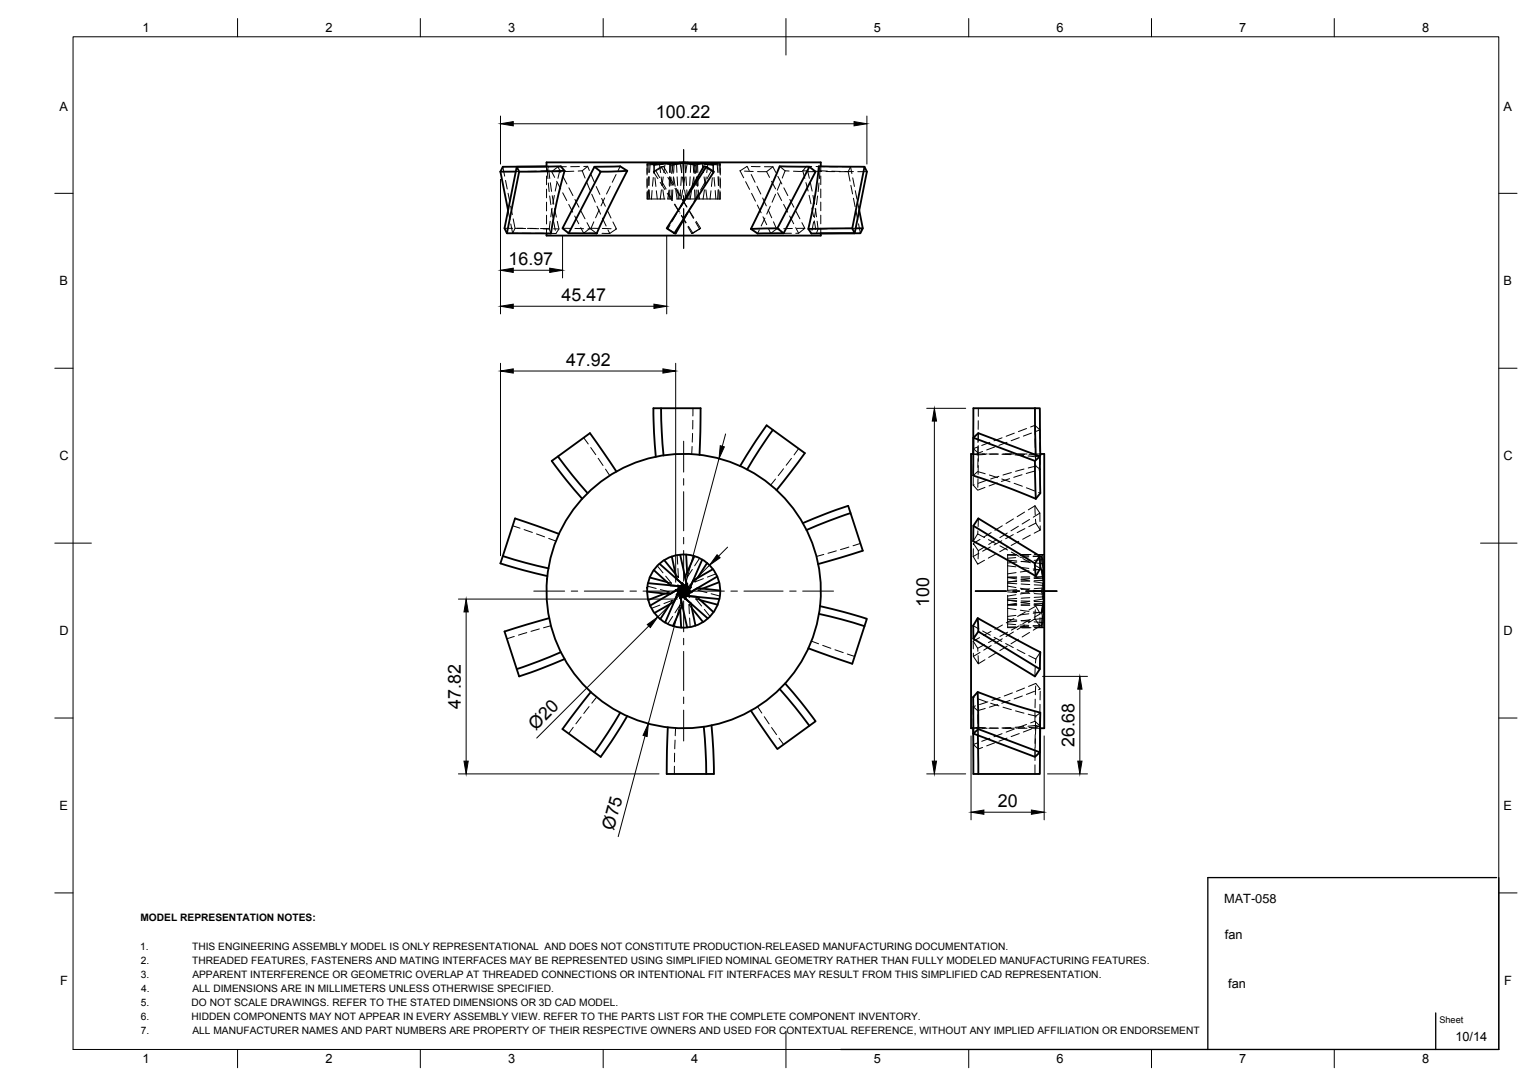
ISO-10303-21;
HEADER;
FILE_DESCRIPTION (('STEP AP214'),
    '1' );
FILE_NAME ('fan.step',
    '2026-10-21T17:54:40',
    ( '' ),
    ( '' ),
    'SwSTEP 2.0',
    'SolidWorks 2026',
    '' );
FILE_SCHEMA (( 'AUTOMOTIVE_DESIGN' ));
ENDSEC;

DATA;
#1=CARTESIAN_POINT ( 'NONE',  ( -0.3862712429686977478, 1.188820645368937390, -10.00000000000000000 ) ) ;
#18=CARTESIAN_POINT ( 'NONE',  ( -1.011271242968683426, -0.7347315653655928092, 3.333333333333333481 ) ) ;
#19=CARTESIAN_POINT ( 'NONE',  ( 42.78107912161490844, -16.56908454419397003, -9.367992836599951190 ) ) ;
#23=B_SPLINE_CURVE_WITH_KNOTS ( 'NONE', 3,
 ( #8249, #22875, #15684, #35464 ),
 .UNSPECIFIED., .F., .F.,
 ( 4, 4 ),
 ( 0.9895749839358303213, 1.000000000000000000 ),
 .UNSPECIFIED. ) ;
#32=CARTESIAN_POINT ( 'NONE',  ( -24.39427009666018265, -44.07992421011638129, 8.807470649214879543 ) ) ;
#37=CARTESIAN_POINT ( 'NONE',  ( 38.06347959788622859, -17.13191708601470964, -8.080361901872240793 ) ) ;
#38=FACE_OUTER_BOUND ( 'NONE', #34200, .T. ) ;
#42=EDGE_LOOP ( 'NONE', ( #31144, #13391, #8793, #47116, #38295 ) ) ;
#43=FACE_OUTER_BOUND ( 'NONE', #38714, .T. ) ;
#44=CARTESIAN_POINT ( 'NONE',  ( 45.64490844644691236, 21.32281559348795952, 8.807470649214879543 ) ) ;
#48=ORIENTED_EDGE ( 'NONE', *, *, #42434, .T. ) ;
#56=CARTESIAN_POINT ( 'NONE',  ( 47.23269937569327226, -16.43609759007049931, -2.408242355805840784 ) ) ;
#65=CARTESIAN_POINT ( 'NONE',  ( -0.3370904143228978245, 0.2449105217885259589, 10.00000000000000000 ) ) ;
#67=CARTESIAN_POINT ( 'NONE',  ( -12.78770032058971395, -31.68259716188267916, 7.455576670931136185 ) ) ;
#71=CARTESIAN_POINT ( 'NONE',  ( 10.30302290646030450, 13.08520913973580235, -9.683996418299976483 ) ) ;
#74=CARTESIAN_POINT ( 'NONE',  ( 50.11058929355269953, -7.578863168071589662, 7.455576670931136185 ) ) ;
#76=VERTEX_POINT ( 'NONE', #17762 ) ;
#84=CARTESIAN_POINT ( 'NONE',  ( -0.8965959638259611841, -1.582931917743307215, 9.903764339332084887 ) ) ;
#89=ORIENTED_EDGE ( 'NONE', *, *, #20681, .F. ) ;
#93=CARTESIAN_POINT ( 'NONE',  ( -32.43949840348904701, -7.871562655726274116, -9.367992836599954742 ) ) ;
#102=CARTESIAN_POINT ( 'NONE',  ( 1.011271242968688311, -0.7347315653655855927, 10.00000000000000000 ) ) ;
#108=ADVANCED_FACE ( 'NONE', ( #42862 ), #18238, .T. ) ;
#109=B_SPLINE_CURVE_WITH_KNOTS ( 'NONE', 3,
 ( #13337, #1308, #25156, #24903 ),
 .UNSPECIFIED., .F., .F.,
 ( 4, 4 ),
 ( 1.110764993427085326E-17, 0.002466147708923237519 ),
 .UNSPECIFIED. ) ;
#115=CARTESIAN_POINT ( 'NONE',  ( 24.39427009665985224, 44.07992421011656603, 8.807470649214879543 ) ) ;
#130=EDGE_CURVE ( 'NONE', #39856, #25517, #44158, .T. ) ;
#132=CIRCLE ( 'NONE', #9133, 37.50000000000000000 ) ;
#138=ADVANCED_FACE ( 'NONE', ( #43 ), #14562, .T. ) ;
#142=CARTESIAN_POINT ( 'NONE',  ( 1.088201875076330705, 0.7239277119154168272, 9.945465949847356768 ) ) ;
#146=ORIENTED_EDGE ( 'NONE', *, *, #12335, .F. ) ;
#148=CARTESIAN_POINT ( 'NONE',  ( 35.51846793572394034, -35.99772139009119343, 7.906207997025717304 ) ) ;
#149=CARTESIAN_POINT ( 'NONE',  ( -4.763548243873389154, 16.57409059453848599, 8.727788335465566760 ) ) ;
#154=CARTESIAN_POINT ( 'NONE',  ( 2.188678504086826848, -0.3267089737525829540, 9.881002359080282460 ) ) ;
#157=CARTESIAN_POINT ( 'NONE',  ( 1.249999999999999778, 0.000000000000000000, 3.333333333333333481 ) ) ;
#158=CARTESIAN_POINT ( 'NONE',  ( 1.228394325311184421, -1.341866297401743235, 9.903764339332088440 ) ) ;
#165=LINE ( 'NONE', #47317, #28159 ) ;
#170=CARTESIAN_POINT ( 'NONE',  ( -0.3862712429686977478, 1.188820645368937390, -3.333333333333333481 ) ) ;
#178=CARTESIAN_POINT ( 'NONE',  ( 26.18032376592674737, -21.95228666728361233, 7.455576670931136185 ) ) ;
#188=CARTESIAN_POINT ( 'NONE',  ( -49.46074318306826001, 9.578883844007169301, 8.807470649214879543 ) ) ;
#197=ORIENTED_EDGE ( 'NONE', *, *, #48845, .F. ) ;
#213=CARTESIAN_POINT ( 'NONE',  ( -0.4830800013901715428, -1.200413232422907761, 9.947020512645419643 ) ) ;
#219=CARTESIAN_POINT ( 'NONE',  ( 1.011271242968677653, 0.7347315653656002477, 10.00000000000000000 ) ) ;
#225=CARTESIAN_POINT ( 'NONE',  ( -1.365263087672800246, 0.5437404457009007430, 9.958264684458713489 ) ) ;
#227=CARTESIAN_POINT ( 'NONE',  ( -0.9983599181300891745, -1.124146016603549070, 9.953784399990620813 ) ) ;
#231=CARTESIAN_POINT ( 'NONE',  ( -44.99506233596264337, -23.32283626942287214, 7.455576670931136185 ) ) ;
#233=CARTESIAN_POINT ( 'NONE',  ( 0.4166666666666669072, 0.000000000000000000, 10.00000000000000000 ) ) ;
#238=CARTESIAN_POINT ( 'NONE',  ( -1.222012661920452326, 0.2471648704738776681, 9.981352469109934233 ) ) ;
#239=CARTESIAN_POINT ( 'NONE',  ( -1.249999999999999778, 0.000000000000000000, 9.972675548442463622 ) ) ;
#253=ORIENTED_EDGE ( 'NONE', *, *, #26936, .F. ) ;
#255=EDGE_CURVE ( 'NONE', #50289, #1639, #37383, .T. ) ;
#256=CARTESIAN_POINT ( 'NONE',  ( -14.52758583651993618, -8.922352469211071835, 8.953103998512858652 ) ) ;
#270=ORIENTED_EDGE ( 'NONE', *, *, #36402, .F. ) ;
#285=CARTESIAN_POINT ( 'NONE',  ( 37.27397286063867199, -4.111076158911552092, 7.697694107796188234 ) ) ;
#289=B_SPLINE_SURFACE_WITH_KNOTS ( 'NONE', 3, 3, ( 
 ( #36201, #41482, #14018, #25837 ),
 ( #10681, #49135, #24646, #8988 ),
 ( #37654, #47941, #16676, #34051 ),
 ( #45298, #29938, #45553, #6075 ) ),
 .UNSPECIFIED., .F., .F., .F.,
 ( 4, 4 ),
 ( 4, 4 ),
 ( 0.000000000000000000, 1.000000000000000000 ),
 ( 0.000000000000000000, 1.000000000000000000 ),
 .UNSPECIFIED. ) ;
#290=VERTEX_POINT ( 'NONE', #6397 ) ;
#298=CARTESIAN_POINT ( 'NONE',  ( 0.3862712429686727678, 1.188820645368945605, -3.333333333333333481 ) ) ;
#299=CARTESIAN_POINT ( 'NONE',  ( -0.1287570809895658697, 0.3962735484563123523, 10.00000000000000000 ) ) ;
#305=SHAPE_DEFINITION_REPRESENTATION ( #14247, #39915 ) ;
#308=CARTESIAN_POINT ( 'NONE',  ( -3.975459390375366997, -0.2195152216756601216, -2.642742795433417058E-16 ) ) ;
#312=CARTESIAN_POINT ( 'NONE',  ( -0.8433491450857070193, 0.9182416014173486740, 9.981352469109932457 ) ) ;
#323=VERTEX_POINT ( 'NONE', #49457 ) ;
#334=ORIENTED_EDGE ( 'NONE', *, *, #5259, .T. ) ;
#335=CARTESIAN_POINT ( 'NONE',  ( 7.937171537365877327, 0.3824377404836619698, 9.432811472610140413 ) ) ;
#339=VERTEX_POINT ( 'NONE', #33870 ) ;
#344=CARTESIAN_POINT ( 'NONE',  ( 36.97942854200454832, -6.226705766838405154, 8.914903342594563185 ) ) ;
#352=ORIENTED_EDGE ( 'NONE', *, *, #46014, .T. ) ;
#362=CARTESIAN_POINT ( 'NONE',  ( -29.18392875402943432, -17.44843138996582965, 7.906207997025717304 ) ) ;
#388=CARTESIAN_POINT ( 'NONE',  ( 8.277096487746778308, -33.14818118907697198, 7.455576670931136185 ) ) ;
#391=ORIENTED_EDGE ( 'NONE', *, *, #26509, .F. ) ;
#395=CARTESIAN_POINT ( 'NONE',  ( 23.82716369509147825, 44.49195112876006419, 8.356839323120299312 ) ) ;
#397=EDGE_LOOP ( 'NONE', ( #43742, #46810, #26881 ) ) ;
#400=CARTESIAN_POINT ( 'NONE',  ( -3.229232847726260403, 16.57333684275945629, 9.178419661560148768 ) ) ;
#408=EDGE_LOOP ( 'NONE', ( #49712, #23075, #15648, #3432 ) ) ;
#414=CARTESIAN_POINT ( 'NONE',  ( 6.174150299305392053, -50.00000000000000711, 8.807470649214879543 ) ) ;
#438=FACE_OUTER_BOUND ( 'NONE', #43936, .T. ) ;
#446=ORIENTED_EDGE ( 'NONE', *, *, #24923, .F. ) ;
#449=VERTEX_POINT ( 'NONE', #669 ) ;
#456=CARTESIAN_POINT ( 'NONE',  ( 33.08717642956892746, 5.870837526465160217, -8.016098858316199838 ) ) ;
#463=ORIENTED_EDGE ( 'NONE', *, *, #39701, .T. ) ;
#468=CARTESIAN_POINT ( 'NONE',  ( -9.998889670239194061, -0.1490146381531308739, 9.282506307616474217 ) ) ;
#478=CARTESIAN_POINT ( 'NONE',  ( -34.38425513258694366, 36.82177522737846687, 8.807470649214879543 ) ) ;
#483=CARTESIAN_POINT ( 'NONE',  ( -26.18032376592659105, 21.95228666728381128, 7.455576670931136185 ) ) ;
#487=CARTESIAN_POINT ( 'NONE',  ( -6.174150299305392053, 50.00000000000000711, 8.807470649214879543 ) ) ;
#490=CARTESIAN_POINT ( 'NONE',  ( 2.462075149652696027, -16.57295996686994499, 9.403735324607438884 ) ) ;
#494=CARTESIAN_POINT ( 'NONE',  ( 1.578643388466006714, -1.550786058692517511, 9.881002359080275355 ) ) ;
#496=CARTESIAN_POINT ( 'NONE',  ( 0.2773062244624638351, -1.251557370488896481, 9.948547179989619238 ) ) ;
#508=CARTESIAN_POINT ( 'NONE',  ( -49.46074318306826001, 9.578883844007169301, 8.807470649214879543 ) ) ;
#516=B_SPLINE_CURVE_WITH_KNOTS ( 'NONE', 3,
 ( #27272, #33769, #31384, #8032 ),
 .UNSPECIFIED., .F., .F.,
 ( 4, 4 ),
 ( 3.824349771687705441E-16, 0.009762429746916051129 ),
 .UNSPECIFIED. ) ;
#521=ORIENTED_EDGE ( 'NONE', *, *, #27225, .F. ) ;
#525=EDGE_CURVE ( 'NONE', #17682, #46476, #42731, .T. ) ;
#533=CARTESIAN_POINT ( 'NONE',  ( -1.280882217648866117, 0.5301415400469891015, 9.960033073700733652 ) ) ;
#542=CARTESIAN_POINT ( 'NONE',  ( -1.250000000000000222, 0.000000000000000000, -3.333333333333333481 ) ) ;
#549=CARTESIAN_POINT ( 'NONE',  ( -16.02661358026017524, -4.530191650547608972, -9.683996418299976483 ) ) ;
#565=CARTESIAN_POINT ( 'NONE',  ( -1.011271242968683426, -0.7347315653655928092, 3.333333333333333481 ) ) ;
#566=VERTEX_POINT ( 'NONE', #21168 ) ;
#603=ORIENTED_EDGE ( 'NONE', *, *, #32628, .T. ) ;
#616=ORIENTED_EDGE ( 'NONE', *, *, #17986, .F. ) ;
#617=CARTESIAN_POINT ( 'NONE',  ( 4.353119224256710496, 9.002796955358187247, 0.000000000000000000 ) ) ;
#634=CARTESIAN_POINT ( 'NONE',  ( -7.937171537365877327, -0.3824377404836087346, 9.432811472610140413 ) ) ;
#636=CARTESIAN_POINT ( 'NONE',  ( -0.6440276692615888310, -16.64212148744554298, -9.683996418299976483 ) ) ;
#642=FACE_OUTER_BOUND ( 'NONE', #16793, .T. ) ;
#648=CARTESIAN_POINT ( 'NONE',  ( 25.04522487443081502, -22.77512090857307925, 8.356839323120299312 ) ) ;
#655=CARTESIAN_POINT ( 'NONE',  ( -34.08355720199904226, 2.371364769369340042, 7.455576670931136185 ) ) ;
#656=ORIENTED_EDGE ( 'NONE', *, *, #48271, .F. ) ;
#657=CARTESIAN_POINT ( 'NONE',  ( -1.057156451998854996, 0.7920882637787067804, 9.943883492372851407 ) ) ;
#661=FACE_OUTER_BOUND ( 'NONE', #3377, .T. ) ;
#666=CARTESIAN_POINT ( 'NONE',  ( 34.08355720199905647, -2.371364769369109116, 7.455576670931136185 ) ) ;
#669=CARTESIAN_POINT ( 'NONE',  ( -20.21530556545279111, 31.58467066308232063, -9.422646554964174470 ) ) ;
#672=CARTESIAN_POINT ( 'NONE',  ( 20.40054609052976531, -26.26366202847973597, -3.760136334089591248 ) ) ;
#678=CARTESIAN_POINT ( 'NONE',  ( 0.9494396179258391966, -9.954826186926261755, 9.646707543097345905 ) ) ;
#686=CARTESIAN_POINT ( 'NONE',  ( 0.3896797354184660667, -1.262193838292004155, 9.943883492372872723 ) ) ;
#688=B_SPLINE_CURVE_WITH_KNOTS ( 'NONE', 3,
 ( #8937, #24844, #17140, #45060 ),
 .UNSPECIFIED., .F., .F.,
 ( 4, 4 ),
 ( 0.01010185847678695022, 0.01012833122191988955 ),
 .UNSPECIFIED. ) ;
#694=B_SPLINE_SURFACE_WITH_KNOTS ( 'NONE', 3, 3, ( 
 ( #30681, #46277, #15527, #50370 ),
 ( #15286, #30946, #46531, #27073 ),
 ( #42705, #38897, #23215, #7579 ),
 ( #3722, #19374, #35056, #28845 ) ),
 .UNSPECIFIED., .F., .F., .F.,
 ( 4, 4 ),
 ( 4, 4 ),
 ( 0.000000000000000000, 1.000000000000000000 ),
 ( 0.000000000000000000, 1.000000000000000000 ),
 .UNSPECIFIED. ) ;
#696=ORIENTED_EDGE ( 'NONE', *, *, #28856, .F. ) ;
#712=CARTESIAN_POINT ( 'NONE',  ( 34.95136153415558056, -36.40974830873469870, 8.356839323120299312 ) ) ;
#715=VERTEX_POINT ( 'NONE', #28612 ) ;
#733=CARTESIAN_POINT ( 'NONE',  ( -9.919534718723015843, 1.461167986671116470, 9.524510970296136136 ) ) ;
#736=CARTESIAN_POINT ( 'NONE',  ( 30.77287599203632951, 12.70002479445995824, 3.199614146704519602 ) ) ;
#744=CARTESIAN_POINT ( 'NONE',  ( 2.595273106918288164, 2.906811120256387326, 9.741991644047248045 ) ) ;
#745=EDGE_CURVE ( 'NONE', #4376, #24866, #38008, .T. ) ;
#747=CARTESIAN_POINT ( 'NONE',  ( 5.505322767148756569, -37.09368438467003415, 8.914903342594564961 ) ) ;
#756=CARTESIAN_POINT ( 'NONE',  ( -10.30302290646040397, -13.08520913973572597, -9.683996418299976483 ) ) ;
#763=ORIENTED_EDGE ( 'NONE', *, *, #20651, .T. ) ;
#764=ORIENTED_EDGE ( 'NONE', *, *, #23321, .T. ) ;
#776=CARTESIAN_POINT ( 'NONE',  ( -16.94310420131188266, 28.83076186680435171, -8.917361510505369182 ) ) ;
#783=CARTESIAN_POINT ( 'NONE',  ( -1.088201916217454546, -0.7239275277298468092, 9.945465957785078359 ) ) ;
#788=CARTESIAN_POINT ( 'NONE',  ( -34.38425513258695077, 36.82177522737848108, 8.807470649214879543 ) ) ;
#806=CARTESIAN_POINT ( 'NONE',  ( 0.1265591857323814795, 1.213367045380162823, 9.963925895596176474 ) ) ;
#818=CARTESIAN_POINT ( 'NONE',  ( 0.5107275442771160856, 1.175643901748075537, 9.976582533991678048 ) ) ;
#820=FACE_BOUND ( 'NONE', #42955, .T. ) ;
#823=ORIENTED_EDGE ( 'NONE', *, *, #37911, .F. ) ;
#842=PRODUCT_DEFINITION ( 'UNKNOWN', '', #50382, #12393 ) ;
#857=ORIENTED_EDGE ( 'NONE', *, *, #37508, .F. ) ;
#860=FACE_OUTER_BOUND ( 'NONE', #47872, .T. ) ;
#866=CARTESIAN_POINT ( 'NONE',  ( -46.10908423965022251, -19.89422939639105437, 1.847720168420772691 ) ) ;
#884=CARTESIAN_POINT ( 'NONE',  ( -9.645054515263723260, 2.693981805359463078, 6.429802539306485265 ) ) ;
#896=CARTESIAN_POINT ( 'NONE',  ( 4.672045878990125800, -50.00000000000000711, 1.847720168420772691 ) ) ;
#897=CARTESIAN_POINT ( 'NONE',  ( 3.239037401336969602, 33.28348308860766025, -8.917361510505369182 ) ) ;
#898=FACE_OUTER_BOUND ( 'NONE', #9786, .T. ) ;
#900=B_SPLINE_CURVE_WITH_KNOTS ( 'NONE', 3,
 ( #9085, #634, #24744, #13179 ),
 .UNSPECIFIED., .F., .F.,
 ( 4, 4 ),
 ( 0.8097120833243681703, 0.9322955464062560038 ),
 .UNSPECIFIED. ) ;
#904=CARTESIAN_POINT ( 'NONE',  ( 14.91630425054810161, -7.943683830272122215, -9.008049429158100807 ) ) ;
#914=ORIENTED_EDGE ( 'NONE', *, *, #10312, .F. ) ;
#927=CARTESIAN_POINT ( 'NONE',  ( 1.437255894074055185, -3.713052624461447682, -1.301042606982605321E-15 ) ) ;
#932=CARTESIAN_POINT ( 'NONE',  ( -1.862232582514199875, -0.9302239440314029606, 9.888808121373916293 ) ) ;
#937=LINE ( 'NONE', #39687, #19297 ) ;
#938=CARTESIAN_POINT ( 'NONE',  ( 17.23491422248386584, -0.5912720620000816441, 8.727788335465566760 ) ) ;
#949=CARTESIAN_POINT ( 'NONE',  ( 20.08067494016817633, 41.72051557472632055, 7.455576670931136185 ) ) ;
#952=CARTESIAN_POINT ( 'NONE',  ( -35.87018513526855656, -11.05844981164215746, -6.568693074176323421 ) ) ;
#955=DIRECTION ( 'NONE',  ( -0.2599384441937725998, 0.8000082703740912793, -0.5407575913134976542 ) ) ;
#961=CARTESIAN_POINT ( 'NONE',  ( -3.345242017215803276, 2.159124855890678596, -2.642742795433417058E-16 ) ) ;
#977=CARTESIAN_POINT ( 'NONE',  ( 4.030068433199813782, -6.879221474127158231, -6.505213034913026604E-16 ) ) ;
#989=CARTESIAN_POINT ( 'NONE',  ( 0.000000000000000000, 0.000000000000000000, 10.00000000000000000 ) ) ;
#993=CARTESIAN_POINT ( 'NONE',  ( 31.93002621080262671, 9.285431160462559674, -2.408242355805840784 ) ) ;
#999=EDGE_CURVE ( 'NONE', #12768, #45415, #1198, .T. ) ;
#1012=CARTESIAN_POINT ( 'NONE',  ( -0.9983599181300891745, -1.124146016603549070, 9.953784399990620813 ) ) ;
#1019=ORIENTED_EDGE ( 'NONE', *, *, #24264, .T. ) ;
#1036=CIRCLE ( 'NONE', #44408, 37.50000000000000000 ) ;
#1037=CARTESIAN_POINT ( 'NONE',  ( -34.91952936320829792, 13.67027684621028349, -9.422646554964178023 ) ) ;
#1039=VECTOR ( 'NONE', #9761, 1000.000000000000114 ) ;
#1041=CARTESIAN_POINT ( 'NONE',  ( -1.011271242968683426, -0.7347315653655928092, 10.00000000000000000 ) ) ;
#1048=CARTESIAN_POINT ( 'NONE',  ( -35.51846793572368455, 35.99772139009146343, 7.906207997025717304 ) ) ;
#1054=EDGE_CURVE ( 'NONE', #43553, #14725, #7925, .T. ) ;
#1058=VERTEX_POINT ( 'NONE', #40863 ) ;
#1069=VERTEX_POINT ( 'NONE', #12649 ) ;
#1070=CARTESIAN_POINT ( 'NONE',  ( 0.3370904143228924954, 0.2449105217885333141, 10.00000000000000000 ) ) ;
#1074=CARTESIAN_POINT ( 'NONE',  ( 18.67411147745603373, 27.51799019669827473, -3.760136334089591248 ) ) ;
#1087=ADVANCED_FACE ( 'NONE', ( #36286 ), #10893, .T. ) ;
#1089=CARTESIAN_POINT ( 'NONE',  ( 8.176860274785711979, -5.756644512789521606, 9.282506307616484875 ) ) ;
#1091=B_SPLINE_CURVE_WITH_KNOTS ( 'NONE', 3,
 ( #48534, #44212, #9084, #24739 ),
 .UNSPECIFIED., .F., .F.,
 ( 4, 4 ),
 ( 0.9688112071879400045, 0.9724175925769219520 ),
 .UNSPECIFIED. ) ;
#1097=DIRECTION ( 'NONE',  ( 0.000000000000000000, 0.000000000000000000, -1.000000000000000000 ) ) ;
#1100=CARTESIAN_POINT ( 'NONE',  ( -0.02998614097933045841, -1.600097392939481056, 9.919954280166498606 ) ) ;
#1104=CARTESIAN_POINT ( 'NONE',  ( -7.203307948779601233, 6.979912421814565171, 9.516222621873129839 ) ) ;
#1117=EDGE_CURVE ( 'NONE', #323, #20716, #47031, .T. ) ;
#1119=CARTESIAN_POINT ( 'NONE',  ( 0.3862712429686894766, -1.188820645368940276, -10.00000000000000000 ) ) ;
#1130=CARTESIAN_POINT ( 'NONE',  ( -27.73884755486766096, 25.23502201956265978, 7.697694107796191787 ) ) ;
#1131=ORIENTED_EDGE ( 'NONE', *, *, #31229, .T. ) ;
#1133=B_SPLINE_SURFACE_WITH_KNOTS ( 'NONE', 3, 3, ( 
 ( #2109, #17756, #29306, #17252 ),
 ( #33174, #21344, #17500, #24707 ),
 ( #40843, #16997, #1357, #9550 ),
 ( #40354, #36519, #21865, #49253 ) ),
 .UNSPECIFIED., .F., .F., .F.,
 ( 4, 4 ),
 ( 4, 4 ),
 ( 0.000000000000000000, 1.000000000000000000 ),
 ( 0.000000000000000000, 1.000000000000000000 ),
 .UNSPECIFIED. ) ;
#1134=CARTESIAN_POINT ( 'NONE',  ( -48.33712804702535237, -13.03701565032741705, -9.367992836599951190 ) ) ;
#1137=CARTESIAN_POINT ( 'NONE',  ( 49.46074318306830975, -9.578883844006833570, 8.807470649214879543 ) ) ;
#1144=ORIENTED_EDGE ( 'NONE', *, *, #37806, .T. ) ;
#1164=CARTESIAN_POINT ( 'NONE',  ( 44.99506233596247995, 23.32283626942318833, 7.455576670931136185 ) ) ;
#1172=CARTESIAN_POINT ( 'NONE',  ( -0.1287570809895602630, -0.3962735484563142396, 10.00000000000000000 ) ) ;
#1193=CARTESIAN_POINT ( 'NONE',  ( -0.3862712429686809279, -1.188820645368943163, 3.333333333333333481 ) ) ;
#1198=B_SPLINE_CURVE_WITH_KNOTS ( 'NONE', 3,
 ( #4713, #28057, #44689, #20352 ),
 .UNSPECIFIED., .F., .F.,
 ( 4, 4 ),
 ( 0.000000000000000000, 0.002368422649471283413 ),
 .UNSPECIFIED. ) ;
#1200=CARTESIAN_POINT ( 'NONE',  ( -0.8155877869437639927, -0.9072449372115535260, 9.963925895596188909 ) ) ;
#1201=CARTESIAN_POINT ( 'NONE',  ( -2.052549611693787135, 0.2039603569406744088, 9.894754715216729224 ) ) ;
#1209=CARTESIAN_POINT ( 'NONE',  ( 0.3370904143228924954, 0.2449105217885333141, 10.00000000000000000 ) ) ;
#1214=ORIENTED_EDGE ( 'NONE', *, *, #24898, .F. ) ;
#1215=CARTESIAN_POINT ( 'NONE',  ( 2.945500763482279627, 16.64098165802040086, -9.008049429158100807 ) ) ;
#1226=CARTESIAN_POINT ( 'NONE',  ( 3.798817505216071755, 5.709742178110386313, 9.753789706659947711 ) ) ;
#1229=CARTESIAN_POINT ( 'NONE',  ( -1.066995270233474624, 33.23888904628638841, -3.760136334089591248 ) ) ;
#1233=ORIENTED_EDGE ( 'NONE', *, *, #50556, .T. ) ;
#1235=CARTESIAN_POINT ( 'NONE',  ( 5.888214538810389698, 16.20866436362417673, 8.727788335465566760 ) ) ;
#1238=ORIENTED_EDGE ( 'NONE', *, *, #31217, .T. ) ;
#1248=CARTESIAN_POINT ( 'NONE',  ( 44.94002984196458073, 9.722063056714072005, -8.016098858316205167 ) ) ;
#1259=CARTESIAN_POINT ( 'NONE',  ( -0.6721397084974984892, -9.977385840602783773, 0.000000000000000000 ) ) ;
#1270=FACE_OUTER_BOUND ( 'NONE', #33337, .T. ) ;
#1274=ORIENTED_EDGE ( 'NONE', *, *, #16711, .T. ) ;
#1275=EDGE_LOOP ( 'NONE', ( #17040, #2179, #4711 ) ) ;
#1280=ORIENTED_EDGE ( 'NONE', *, *, #31121, .T. ) ;
#1285=CARTESIAN_POINT ( 'NONE',  ( -17.51065725283106644, 28.41934970907792390, -9.367992836599951190 ) ) ;
#1303=CARTESIAN_POINT ( 'NONE',  ( 7.359817328027030925, 15.16751262232805431, 2.590526750877053086 ) ) ;
#1306=CARTESIAN_POINT ( 'NONE',  ( 1.081517186030698241, -0.5722085955955613645, 9.993783931180535873 ) ) ;
#1308=CARTESIAN_POINT ( 'NONE',  ( 19.61585174098975770, -31.96834229807152283, -9.011255500499643745 ) ) ;
#1310=ORIENTED_EDGE ( 'NONE', *, *, #255, .T. ) ;
#1329=CARTESIAN_POINT ( 'NONE',  ( 13.59579750444771307, -10.60877755095900632, 8.727788335465566760 ) ) ;
#1334=EDGE_LOOP ( 'NONE', ( #25696, #12876, #33436 ) ) ;
#1354=EDGE_CURVE ( 'NONE', #16979, #715, #36101, .T. ) ;
#1356=CARTESIAN_POINT ( 'NONE',  ( 5.083187235775197266, 8.611690166631179366, 9.646707543097347681 ) ) ;
#1357=CARTESIAN_POINT ( 'NONE',  ( -15.98719783915689163, 4.501063718205989161, 3.266473740018926541 ) ) ;
#1362=B_SPLINE_CURVE_WITH_KNOTS ( 'NONE', 3,
 ( #23325, #18447, #23843, #46889 ),
 .UNSPECIFIED., .F., .F.,
 ( 4, 4 ),
 ( 0.000000000000000000, 0.2545280377015988749 ),
 .UNSPECIFIED. ) ;
#1367=DIRECTION ( 'NONE',  ( 0.000000000000000000, -1.000000000000000000, 0.000000000000000000 ) ) ;
#1374=CARTESIAN_POINT ( 'NONE',  ( 9.696760411815720460, 2.443938934556958653, 0.000000000000000000 ) ) ;
#1377=CARTESIAN_POINT ( 'NONE',  ( 5.325040722962521400, -2.676059336580344006, 7.623296525288703052E-16 ) ) ;
#1381=VERTEX_POINT ( 'NONE', #24160 ) ;
#1399=CARTESIAN_POINT ( 'NONE',  ( 30.21887974406487487, -14.69854701517530060, -8.016098858316205167 ) ) ;
#1407=CARTESIAN_POINT ( 'NONE',  ( -2.945500763482280959, -16.64098165802040086, -9.008049429158102583 ) ) ;
#1415=CARTESIAN_POINT ( 'NONE',  ( 14.76429217231961566, 8.192625680377691566, 9.178419661560148768 ) ) ;
#1425=CARTESIAN_POINT ( 'NONE',  ( -25.63461350838931807, 43.17876197216396861, -8.016098858316199838 ) ) ;
#1433=CARTESIAN_POINT ( 'NONE',  ( 0.1287570809895604018, 0.3962735484563146282, -10.00000000000000000 ) ) ;
#1440=VERTEX_POINT ( 'NONE', #28755 ) ;
#1441=CARTESIAN_POINT ( 'NONE',  ( 2.052549611693792464, -0.2039603569406628347, 9.894754715216725671 ) ) ;
#1443=B_SPLINE_SURFACE_WITH_KNOTS ( 'NONE', 3, 3, ( 
 ( #32886, #21064, #17467, #8779 ),
 ( #20307, #48222, #39832, #16469 ),
 ( #36750, #28769, #20807, #1070 ),
 ( #1824, #13357, #1329, #21315 ) ),
 .UNSPECIFIED., .F., .F., .F.,
 ( 4, 4 ),
 ( 4, 4 ),
 ( 0.000000000000000000, 1.000000000000000000 ),
 ( 0.000000000000000000, 1.000000000000000000 ),
 .UNSPECIFIED. ) ;
#1456=CARTESIAN_POINT ( 'NONE',  ( 20.20970188815904933, 31.63128376650817941, 3.209567239418972484 ) ) ;
#1461=CARTESIAN_POINT ( 'NONE',  ( 5.505322767148756569, -37.09368438467003415, 8.914903342594564961 ) ) ;
#1462=CARTESIAN_POINT ( 'NONE',  ( -3.893440188967678406, -0.6391102816410980658, 6.494306115488113207 ) ) ;
#1467=CARTESIAN_POINT ( 'NONE',  ( 4.641001526964560142, 33.28196331604080171, -8.016098858316199838 ) ) ;
#1477=ORIENTED_EDGE ( 'NONE', *, *, #34023, .T. ) ;
#1478=FACE_OUTER_BOUND ( 'NONE', #18244, .T. ) ;
#1483=ORIENTED_EDGE ( 'NONE', *, *, #9316, .F. ) ;
#1491=CARTESIAN_POINT ( 'NONE',  ( -0.1469336902871204442, -1.496274467947957376, 9.953784399990622589 ) ) ;
#1497=CARTESIAN_POINT ( 'NONE',  ( 22.69295089195473025, 45.31600496604705341, 7.455576670931136185 ) ) ;
#1504=CARTESIAN_POINT ( 'NONE',  ( -7.398363427652414614, 15.19415887381139108, -9.008049429158100807 ) ) ;
#1509=CARTESIAN_POINT ( 'NONE',  ( -15.42815683172655028, -34.17926237904570996, 7.697694107796190899 ) ) ;
#1510=CARTESIAN_POINT ( 'NONE',  ( -9.999999999999994671, -1.598124844265358068E-11, 9.303249460319950259 ) ) ;
#1513=ORIENTED_EDGE ( 'NONE', *, *, #38479, .T. ) ;
#1520=ORIENTED_EDGE ( 'NONE', *, *, #5204, .F. ) ;
#1524=VECTOR ( 'NONE', #37111, 1000.000000000000000 ) ;
#1530=CARTESIAN_POINT ( 'NONE',  ( -6.875132362119187768, 33.14667368551891258, 8.356839323120299312 ) ) ;
#1532=B_SPLINE_CURVE_WITH_KNOTS ( 'NONE', 3,
 ( #37436, #16713, #17656, #33324 ),
 .UNSPECIFIED., .F., .F.,
 ( 4, 4 ),
 ( 1.202632570208740988E-15, 0.0002520763768916307011 ),
 .UNSPECIFIED. ) ;
#1541=ORIENTED_EDGE ( 'NONE', *, *, #27872, .T. ) ;
#1543=CARTESIAN_POINT ( 'NONE',  ( -1.104609456715841986, -0.6504863887005195577, 9.948547179989617462 ) ) ;
#1562=CARTESIAN_POINT ( 'NONE',  ( 1.305887768059120768, -0.05395936524050352207, 9.945465957785110334 ) ) ;
#1564=ORIENTED_EDGE ( 'NONE', *, *, #42492, .F. ) ;
#1567=CARTESIAN_POINT ( 'NONE',  ( -31.28234235046239320, -11.28615439405757392, -3.760136334089591248 ) ) ;
#1587=CARTESIAN_POINT ( 'NONE',  ( -9.970345420962654970, 0.8985218257325405800, 2.778652340039163171 ) ) ;
#1599=ORIENTED_EDGE ( 'NONE', *, *, #39802, .T. ) ;
#1613=ORIENTED_EDGE ( 'NONE', *, *, #42830, .T. ) ;
#1624=CARTESIAN_POINT ( 'NONE',  ( 9.281355226777661116, -3.722424633806168615, 0.000000000000000000 ) ) ;
#1630=CARTESIAN_POINT ( 'NONE',  ( 1.250000000000000222, 0.000000000000000000, 10.00000000000000000 ) ) ;
#1639=VERTEX_POINT ( 'NONE', #35403 ) ;
#1648=CARTESIAN_POINT ( 'NONE',  ( 20.37409433807990666, 26.28007012093483397, -2.408242355805840784 ) ) ;
#1649=CARTESIAN_POINT ( 'NONE',  ( -16.15814872688569181, -4.048305257546697788, -2.870787844569587133 ) ) ;
#1654=CARTESIAN_POINT ( 'NONE',  ( -18.38319608353667434, 32.68498281710182596, -8.192531242611268638 ) ) ;
#1660=CARTESIAN_POINT ( 'NONE',  ( -1.552956552085981379, -0.2464513101957222507, 9.945241992664930919 ) ) ;
#1665=B_SPLINE_CURVE_WITH_KNOTS ( 'NONE', 3,
 ( #1927, #30132, #5767, #29372 ),
 .UNSPECIFIED., .F., .F.,
 ( 4, 4 ),
 ( 1.788112030672749005E-18, 0.009404691289023351872 ),
 .UNSPECIFIED. ) ;
#1673=AXIS2_PLACEMENT_3D ( 'NONE', #47188, #4871, #27484 ) ;
#1676=VERTEX_POINT ( 'NONE', #42057 ) ;
#1689=CARTESIAN_POINT ( 'NONE',  ( 20.21530556545302559, -31.58467066308217497, -9.422646554964174470 ) ) ;
#1696=CARTESIAN_POINT ( 'NONE',  ( 17.67745476136639482, 37.99701471135983155, 7.544061037322996377 ) ) ;
#1703=CARTESIAN_POINT ( 'NONE',  ( -15.44803555374685189, -6.237487519713257100, -3.546734833711462365 ) ) ;
#1705=CARTESIAN_POINT ( 'NONE',  ( 6.174150299305392053, -50.00000000000000000, 8.807470649214879543 ) ) ;
#1721=CARTESIAN_POINT ( 'NONE',  ( -0.6812154050773484570, -2.552002810692194590, 9.847478953136988622 ) ) ;
#1725=ORIENTED_EDGE ( 'NONE', *, *, #46852, .T. ) ;
#1729=ORIENTED_EDGE ( 'NONE', *, *, #43705, .F. ) ;
#1730=ORIENTED_EDGE ( 'NONE', *, *, #33079, .T. ) ;
#1732=CARTESIAN_POINT ( 'NONE',  ( 1.769963848780946369, -9.842115015280432644, 0.000000000000000000 ) ) ;
#1737=CIRCLE ( 'NONE', #6632, 10.00000000000000000 ) ;
#1746=CARTESIAN_POINT ( 'NONE',  ( 33.08717642956892746, 5.870837526465160217, -8.016098858316199838 ) ) ;
#1748=FACE_OUTER_BOUND ( 'NONE', #29837, .T. ) ;
#1762=CARTESIAN_POINT ( 'NONE',  ( -12.16428377685542195, -11.73151505502925929, -9.008049429158102583 ) ) ;
#1772=ORIENTED_EDGE ( 'NONE', *, *, #25237, .T. ) ;
#1774=CARTESIAN_POINT ( 'NONE',  ( -12.78770032058971395, -31.68259716188267916, 7.455576670931136185 ) ) ;
#1777=CARTESIAN_POINT ( 'NONE',  ( 44.99506233596247995, 23.32283626942318833, 7.455576670931136185 ) ) ;
#1790=VERTEX_POINT ( 'NONE', #17144 ) ;
#1794=ORIENTED_EDGE ( 'NONE', *, *, #9385, .F. ) ;
#1797=CARTESIAN_POINT ( 'NONE',  ( 1.250000000000000222, 0.000000000000000000, -3.333333333333333481 ) ) ;
#1802=CARTESIAN_POINT ( 'NONE',  ( 36.28567981536807707, 9.465698090293649614, -9.422646554964174470 ) ) ;
#1805=CARTESIAN_POINT ( 'NONE',  ( -46.10908423965022251, -19.89422939639105437, 1.847720168420772691 ) ) ;
#1807=B_SPLINE_CURVE_WITH_KNOTS ( 'NONE', 3,
 ( #29286, #12875, #24690, #17482 ),
 .UNSPECIFIED., .F., .F.,
 ( 4, 4 ),
 ( 3.469446951953614189E-18, 8.326314924666544353E-06 ),
 .UNSPECIFIED. ) ;
#1813=CARTESIAN_POINT ( 'NONE',  ( 0.4402108221923025089, -2.015156302359150331, 9.891980816076525684 ) ) ;
#1815=EDGE_LOOP ( 'NONE', ( #38601, #5434, #31334 ) ) ;
#1817=FACE_OUTER_BOUND ( 'NONE', #16806, .T. ) ;
#1822=CARTESIAN_POINT ( 'NONE',  ( 3.451199899302578977, -1.973209700276733480, 3.247138913692424467 ) ) ;
#1823=VERTEX_POINT ( 'NONE', #35663 ) ;
#1824=CARTESIAN_POINT ( 'NONE',  ( 36.08557433729230723, -35.58569447144768105, 7.455576670931136185 ) ) ;
#1836=CARTESIAN_POINT ( 'NONE',  ( -35.51846793572368455, 35.99772139009146343, 7.906207997025717304 ) ) ;
#1842=CARTESIAN_POINT ( 'NONE',  ( -0.2050626648094178439, 1.807624707194796843, 9.903764339332081335 ) ) ;
#1851=LINE ( 'NONE', #48748, #13088 ) ;
#1853=CARTESIAN_POINT ( 'NONE',  ( -3.087186397306470820, -2.514307945609864259, -2.642742795433417058E-16 ) ) ;
#1864=PLANE ( 'NONE',  #2561 ) ;
#1883=CARTESIAN_POINT ( 'NONE',  ( -0.7849184246622071814, 1.242376769534369041, 9.958264684458713489 ) ) ;
#1888=CARTESIAN_POINT ( 'NONE',  ( -7.303893058183219544, 3.196590768179758069, 3.455894424797545383E-16 ) ) ;
#1889=ADVANCED_FACE ( 'NONE', ( #2243 ), #41176, .T. ) ;
#1902=CARTESIAN_POINT ( 'NONE',  ( -2.538055338523173443, -33.28424297489108596, -9.367992836599951190 ) ) ;
#1912=VERTEX_POINT ( 'NONE', #14290 ) ;
#1927=CARTESIAN_POINT ( 'NONE',  ( -3.231548175622898089, 9.463461120997347820, 9.282506307616472441 ) ) ;
#1928=CARTESIAN_POINT ( 'NONE',  ( -30.21887974406478250, 14.69854701517551021, -8.016098858316205167 ) ) ;
#1952=CARTESIAN_POINT ( 'NONE',  ( -0.3862712429686895876, 1.188820645368940720, 3.333333333333333481 ) ) ;
#1953=CARTESIAN_POINT ( 'NONE',  ( -19.00512336303680883, 32.33518880947672614, -8.600750091277037157 ) ) ;
#1954=DIRECTION ( 'NONE',  ( -0.000000000000000000, -0.000000000000000000, -1.000000000000000000 ) ) ;
#1957=B_SPLINE_SURFACE_WITH_KNOTS ( 'NONE', 3, 3, ( 
 ( #18458, #14611, #14873, #42562 ),
 ( #11539, #7441, #34382, #49719 ),
 ( #30788, #19210, #26677, #41811 ),
 ( #30522, #23065, #38740, #50212 ) ),
 .UNSPECIFIED., .F., .F., .F.,
 ( 4, 4 ),
 ( 4, 4 ),
 ( 0.000000000000000000, 1.000000000000000000 ),
 ( 0.000000000000000000, 1.000000000000000000 ),
 .UNSPECIFIED. ) ;
#1959=CARTESIAN_POINT ( 'NONE',  ( -49.46074318306826001, 9.578883844007169301, 8.807470649214879543 ) ) ;
#1963=CARTESIAN_POINT ( 'NONE',  ( 6.174150299305392053, -50.00000000000000711, 8.807470649214879543 ) ) ;
#1979=EDGE_CURVE ( 'NONE', #16294, #12217, #29956, .T. ) ;
#1985=CARTESIAN_POINT ( 'NONE',  ( -0.2401930789658029419, -1.414287202658127685, 9.950105812514292936 ) ) ;
#1989=CARTESIAN_POINT ( 'NONE',  ( 36.62549812225761769, 8.082823558958848409, -8.600750091277037157 ) ) ;
#1991=ADVANCED_FACE ( 'NONE', ( #1748 ), #9635, .T. ) ;
#2034=ADVANCED_FACE ( 'NONE', ( #2995 ), #40768, .T. ) ;
#2056=CARTESIAN_POINT ( 'NONE',  ( -14.86945752723352498, -7.944783388878907004, 2.590526750877053086 ) ) ;
#2061=B_SPLINE_CURVE_WITH_KNOTS ( 'NONE', 3,
 ( #46805, #2973, #50648, #27619 ),
 .UNSPECIFIED., .F., .F.,
 ( 4, 4 ),
 ( 0.0008438930667322229028, 0.001027058643692256579 ),
 .UNSPECIFIED. ) ;
#2063=CARTESIAN_POINT ( 'NONE',  ( -45.42829307628559832, -21.98948915213271960, 8.356839323120299312 ) ) ;
#2067=CARTESIAN_POINT ( 'NONE',  ( 0.1475726264153646716, 1.496347932843221429, 9.927319414211224213 ) ) ;
#2069=CARTESIAN_POINT ( 'NONE',  ( -2.462075149652696027, 16.57295996686994499, 9.403735324607438884 ) ) ;
#2087=EDGE_CURVE ( 'NONE', #46411, #12768, #49540, .T. ) ;
#2091=CARTESIAN_POINT ( 'NONE',  ( 0.9001353430043829151, 1.054615064032355498, 9.960027343377989340 ) ) ;
#2109=CARTESIAN_POINT ( 'NONE',  ( -46.11867747200562917, 19.86470446310265103, -8.016098858316199838 ) ) ;
#2110=CARTESIAN_POINT ( 'NONE',  ( 9.760995290733820440, -2.173239732351728293, 9.646707543097347681 ) ) ;
#2111=CARTESIAN_POINT ( 'NONE',  ( -1.104609456715841986, -0.6504863887005195577, 9.948547179989617462 ) ) ;
#2116=B_SPLINE_CURVE_WITH_KNOTS ( 'NONE', 3,
 ( #28303, #36783, #31916, #32662 ),
 .UNSPECIFIED., .F., .F.,
 ( 4, 4 ),
 ( 3.127317220692750759E-18, 0.002458791966311098948 ),
 .UNSPECIFIED. ) ;
#2136=ADVANCED_FACE ( 'NONE', ( #39943 ), #33418, .T. ) ;
#2137=CARTESIAN_POINT ( 'NONE',  ( -0.7604583772867632430, 1.297021979207275466, 9.944962737436837230 ) ) ;
#2141=FACE_OUTER_BOUND ( 'NONE', #19435, .T. ) ;
#2144=CARTESIAN_POINT ( 'NONE',  ( 0.9358216137850741134, -0.9039474357314646324, 9.986087673579140400 ) ) ;
#2146=CARTESIAN_POINT ( 'NONE',  ( -0.3370904143228927730, -0.2449105217885335917, -10.00000000000000000 ) ) ;
#2151=CARTESIAN_POINT ( 'NONE',  ( 46.76852358249013975, -17.86468378716709182, -9.367992836599951190 ) ) ;
#2158=VERTEX_POINT ( 'NONE', #43184 ) ;
#2160=CARTESIAN_POINT ( 'NONE',  ( 48.33712804702526000, 13.03701565032775456, -9.367992836599954742 ) ) ;
#2179=ORIENTED_EDGE ( 'NONE', *, *, #7975, .F. ) ;
#2205=CARTESIAN_POINT ( 'NONE',  ( 24.19621561048219149, 28.69654500124514129, -5.338708898921616708 ) ) ;
#2206=CARTESIAN_POINT ( 'NONE',  ( -15.00099850811941948, -7.462898891544107016, 9.403735324607438884 ) ) ;
#2209=CARTESIAN_POINT ( 'NONE',  ( 30.25247992116058526, -39.82368563463805344, -3.760136334089591248 ) ) ;
#2217=CARTESIAN_POINT ( 'NONE',  ( -0.3370904143228943828, -0.2449105217885308716, 10.00000000000000000 ) ) ;
#2220=EDGE_LOOP ( 'NONE', ( #34116, #19277, #21719, #1477 ) ) ;
#2223=CARTESIAN_POINT ( 'NONE',  ( 37.27397286063867199, -4.111076158911552092, 7.697694107796188234 ) ) ;
#2229=ORIENTED_EDGE ( 'NONE', *, *, #21930, .T. ) ;
#2236=CARTESIAN_POINT ( 'NONE',  ( -35.35872492446279125, 12.59883863067526910, -2.490396854064192755 ) ) ;
#2238=CARTESIAN_POINT ( 'NONE',  ( -1.250000000000000222, 0.000000000000000000, 3.333333333333333481 ) ) ;
#2240=CARTESIAN_POINT ( 'NONE',  ( 10.69268279052430159, 12.77266927778462779, -2.870787844569587133 ) ) ;
#2243=FACE_OUTER_BOUND ( 'NONE', #8427, .T. ) ;
#2244=B_SPLINE_CURVE_WITH_KNOTS ( 'NONE', 3,
 ( #22400, #45715, #45467, #38331 ),
 .UNSPECIFIED., .F., .F.,
 ( 4, 4 ),
 ( 0.000000000000000000, 0.2562577668812812681 ),
 .UNSPECIFIED. ) ;
#2248=CARTESIAN_POINT ( 'NONE',  ( -29.61572577327014955, -16.11461842845715253, 8.807470649214879543 ) ) ;
#2250=ORIENTED_EDGE ( 'NONE', *, *, #6688, .F. ) ;
#2257=CARTESIAN_POINT ( 'NONE',  ( 8.176860274785711979, -5.756644512789521606, 9.282506307616484875 ) ) ;
#2261=B_SPLINE_SURFACE_WITH_KNOTS ( 'NONE', 3, 3, ( 
 ( #1959, #20698, #12985, #17603 ),
 ( #40712, #28647, #29164, #9653 ),
 ( #5549, #5297, #44277, #33020 ),
 ( #9404, #44780, #45025, #8898 ) ),
 .UNSPECIFIED., .F., .F., .F.,
 ( 4, 4 ),
 ( 4, 4 ),
 ( 0.000000000000000000, 1.000000000000000000 ),
 ( 0.000000000000000000, 1.000000000000000000 ),
 .UNSPECIFIED. ) ;
#2268=VERTEX_POINT ( 'NONE', #7796 ) ;
#2282=VERTEX_POINT ( 'NONE', #48738 ) ;
#2289=ADVANCED_FACE ( 'NONE', ( #25185 ), #28884, .T. ) ;
#2292=CARTESIAN_POINT ( 'NONE',  ( 22.69295089195473736, 45.31600496604706052, 7.455576670931136185 ) ) ;
#2302=CARTESIAN_POINT ( 'NONE',  ( 1.197382828408165567, -0.5140992728903442943, 9.961922210043278270 ) ) ;
#2303=CARTESIAN_POINT ( 'NONE',  ( -13.59579750444763668, 10.60877755095910935, 8.727788335465566760 ) ) ;
#2304=CARTESIAN_POINT ( 'NONE',  ( 0.3862712429686810944, 1.188820645368943607, -3.333333333333333481 ) ) ;
#2309=CARTESIAN_POINT ( 'NONE',  ( -7.576114424932982594, 50.00000000000000711, 7.906207997025717304 ) ) ;
#2316=ORIENTED_EDGE ( 'NONE', *, *, #9028, .T. ) ;
#2327=FACE_OUTER_BOUND ( 'NONE', #43838, .T. ) ;
#2332=CARTESIAN_POINT ( 'NONE',  ( -0.4430828623856294946, -1.527151971571945266, 9.933337059263825708 ) ) ;
#2336=CARTESIAN_POINT ( 'NONE',  ( -16.76006782980216059, 2.050259795448645228, 9.178419661560148768 ) ) ;
#2337=B_SPLINE_CURVE_WITH_KNOTS ( 'NONE', 3,
 ( #12521, #39239, #27679, #36149 ),
 .UNSPECIFIED., .F., .F.,
 ( 4, 4 ),
 ( 0.000000000000000000, 0.2562577668812813791 ),
 .UNSPECIFIED. ) ;
#2346=EDGE_CURVE ( 'NONE', #29795, #10907, #33649, .T. ) ;
#2359=CARTESIAN_POINT ( 'NONE',  ( -0.3862712429686729343, -1.188820645368946050, -10.00000000000000000 ) ) ;
#2375=B_SPLINE_SURFACE_WITH_KNOTS ( 'NONE', 3, 3, ( 
 ( #29137, #13476, #28881, #8871 ),
 ( #20929, #36614, #5526, #1193 ),
 ( #28620, #20414, #44256, #44501 ),
 ( #39939, #36349, #32236, #33000 ) ),
 .UNSPECIFIED., .F., .F., .F.,
 ( 4, 4 ),
 ( 4, 4 ),
 ( 0.000000000000000000, 1.000000000000000000 ),
 ( 0.000000000000000000, 1.000000000000000000 ),
 .UNSPECIFIED. ) ;
#2389=CARTESIAN_POINT ( 'NONE',  ( 13.92102703536701114, 30.85732372859822803, 8.356839323120299312 ) ) ;
#2395=EDGE_CURVE ( 'NONE', #44892, #32574, #23276, .T. ) ;
#2400=DIRECTION ( 'NONE',  ( -1.000000000000000000, 0.000000000000000000, 0.000000000000000000 ) ) ;
#2403=CARTESIAN_POINT ( 'NONE',  ( -0.2776613828612424784, 1.251395203515897503, 9.967237415621765351 ) ) ;
#2418=EDGE_CURVE ( 'NONE', #38616, #43903, #6155, .T. ) ;
#2421=B_SPLINE_CURVE_WITH_KNOTS ( 'NONE', 3,
 ( #9540, #32647, #37520, #21337 ),
 .UNSPECIFIED., .F., .F.,
 ( 4, 4 ),
 ( 5.641302087951259315E-05, 0.0003272669002642556607 ),
 .UNSPECIFIED. ) ;
#2423=VERTEX_POINT ( 'NONE', #45407 ) ;
#2431=CARTESIAN_POINT ( 'NONE',  ( -0.9598058911017687267, -1.847159827636240426, 9.888808121373918070 ) ) ;
#2437=DIRECTION ( 'NONE',  ( -1.000000000000000000, 0.000000000000000000, 0.000000000000000000 ) ) ;
#2439=CARTESIAN_POINT ( 'NONE',  ( 0.4548599190037341811, 1.225298710497799703, 9.945465957785110334 ) ) ;
#2451=FACE_OUTER_BOUND ( 'NONE', #397, .T. ) ;
#2458=CARTESIAN_POINT ( 'NONE',  ( 1.780557400379557231, 1.041314823045442095, 9.889206917020299414 ) ) ;
#2461=CARTESIAN_POINT ( 'NONE',  ( -25.61277432017861955, 22.36370378792854297, 7.906207997025717304 ) ) ;
#2464=ORIENTED_EDGE ( 'NONE', *, *, #7471, .F. ) ;
#2473=EDGE_CURVE ( 'NONE', #449, #46833, #29413, .T. ) ;
#2490=CARTESIAN_POINT ( 'NONE',  ( -1.250000000000000222, 0.000000000000000000, -10.00000000000000000 ) ) ;
#2495=CARTESIAN_POINT ( 'NONE',  ( 1.172603113866929725, 0.3455467477709275870, 9.987567862361069970 ) ) ;
#2497=CARTESIAN_POINT ( 'NONE',  ( 50.11058929355270664, -7.578863168071591438, 7.455576670931136185 ) ) ;
#2528=FACE_OUTER_BOUND ( 'NONE', #1334, .T. ) ;
#2533=CARTESIAN_POINT ( 'NONE',  ( -8.813458710706198573, -4.724716452304520864, 0.000000000000000000 ) ) ;
#2550=B_SPLINE_CURVE_WITH_KNOTS ( 'NONE', 3,
 ( #46621, #11008, #50466, #15374 ),
 .UNSPECIFIED., .F., .F.,
 ( 4, 4 ),
 ( 1.760159736610854221E-18, 0.0009539133080775338879 ),
 .UNSPECIFIED. ) ;
#2554=CARTESIAN_POINT ( 'NONE',  ( -1.011271242968683426, -0.7347315653655928092, -10.00000000000000000 ) ) ;
#2555=CARTESIAN_POINT ( 'NONE',  ( -0.2773062244624664441, 1.251557370488897813, 9.948547179989621014 ) ) ;
#2561=AXIS2_PLACEMENT_3D ( 'NONE', #36529, #1367, #20344 ) ;
#2562=ORIENTED_EDGE ( 'NONE', *, *, #16697, .T. ) ;
#2565=CARTESIAN_POINT ( 'NONE',  ( 1.250000000000000222, 0.000000000000000000, 10.00000000000000000 ) ) ;
#2567=CARTESIAN_POINT ( 'NONE',  ( 1.258633725701695294, -0.04081300982073039069, 9.974012008644017158 ) ) ;
#2572=CARTESIAN_POINT ( 'NONE',  ( -18.38319608353667434, 32.68498281710182596, -8.192531242611268638 ) ) ;
#2576=CARTESIAN_POINT ( 'NONE',  ( -34.95136153415531766, 36.40974830873496870, 8.356839323120299312 ) ) ;
#2589=ORIENTED_EDGE ( 'NONE', *, *, #525, .T. ) ;
#2592=CARTESIAN_POINT ( 'NONE',  ( -4.997592503980432532, -3.246827225423192687, 1.992221491942114397E-15 ) ) ;
#2594=EDGE_CURVE ( 'NONE', #30805, #19380, #4112, .T. ) ;
#2598=CARTESIAN_POINT ( 'NONE',  ( 15.45175104485250728, -6.222373774239001065, -2.870787844569587133 ) ) ;
#2599=ADVANCED_FACE ( 'NONE', ( #8478 ), #16173, .F. ) ;
#2613=FACE_OUTER_BOUND ( 'NONE', #2220, .T. ) ;
#2618=CARTESIAN_POINT ( 'NONE',  ( 49.67735855322978011, -8.912210285361751971, 8.356839323120299312 ) ) ;
#2635=ORIENTED_EDGE ( 'NONE', *, *, #20465, .F. ) ;
#2644=CARTESIAN_POINT ( 'NONE',  ( -3.087186397306470820, -2.514307945609864259, -2.642742795433417058E-16 ) ) ;
#2646=EDGE_LOOP ( 'NONE', ( #14887, #27881, #28355, #15359 ) ) ;
#2653=EDGE_LOOP ( 'NONE', ( #13262, #17292, #31530 ) ) ;
#2658=EDGE_CURVE ( 'NONE', #50662, #36948, #19601, .T. ) ;
#2672=CARTESIAN_POINT ( 'NONE',  ( -2.538055338523173443, -50.00000000000000000, -9.367992836599951190 ) ) ;
#2682=B_SPLINE_SURFACE_WITH_KNOTS ( 'NONE', 3, 3, ( 
 ( #24200, #27786, #15726, #11369 ),
 ( #11888, #27546, #7794, #8294 ),
 ( #23933, #39862, #39597, #35768 ),
 ( #42660, #7534, #23169, #19320 ) ),
 .UNSPECIFIED., .F., .F., .F.,
 ( 4, 4 ),
 ( 4, 4 ),
 ( 0.000000000000000000, 1.000000000000000000 ),
 ( 0.000000000000000000, 1.000000000000000000 ),
 .UNSPECIFIED. ) ;
#2684=CARTESIAN_POINT ( 'NONE',  ( -46.11867747200562917, 19.86470446310265103, -8.016098858316199838 ) ) ;
#2694=CARTESIAN_POINT ( 'NONE',  ( -45.64490844644706868, -21.32281559348764333, 8.807470649214879543 ) ) ;
#2695=CARTESIAN_POINT ( 'NONE',  ( -14.48769039275601145, -30.44468701195584970, 8.807470649214879543 ) ) ;
#2700=EDGE_LOOP ( 'NONE', ( #11883, #13664, #45812 ) ) ;
#2701=VERTEX_POINT ( 'NONE', #21776 ) ;
#2702=CARTESIAN_POINT ( 'NONE',  ( -0.6595498452743703277, 16.59563386392009576, 3.266473740018926541 ) ) ;
#2709=CARTESIAN_POINT ( 'NONE',  ( 8.277096487746778308, -50.00000000000000711, 7.455576670931136185 ) ) ;
#2718=CARTESIAN_POINT ( 'NONE',  ( -42.78107912161479476, 16.56908454419426135, -9.367992836599951190 ) ) ;
#2734=CARTESIAN_POINT ( 'NONE',  ( -1.250000000000000222, 0.000000000000000000, -3.333333333333333481 ) ) ;
#2743=ORIENTED_EDGE ( 'NONE', *, *, #40149, .T. ) ;
#2758=CARTESIAN_POINT ( 'NONE',  ( -24.39427009666018265, -44.07992421011638129, 8.807470649214879543 ) ) ;
#2760=ORIENTED_EDGE ( 'NONE', *, *, #21930, .F. ) ;
#2767=CARTESIAN_POINT ( 'NONE',  ( -46.76852358249002606, 17.86468378716741512, -9.367992836599954742 ) ) ;
#2773=ORIENTED_EDGE ( 'NONE', *, *, #2346, .F. ) ;
#2784=DIRECTION ( 'NONE',  ( -1.000000000000000000, 0.000000000000000000, 0.000000000000000000 ) ) ;
#2785=B_SPLINE_CURVE_WITH_KNOTS ( 'NONE', 3,
 ( #3000, #15827, #4285, #31492 ),
 .UNSPECIFIED., .F., .F.,
 ( 4, 4 ),
 ( 1.592264493058081649E-17, 0.009404495247862340590 ),
 .UNSPECIFIED. ) ;
#2788=B_SPLINE_SURFACE_WITH_KNOTS ( 'NONE', 3, 3, ( 
 ( #31024, #483, #31787, #47372 ),
 ( #3811, #19715, #35394, #31535 ),
 ( #9426, #35893, #33043, #32548 ),
 ( #12773, #16886, #17130, #48631 ) ),
 .UNSPECIFIED., .F., .F., .F.,
 ( 4, 4 ),
 ( 4, 4 ),
 ( 0.000000000000000000, 1.000000000000000000 ),
 ( 0.000000000000000000, 1.000000000000000000 ),
 .UNSPECIFIED. ) ;
#2795=ORIENTED_EDGE ( 'NONE', *, *, #50287, .F. ) ;
#2796=CARTESIAN_POINT ( 'NONE',  ( -0.6369768774138663270, 1.285364331396255944, 9.950105812514292936 ) ) ;
#2797=ADVANCED_FACE ( 'NONE', ( #42970 ), #38212, .F. ) ;
#2802=CARTESIAN_POINT ( 'NONE',  ( 8.001683061421385190, 5.997755262142701937, 9.282506307616484875 ) ) ;
#2806=CARTESIAN_POINT ( 'NONE',  ( 23.26005729352310425, 44.90397804740356236, 7.906207997025717304 ) ) ;
#2822=ORIENTED_EDGE ( 'NONE', *, *, #6477, .T. ) ;
#2840=FACE_BOUND ( 'NONE', #31497, .T. ) ;
#2841=CARTESIAN_POINT ( 'NONE',  ( 12.35406723005396046, -11.51001571518080624, 9.178419661560148768 ) ) ;
#2860=CARTESIAN_POINT ( 'NONE',  ( -1.724908962443186367, 9.880865948510580310, 9.516222621873128062 ) ) ;
#2861=CARTESIAN_POINT ( 'NONE',  ( -4.207128120815918256E-14, 3.058192377181588826E-14, 10.00000000000000000 ) ) ;
#2870=CARTESIAN_POINT ( 'NONE',  ( 1.365263087672787590, -0.5437404457008400138, 9.958264684458717042 ) ) ;
#2871=CARTESIAN_POINT ( 'NONE',  ( 16.94310420131209227, -28.83076186680421671, -8.917361510505369182 ) ) ;
#2875=CARTESIAN_POINT ( 'NONE',  ( 46.10908423965007330, 19.89422939639137766, 1.847720168420772691 ) ) ;
#2879=ORIENTED_EDGE ( 'NONE', *, *, #12373, .T. ) ;
#2890=CARTESIAN_POINT ( 'NONE',  ( -1.337801958641930300, -1.088266084286974689, 9.928159647716134018 ) ) ;
#2891=ORIENTED_EDGE ( 'NONE', *, *, #43824, .T. ) ;
#2906=CARTESIAN_POINT ( 'NONE',  ( -0.9923808968704912470, 0.8303844723052444809, 9.947020512645417867 ) ) ;
#2914=FACE_OUTER_BOUND ( 'NONE', #47406, .T. ) ;
#2929=CARTESIAN_POINT ( 'NONE',  ( 0.3862712429686810944, 1.188820645368943607, 10.00000000000000000 ) ) ;
#2935=CARTESIAN_POINT ( 'NONE',  ( 45.64490844644691236, 21.32281559348795952, 8.807470649214879543 ) ) ;
#2943=CARTESIAN_POINT ( 'NONE',  ( -23.82716369509181575, -44.49195112875988656, 8.356839323120299312 ) ) ;
#2944=CARTESIAN_POINT ( 'NONE',  ( 9.260964247899973856, -13.84230907185609460, -9.683996418299976483 ) ) ;
#2952=CARTESIAN_POINT ( 'NONE',  ( -4.672045878990125800, 50.00000000000000711, 1.847720168420772691 ) ) ;
#2954=CARTESIAN_POINT ( 'NONE',  ( -36.08557433729205144, 35.58569447144795816, 7.455576670931136185 ) ) ;
#2962=CARTESIAN_POINT ( 'NONE',  ( -1.011271242968693862, 0.7347315653655780432, -3.333333333333333481 ) ) ;
#2963=ORIENTED_EDGE ( 'NONE', *, *, #24972, .T. ) ;
#2964=CARTESIAN_POINT ( 'NONE',  ( -38.83486119589580454, 15.16159403945161621, -9.387872844313825738 ) ) ;
#2973=CARTESIAN_POINT ( 'NONE',  ( 1.841313484560079816, 1.034875822465065820, 9.884520277910693764 ) ) ;
#2975=ORIENTED_EDGE ( 'NONE', *, *, #2473, .F. ) ;
#2989=CARTESIAN_POINT ( 'NONE',  ( 9.221081804193270059, 13.81382350053991104, 3.266473740018926541 ) ) ;
#2995=FACE_OUTER_BOUND ( 'NONE', #40559, .T. ) ;
#2998=CARTESIAN_POINT ( 'NONE',  ( 3.996390545799824334, -16.57371371864897469, 8.953103998512858652 ) ) ;
#3000=CARTESIAN_POINT ( 'NONE',  ( 8.001683061421385190, 5.997755262142701937, 9.282506307616484875 ) ) ;
#3011=CARTESIAN_POINT ( 'NONE',  ( -9.221081804193374865, -13.81382350053984176, 3.266473740018926541 ) ) ;
#3029=ORIENTED_EDGE ( 'NONE', *, *, #18887, .F. ) ;
#3032=ORIENTED_EDGE ( 'NONE', *, *, #46572, .T. ) ;
#3050=CARTESIAN_POINT ( 'NONE',  ( -0.5133303889063141057, 1.273801409042568888, 9.946805383069623474 ) ) ;
#3055=CARTESIAN_POINT ( 'NONE',  ( 25.63461350838963426, -43.17876197216376966, -8.016098858316199838 ) ) ;
#3060=CARTESIAN_POINT ( 'NONE',  ( -24.87968592351613495, -28.06706927586046518, -8.600750091277037157 ) ) ;
#3062=CARTESIAN_POINT ( 'NONE',  ( 34.08355720199905647, -2.371364769369109116, 7.455576670931136185 ) ) ;
#3069=CARTESIAN_POINT ( 'NONE',  ( 1.267276237729528354, -0.08162529406826456169, 9.975314328424614629 ) ) ;
#3075=CARTESIAN_POINT ( 'NONE',  ( 0.3862712429686978033, -1.188820645368937834, 10.00000000000000000 ) ) ;
#3088=EDGE_CURVE ( 'NONE', #26328, #3380, #34892, .T. ) ;
#3089=CARTESIAN_POINT ( 'NONE',  ( -0.7601424845489993531, 1.297311920617006065, 9.927319414211224213 ) ) ;
#3091=FACE_OUTER_BOUND ( 'NONE', #10508, .T. ) ;
#3097=B_SPLINE_SURFACE_WITH_KNOTS ( 'NONE', 3, 3, ( 
 ( #32175, #8823, #8072, #39378 ),
 ( #23961, #47013, #24476, #4214 ),
 ( #35528, #40125, #16018, #4956 ),
 ( #20613, #36292, #16768, #10337 ) ),
 .UNSPECIFIED., .F., .F., .F.,
 ( 4, 4 ),
 ( 4, 4 ),
 ( 0.000000000000000000, 1.000000000000000000 ),
 ( 0.000000000000000000, 1.000000000000000000 ),
 .UNSPECIFIED. ) ;
#3098=ORIENTED_EDGE ( 'NONE', *, *, #1117, .T. ) ;
#3100=CARTESIAN_POINT ( 'NONE',  ( 13.59579750444771307, -10.60877755095900632, 8.727788335465566760 ) ) ;
#3105=CARTESIAN_POINT ( 'NONE',  ( 1.011271242968688311, -0.7347315653655855927, 10.00000000000000000 ) ) ;
#3107=CARTESIAN_POINT ( 'NONE',  ( 33.16902712922644270, -37.70469005304286725, 1.847720168420772691 ) ) ;
#3113=CARTESIAN_POINT ( 'NONE',  ( -2.595273106918313033, -2.906811120256372671, 9.741991644047246268 ) ) ;
#3133=ORIENTED_EDGE ( 'NONE', *, *, #29928, .F. ) ;
#3134=CARTESIAN_POINT ( 'NONE',  ( 32.43949840348898306, 7.871562655726499713, -9.367992836599954742 ) ) ;
#3137=VERTEX_POINT ( 'NONE', #17806 ) ;
#3140=CARTESIAN_POINT ( 'NONE',  ( 16.07893968642772364, 33.88550589494195009, 8.100132398494510610 ) ) ;
#3144=B_SPLINE_CURVE_WITH_KNOTS ( 'NONE', 3,
 ( #41947, #21682, #49592, #49093 ),
 .UNSPECIFIED., .F., .F.,
 ( 4, 4 ),
 ( 0.000000000000000000, 0.001246897409371962393 ),
 .UNSPECIFIED. ) ;
#3152=CARTESIAN_POINT ( 'NONE',  ( 0.3862712429686894766, -1.188820645368940276, 3.333333333333333481 ) ) ;
#3177=B_SPLINE_CURVE_WITH_KNOTS ( 'NONE', 3,
 ( #11859, #19027, #3644, #20057 ),
 .UNSPECIFIED., .F., .F.,
 ( 4, 4 ),
 ( 0.000000000000000000, 0.0009539133080771172290 ),
 .UNSPECIFIED. ) ;
#3189=CARTESIAN_POINT ( 'NONE',  ( 9.260964247899973856, -13.84230907185609460, -9.683996418299976483 ) ) ;
#3190=CARTESIAN_POINT ( 'NONE',  ( -7.749480817862350435, -14.85497772329513211, 9.403735324607438884 ) ) ;
#3193=B_SPLINE_SURFACE_WITH_KNOTS ( 'NONE', 3, 3, ( 
 ( #23239, #15316, #10939, #19654 ),
 ( #15046, #18874, #11210, #50653 ),
 ( #46049, #38414, #11967, #170 ),
 ( #50403, #31219, #39430, #26599 ) ),
 .UNSPECIFIED., .F., .F., .F.,
 ( 4, 4 ),
 ( 4, 4 ),
 ( 0.000000000000000000, 1.000000000000000000 ),
 ( 0.000000000000000000, 1.000000000000000000 ),
 .UNSPECIFIED. ) ;
#3197=CARTESIAN_POINT ( 'NONE',  ( -1.249999999999999778, 0.000000000000000000, -3.333333333333333481 ) ) ;
#3199=ORIENTED_EDGE ( 'NONE', *, *, #8595, .F. ) ;
#3207=CARTESIAN_POINT ( 'NONE',  ( 0.3862712429686810944, 1.188820645368943607, 10.00000000000000000 ) ) ;
#3213=DIRECTION ( 'NONE',  ( -0.000000000000000000, -0.000000000000000000, -1.000000000000000000 ) ) ;
#3238=CARTESIAN_POINT ( 'NONE',  ( -3.245326723439060146, -7.282604692634697230, 0.000000000000000000 ) ) ;
#3240=CARTESIAN_POINT ( 'NONE',  ( 46.76852358249013975, -17.86468378716709537, -9.367992836599954742 ) ) ;
#3244=CARTESIAN_POINT ( 'NONE',  ( 36.08557433729230723, -35.58569447144768105, 7.455576670931136185 ) ) ;
#3254=CARTESIAN_POINT ( 'NONE',  ( 3.940019464150765760, 33.28272320232423453, -8.466730184410787174 ) ) ;
#3259=CARTESIAN_POINT ( 'NONE',  ( -12.16428377685542017, -11.73151505502925929, -9.008049429158100807 ) ) ;
#3271=CARTESIAN_POINT ( 'NONE',  ( 0.1469336902871260508, 1.496274467947966258, 9.953784399990622589 ) ) ;
#3285=CARTESIAN_POINT ( 'NONE',  ( 27.31081730472575941, 41.96092862852144378, 3.199614146704519602 ) ) ;
#3286=CARTESIAN_POINT ( 'NONE',  ( 7.359817328027030925, 15.16751262232805431, 2.590526750877053086 ) ) ;
#3291=CARTESIAN_POINT ( 'NONE',  ( 0.6440276692615888310, 16.64212148744554298, -9.683996418299976483 ) ) ;
#3302=AXIS2_PLACEMENT_3D ( 'NONE', #7934, #8178, #8688 ) ;
#3307=CARTESIAN_POINT ( 'NONE',  ( -0.7964335060761117413, -1.145363263855212477, 9.955131761384825140 ) ) ;
#3309=CARTESIAN_POINT ( 'NONE',  ( -1.962558162477761714, 3.366505435501197407, 9.741991644046970933 ) ) ;
#3314=CARTESIAN_POINT ( 'NONE',  ( -14.76429217231967428, -8.192625680377590314, 9.178419661560148768 ) ) ;
#3316=ORIENTED_EDGE ( 'NONE', *, *, #27779, .T. ) ;
#3332=ORIENTED_EDGE ( 'NONE', *, *, #37837, .T. ) ;
#3333=CARTESIAN_POINT ( 'NONE',  ( -33.16902712922616558, 37.70469005304312304, 1.847720168420772691 ) ) ;
#3338=B_SPLINE_CURVE_WITH_KNOTS ( 'NONE', 3,
 ( #32918, #38538, #25970, #38291 ),
 .UNSPECIFIED., .F., .F.,
 ( 4, 4 ),
 ( 0.9890644561682322422, 1.000000000000000000 ),
 .UNSPECIFIED. ) ;
#3346=CARTESIAN_POINT ( 'NONE',  ( -0.9870575514055066613, -1.980598328282574316, 9.881002359080278907 ) ) ;
#3350=ADVANCED_FACE ( 'NONE', ( #36259 ), #8291, .F. ) ;
#3353=CARTESIAN_POINT ( 'NONE',  ( -2.188678504086925880, 0.3267089737526900350, 9.881002359080270026 ) ) ;
#3356=CARTESIAN_POINT ( 'NONE',  ( 0.7964335060745958428, 1.145363263855377456, 9.955131761384901523 ) ) ;
#3359=CARTESIAN_POINT ( 'NONE',  ( 0.1469336902871260508, 1.496274467947966258, 9.953784399990622589 ) ) ;
#3360=FACE_OUTER_BOUND ( 'NONE', #30031, .T. ) ;
#3369=CARTESIAN_POINT ( 'NONE',  ( -1.011271242968693862, 0.7347315653655780432, 10.00000000000000000 ) ) ;
#3370=ORIENTED_EDGE ( 'NONE', *, *, #26185, .F. ) ;
#3373=CARTESIAN_POINT ( 'NONE',  ( -15.62858259096117841, 5.755205073598721910, -9.683996418299976483 ) ) ;
#3375=CARTESIAN_POINT ( 'NONE',  ( 0.8965959638259385356, 1.582931917743541028, 9.903764339332076005 ) ) ;
#3377=EDGE_LOOP ( 'NONE', ( #17966, #12196, #20456 ) ) ;
#3379=CARTESIAN_POINT ( 'NONE',  ( -0.4611230188129920582, 1.144552435864505835, 9.969907203203804968 ) ) ;
#3380=VERTEX_POINT ( 'NONE', #31900 ) ;
#3402=VERTEX_POINT ( 'NONE', #37281 ) ;
#3416=ORIENTED_EDGE ( 'NONE', *, *, #42506, .T. ) ;
#3421=CARTESIAN_POINT ( 'NONE',  ( 0.3862712429686894766, -1.188820645368940276, 10.00000000000000000 ) ) ;
#3432=ORIENTED_EDGE ( 'NONE', *, *, #40983, .T. ) ;
#3457=CARTESIAN_POINT ( 'NONE',  ( 45.42829307628542779, 21.98948915213303579, 8.356839323120299312 ) ) ;
#3470=CARTESIAN_POINT ( 'NONE',  ( 5.542614707656925432, 8.340505786370636443, 6.429802539306464837 ) ) ;
#3473=ORIENTED_EDGE ( 'NONE', *, *, #15794, .T. ) ;
#3484=EDGE_LOOP ( 'NONE', ( #30437, #29593, #4566 ) ) ;
#3491=CARTESIAN_POINT ( 'NONE',  ( 47.88254548617766204, -14.43607691413525984, -3.760136334089591248 ) ) ;
#3494=CARTESIAN_POINT ( 'NONE',  ( 1.011271242968677653, 0.7347315653656002477, -10.00000000000000000 ) ) ;
#3497=CARTESIAN_POINT ( 'NONE',  ( 1.655785408456140084, 0.7536129375913136474, 9.903764339332061795 ) ) ;
#3508=ORIENTED_EDGE ( 'NONE', *, *, #43790, .F. ) ;
#3510=B_SPLINE_SURFACE_WITH_KNOTS ( 'NONE', 3, 3, ( 
 ( #20658, #24276, #36335, #35840 ),
 ( #8616, #28605, #20398, #44244 ),
 ( #9363, #25267, #9117, #5762 ),
 ( #40918, #24776, #12453, #28114 ) ),
 .UNSPECIFIED., .F., .F., .F.,
 ( 4, 4 ),
 ( 4, 4 ),
 ( 0.000000000000000000, 1.000000000000000000 ),
 ( 0.000000000000000000, 1.000000000000000000 ),
 .UNSPECIFIED. ) ;
#3512=B_SPLINE_CURVE_WITH_KNOTS ( 'NONE', 3,
 ( #7569, #47780, #43465, #4726 ),
 .UNSPECIFIED., .F., .F.,
 ( 4, 4 ),
 ( 0.000000000000000000, 0.2637263876330691592 ),
 .UNSPECIFIED. ) ;
#3522=ORIENTED_EDGE ( 'NONE', *, *, #40149, .F. ) ;
#3523=EDGE_CURVE ( 'NONE', #18198, #23745, #13414, .T. ) ;
#3543=EDGE_CURVE ( 'NONE', #45635, #31056, #2421, .T. ) ;
#3545=CARTESIAN_POINT ( 'NONE',  ( 0.2401930789657907572, 1.414287202658143894, 9.950105812514292936 ) ) ;
#3561=CARTESIAN_POINT ( 'NONE',  ( -3.886636751349460628, 37.33392444503267171, 6.057468652304066836 ) ) ;
#3570=CARTESIAN_POINT ( 'NONE',  ( 14.29087950072012170, 9.652079258044652832, 8.727788335465566760 ) ) ;
#3573=CARTESIAN_POINT ( 'NONE',  ( 49.67735855322978011, -8.912210285361751971, 8.356839323120299312 ) ) ;
#3586=EDGE_CURVE ( 'NONE', #26037, #16958, #48900, .T. ) ;
#3590=ORIENTED_EDGE ( 'NONE', *, *, #24246, .T. ) ;
#3591=CARTESIAN_POINT ( 'NONE',  ( 0.8285222815141930486, 1.889008401827334094, 9.886433018048068178 ) ) ;
#3597=CARTESIAN_POINT ( 'NONE',  ( -32.92553608936650988, -17.96298651181783868, 8.100132398494512387 ) ) ;
#3605=CARTESIAN_POINT ( 'NONE',  ( 1.424123654779712922, 0.3625862473308184009, 9.958264684458541183 ) ) ;
#3608=EDGE_CURVE ( 'NONE', #50186, #2282, #22597, .T. ) ;
#3620=CARTESIAN_POINT ( 'NONE',  ( 29.39982726364966581, 16.78152490921169360, 8.356839323120299312 ) ) ;
#3633=EDGE_CURVE ( 'NONE', #31313, #449, #4866, .T. ) ;
#3644=CARTESIAN_POINT ( 'NONE',  ( -10.00000000000000533, -0.04986450829243618821, 8.654293224463934564 ) ) ;
#3654=ORIENTED_EDGE ( 'NONE', *, *, #8260, .T. ) ;
#3675=ORIENTED_EDGE ( 'NONE', *, *, #19025, .F. ) ;
#3679=B_SPLINE_CURVE_WITH_KNOTS ( 'NONE', 3,
 ( #22815, #30271, #6654, #2802 ),
 .UNSPECIFIED., .F., .F.,
 ( 4, 4 ),
 ( 0.000000000000000000, 0.002368422649471299893 ),
 .UNSPECIFIED. ) ;
#3714=B_SPLINE_CURVE_WITH_KNOTS ( 'NONE', 3,
 ( #5288, #43778, #8651, #24307, #952, #16591 ),
 .UNSPECIFIED., .F., .F.,
 ( 4, 2, 4 ),
 ( 8.673617379884035472E-19, 0.009882509389272365469, 0.01976501877854472747 ),
 .UNSPECIFIED. ) ;
#3715=CARTESIAN_POINT ( 'NONE',  ( 36.08557433729230723, -35.58569447144768105, 7.455576670931136185 ) ) ;
#3722=CARTESIAN_POINT ( 'NONE',  ( 8.277096487746778308, -50.00000000000000711, 7.455576670931136185 ) ) ;
#3731=EDGE_LOOP ( 'NONE', ( #32546, #41000, #20246, #21661 ) ) ;
#3733=VERTEX_POINT ( 'NONE', #285 ) ;
#3754=CARTESIAN_POINT ( 'NONE',  ( -0.2834763335384945515, 1.876787935831946141, 9.900811091504550632 ) ) ;
#3760=CARTESIAN_POINT ( 'NONE',  ( -0.2773062244624664441, 1.251557370488897813, 9.948547179989621014 ) ) ;
#3768=ORIENTED_EDGE ( 'NONE', *, *, #34779, .T. ) ;
#3771=CARTESIAN_POINT ( 'NONE',  ( -16.99749102614300966, 1.320765928724422222, 8.953103998512858652 ) ) ;
#3781=FACE_OUTER_BOUND ( 'NONE', #6382, .T. ) ;
#3783=ORIENTED_EDGE ( 'NONE', *, *, #25279, .F. ) ;
#3800=ORIENTED_EDGE ( 'NONE', *, *, #22070, .T. ) ;
#3801=CARTESIAN_POINT ( 'NONE',  ( -3.975459390375366997, -0.2195152216756601216, -2.642742795433417058E-16 ) ) ;
#3805=ORIENTED_EDGE ( 'NONE', *, *, #8270, .F. ) ;
#3811=CARTESIAN_POINT ( 'NONE',  ( -33.16902712922616558, 37.70469005304312304, 1.847720168420772691 ) ) ;
#3832=B_SPLINE_CURVE_WITH_KNOTS ( 'NONE', 3,
 ( #24714, #5700, #48256, #28301 ),
 .UNSPECIFIED., .F., .F.,
 ( 4, 4 ),
 ( 0.000000000000000000, 0.001246897409371959574 ),
 .UNSPECIFIED. ) ;
#3869=CARTESIAN_POINT ( 'NONE',  ( -16.50002041759928062, -3.070736177214532514, -9.233365092205394475 ) ) ;
#3872=B_SPLINE_CURVE_WITH_KNOTS ( 'NONE', 3,
 ( #49698, #18433, #41785, #14336 ),
 .UNSPECIFIED., .F., .F.,
 ( 4, 4 ),
 ( 0.000000000000000000, 0.0002610106747150516752 ),
 .UNSPECIFIED. ) ;
#3889=CARTESIAN_POINT ( 'NONE',  ( -0.3862712429686809279, -1.188820645368943163, -10.00000000000000000 ) ) ;
#3893=VERTEX_POINT ( 'NONE', #13575 ) ;
#3897=CARTESIAN_POINT ( 'NONE',  ( 0.000000000000000000, 0.000000000000000000, -10.00000000000000000 ) ) ;
#3901=CARTESIAN_POINT ( 'NONE',  ( 23.31729631074197329, 24.19776167542427814, -8.016098858316205167 ) ) ;
#3917=B_SPLINE_CURVE_WITH_KNOTS ( 'NONE', 3,
 ( #17755, #37528, #5691, #37032 ),
 .UNSPECIFIED., .F., .F.,
 ( 4, 4 ),
 ( 0.0002736185395732594399, 0.0005346342798032415345 ),
 .UNSPECIFIED. ) ;
#3929=CARTESIAN_POINT ( 'NONE',  ( -14.86945752723352498, -7.944783388878907004, 2.590526750877053086 ) ) ;
#3954=B_SPLINE_SURFACE_WITH_KNOTS ( 'NONE', 3, 3, ( 
 ( #14795, #45804, #6591, #2490 ),
 ( #30714, #14536, #26853, #2734 ),
 ( #41493, #18381, #34061, #2238 ),
 ( #34302, #46317, #49645, #10689 ) ),
 .UNSPECIFIED., .F., .F., .F.,
 ( 4, 4 ),
 ( 4, 4 ),
 ( 0.000000000000000000, 1.000000000000000000 ),
 ( 0.000000000000000000, 1.000000000000000000 ),
 .UNSPECIFIED. ) ;
#3958=CARTESIAN_POINT ( 'NONE',  ( 34.30563531518984632, 15.23322832906888991, 6.057468652304070389 ) ) ;
#3961=CARTESIAN_POINT ( 'NONE',  ( -0.4426377647354682865, -1.666766018367764834, 9.928159647716134018 ) ) ;
#3972=CARTESIAN_POINT ( 'NONE',  ( 1.114871695981101585, -0.4953159757246433093, 9.963925895596188909 ) ) ;
#3973=CARTESIAN_POINT ( 'NONE',  ( 0.6440276692615888310, 16.64212148744554298, -9.683996418299976483 ) ) ;
#3975=EDGE_CURVE ( 'NONE', #29168, #1639, #10342, .T. ) ;
#3976=EDGE_CURVE ( 'NONE', #32354, #9732, #9690, .T. ) ;
#3980=CARTESIAN_POINT ( 'NONE',  ( -1.011271242968677875, -0.7347315653656004697, 10.00000000000000000 ) ) ;
#3992=CARTESIAN_POINT ( 'NONE',  ( 7.576114424932982594, -50.00000000000000711, 7.906207997025717304 ) ) ;
#4004=EDGE_LOOP ( 'NONE', ( #45643, #20142, #21708, #8905 ) ) ;
#4005=CARTESIAN_POINT ( 'NONE',  ( 0.000000000000000000, 0.000000000000000000, 10.00000000000000000 ) ) ;
#4020=CARTESIAN_POINT ( 'NONE',  ( 32.87128375420895310, 6.537745902885608196, -8.466730184410787174 ) ) ;
#4025=CARTESIAN_POINT ( 'NONE',  ( 0.1287570809895604018, 0.3962735484563146282, 10.00000000000000000 ) ) ;
#4034=CARTESIAN_POINT ( 'NONE',  ( 23.83799721022594298, -28.99517291086361581, 3.209567239418974705 ) ) ;
#4039=CARTESIAN_POINT ( 'NONE',  ( 16.73672383626881199, 2.341008440548111302, -9.008049429158100807 ) ) ;
#4050=DIRECTION ( 'NONE',  ( -1.000000000000000000, 0.000000000000000000, 0.000000000000000000 ) ) ;
#4056=CARTESIAN_POINT ( 'NONE',  ( 9.760995290733820440, -2.173239732351728293, 9.646707543097347681 ) ) ;
#4060=CARTESIAN_POINT ( 'NONE',  ( 2.735102768439324983, -5.294960982149635953, 5.387129544537350156E-16 ) ) ;
#4071=CARTESIAN_POINT ( 'NONE',  ( 0.1287570809895630941, -0.3962735484563133515, 10.00000000000000000 ) ) ;
#4072=CARTESIAN_POINT ( 'NONE',  ( -4.763548243873389154, 16.57409059453848599, 8.727788335465566760 ) ) ;
#4073=CARTESIAN_POINT ( 'NONE',  ( 8.813458710706171928, 4.724716452304571490, 0.000000000000000000 ) ) ;
#4078=B_SPLINE_CURVE_WITH_KNOTS ( 'NONE', 3,
 ( #1510, #36422, #13541, #4827 ),
 .UNSPECIFIED., .F., .F.,
 ( 4, 4 ),
 ( 0.002217981418809652702, 0.002368422649471284280 ),
 .UNSPECIFIED. ) ;
#4082=CARTESIAN_POINT ( 'NONE',  ( -0.6538612634427415360, -1.160398818844775137, 9.951893257060017817 ) ) ;
#4086=CARTESIAN_POINT ( 'NONE',  ( -1.011271242968683204, -0.7347315653655928092, 9.972675548442467175 ) ) ;
#4100=EDGE_LOOP ( 'NONE', ( #10245, #1725, #31201, #13474, #10113, #50113, #38344, #30433, #8919, #20264, #3675, #23335 ) ) ;
#4110=CARTESIAN_POINT ( 'NONE',  ( -12.15085308559838317, 11.68662139125813226, 2.590526750877053086 ) ) ;
#4112=LINE ( 'NONE', #47172, #17541 ) ;
#4116=B_SPLINE_CURVE_WITH_KNOTS ( 'NONE', 3,
 ( #8925, #28675, #13520, #9174 ),
 .UNSPECIFIED., .F., .F.,
 ( 4, 4 ),
 ( 1.734723475976807094E-18, 2.804146970187102689E-05 ),
 .UNSPECIFIED. ) ;
#4120=ORIENTED_EDGE ( 'NONE', *, *, #26509, .T. ) ;
#4121=CARTESIAN_POINT ( 'NONE',  ( -1.250000000000000222, 0.000000000000000000, 10.00000000000000000 ) ) ;
#4127=EDGE_CURVE ( 'NONE', #323, #41298, #36624, .T. ) ;
#4132=CARTESIAN_POINT ( 'NONE',  ( 25.40454589245968364, 27.58367357691700406, -8.192531242611265085 ) ) ;
#4133=CARTESIAN_POINT ( 'NONE',  ( -33.08717642956897009, -5.870837526464926626, -8.016098858316205167 ) ) ;
#4137=EDGE_LOOP ( 'NONE', ( #43328, #16531, #2229, #20430, #253 ) ) ;
#4139=CARTESIAN_POINT ( 'NONE',  ( 29.18392875402930997, 17.44843138996603216, 7.906207997025717304 ) ) ;
#4141=ORIENTED_EDGE ( 'NONE', *, *, #39314, .T. ) ;
#4153=CARTESIAN_POINT ( 'NONE',  ( -0.5672860446885946706, -37.53182223685058716, -6.568693074176339408 ) ) ;
#4160=FACE_OUTER_BOUND ( 'NONE', #16280, .T. ) ;
#4180=ORIENTED_EDGE ( 'NONE', *, *, #37806, .F. ) ;
#4188=CARTESIAN_POINT ( 'NONE',  ( -48.33712804702535948, -13.03701565032741527, -9.367992836599954742 ) ) ;
#4189=EDGE_CURVE ( 'NONE', #32520, #12217, #8170, .T. ) ;
#4190=CARTESIAN_POINT ( 'NONE',  ( -0.8603719846020866369, 1.073163306095949121, 9.972175347158394487 ) ) ;
#4193=FACE_OUTER_BOUND ( 'NONE', #37782, .T. ) ;
#4213=CARTESIAN_POINT ( 'NONE',  ( 0.6665230861360139647, -1.119719016451030891, 9.961922210043265835 ) ) ;
#4214=CARTESIAN_POINT ( 'NONE',  ( 1.249999999999999778, 0.000000000000000000, 3.333333333333333481 ) ) ;
#4216=ORIENTED_EDGE ( 'NONE', *, *, #30705, .T. ) ;
#4225=CARTESIAN_POINT ( 'NONE',  ( -28.96803024440907137, -18.11533787072017176, 7.455576670931136185 ) ) ;
#4254=CARTESIAN_POINT ( 'NONE',  ( -2.538055338523177440, -50.00000000000000711, -9.367992836599954742 ) ) ;
#4259=CARTESIAN_POINT ( 'NONE',  ( -12.78770032058971395, -31.68259716188267916, 7.455576670931136185 ) ) ;
#4273=CARTESIAN_POINT ( 'NONE',  ( 2.920962725444330221, 37.39284056564468983, -9.011255500499645521 ) ) ;
#4274=ORIENTED_EDGE ( 'NONE', *, *, #33425, .T. ) ;
#4275=CARTESIAN_POINT ( 'NONE',  ( -5.107674452599877846, 2.961810711069517765, 9.586754400233969520 ) ) ;
#4284=CARTESIAN_POINT ( 'NONE',  ( 1.035950918207909632, 33.23661552194049307, -2.408242355805840784 ) ) ;
#4285=CARTESIAN_POINT ( 'NONE',  ( 8.569579719062522472, 5.179646911086180694, 3.092310436554641662 ) ) ;
#4300=CARTESIAN_POINT ( 'NONE',  ( 0.3862712429686978033, -1.188820645368937834, -3.333333333333333481 ) ) ;
#4303=ORIENTED_EDGE ( 'NONE', *, *, #2658, .F. ) ;
#4304=ADVANCED_FACE ( 'NONE', ( #28668 ), #44009, .T. ) ;
#4311=B_SPLINE_CURVE_WITH_KNOTS ( 'NONE', 3,
 ( #39254, #4353, #8206, #47649 ),
 .UNSPECIFIED., .F., .F.,
 ( 4, 4 ),
 ( 0.000000000000000000, 2.647279941188464684E-05 ),
 .UNSPECIFIED. ) ;
#4314=CARTESIAN_POINT ( 'NONE',  ( -1.337801958641930300, -1.088266084286974689, 9.928159647716134018 ) ) ;
#4315=ORIENTED_EDGE ( 'NONE', *, *, #13029, .T. ) ;
#4330=CARTESIAN_POINT ( 'NONE',  ( 3.996390545799824334, -16.57371371864897469, 8.953103998512858652 ) ) ;
#4331=CARTESIAN_POINT ( 'NONE',  ( -3.798817505216114387, -5.709742178110357891, 9.753789706659947711 ) ) ;
#4332=CARTESIAN_POINT ( 'NONE',  ( 1.655785408456140084, 0.7536129375913136474, 9.903764339332061795 ) ) ;
#4347=CARTESIAN_POINT ( 'NONE',  ( -28.96803024440907137, -18.11533787072017176, 7.455576670931136185 ) ) ;
#4348=CARTESIAN_POINT ( 'NONE',  ( 3.345242017215822372, -2.159124855890657724, -4.878909776184769953E-16 ) ) ;
#4349=CARTESIAN_POINT ( 'NONE',  ( -33.64889274059387958, 3.704246042440976439, 8.356839323120299312 ) ) ;
#4353=CARTESIAN_POINT ( 'NONE',  ( -0.9985466430029077411, -1.124040728744828188, 9.944962737616616977 ) ) ;
#4355=CARTESIAN_POINT ( 'NONE',  ( 49.46074318306830975, -9.578883844006833570, 8.807470649214879543 ) ) ;
#4362=CARTESIAN_POINT ( 'NONE',  ( 33.26055721649974117, 17.33465289285476985, 8.506357886886741326 ) ) ;
#4363=ORIENTED_EDGE ( 'NONE', *, *, #39990, .F. ) ;
#4376=VERTEX_POINT ( 'NONE', #22480 ) ;
#4379=B_SPLINE_SURFACE_WITH_KNOTS ( 'NONE', 3, 3, ( 
 ( #20646, #28352, #12192, #36321 ),
 ( #43734, #8603, #1415, #8355 ),
 ( #24258, #39914, #48302, #9106 ),
 ( #1164, #36064, #47804, #13196 ) ),
 .UNSPECIFIED., .F., .F., .F.,
 ( 4, 4 ),
 ( 4, 4 ),
 ( 0.000000000000000000, 1.000000000000000000 ),
 ( 0.000000000000000000, 1.000000000000000000 ),
 .UNSPECIFIED. ) ;
#4382=CARTESIAN_POINT ( 'NONE',  ( 46.11867747200574286, -19.86470446310233129, -8.016098858316205167 ) ) ;
#4390=FACE_OUTER_BOUND ( 'NONE', #29976, .T. ) ;
#4394=CARTESIAN_POINT ( 'NONE',  ( 6.208157169185024138, -36.98937201184289592, 8.506357886886741326 ) ) ;
#4396=CARTESIAN_POINT ( 'NONE',  ( -1.011271242968683426, -0.7347315653655928092, -3.333333333333333481 ) ) ;
#4398=CARTESIAN_POINT ( 'NONE',  ( 31.44259251615245887, 38.95901822126168668, -9.367992836599954742 ) ) ;
#4414=CARTESIAN_POINT ( 'NONE',  ( 21.61731705588930907, 25.43568671410602278, -9.367992836599954742 ) ) ;
#4426=VERTEX_POINT ( 'NONE', #7092 ) ;
#4440=CARTESIAN_POINT ( 'NONE',  ( -18.38319608353667434, 32.68498281710182596, -8.192531242611268638 ) ) ;
#4443=EDGE_LOOP ( 'NONE', ( #39054, #15018, #25441, #37982 ) ) ;
#4452=VERTEX_POINT ( 'NONE', #18864 ) ;
#4460=FACE_OUTER_BOUND ( 'NONE', #3484, .T. ) ;
#4461=CARTESIAN_POINT ( 'NONE',  ( 1.011271242968677653, 0.7347315653656002477, 10.00000000000000000 ) ) ;
#4463=ORIENTED_EDGE ( 'NONE', *, *, #9414, .F. ) ;
#4474=CARTESIAN_POINT ( 'NONE',  ( -2.538055338523177440, -33.28424297489108596, -9.367992836599954742 ) ) ;
#4476=CARTESIAN_POINT ( 'NONE',  ( 46.76852358249013264, -17.86468378716708827, -9.367992836599951190 ) ) ;
#4482=EDGE_CURVE ( 'NONE', #29168, #9976, #32238, .T. ) ;
#4483=CARTESIAN_POINT ( 'NONE',  ( 30.21887974406487487, -14.69854701517530060, -8.016098858316199838 ) ) ;
#4490=FACE_OUTER_BOUND ( 'NONE', #5885, .T. ) ;
#4497=EDGE_CURVE ( 'NONE', #20753, #29288, #19415, .T. ) ;
#4499=CARTESIAN_POINT ( 'NONE',  ( -50.11058929355266400, 7.578863168071933387, 7.455576670931136185 ) ) ;
#4500=EDGE_CURVE ( 'NONE', #24077, #6277, #35834, .T. ) ;
#4503=CARTESIAN_POINT ( 'NONE',  ( 1.045807400993768788, -0.6549210616167769894, 9.969907203203808521 ) ) ;
#4507=CARTESIAN_POINT ( 'NONE',  ( 1.632255792517797621, -3.624924591517686867, 3.247138655587366696 ) ) ;
#4513=CARTESIAN_POINT ( 'NONE',  ( 0.1287570809895575430, 0.3962735484563150168, 10.00000000000000000 ) ) ;
#4519=CARTESIAN_POINT ( 'NONE',  ( 17.51065725283126895, -28.41934970907778890, -9.367992836599954742 ) ) ;
#4524=EDGE_CURVE ( 'NONE', #11547, #22255, #39599, .T. ) ;
#4533=CARTESIAN_POINT ( 'NONE',  ( -0.7455485644579464832, -0.9687920084208885285, 9.987567862361071747 ) ) ;
#4535=ORIENTED_EDGE ( 'NONE', *, *, #22988, .F. ) ;
#4550=ORIENTED_EDGE ( 'NONE', *, *, #41213, .F. ) ;
#4551=FACE_OUTER_BOUND ( 'NONE', #27339, .T. ) ;
#4552=CARTESIAN_POINT ( 'NONE',  ( 34.38425513258721367, -36.82177522737820397, 8.807470649214879543 ) ) ;
#4554=EDGE_LOOP ( 'NONE', ( #46438, #2822, #42039 ) ) ;
#4560=FACE_OUTER_BOUND ( 'NONE', #4137, .T. ) ;
#4564=CARTESIAN_POINT ( 'NONE',  ( 24.47767542868285062, -23.18653802921781448, 8.807470649214879543 ) ) ;
#4566=ORIENTED_EDGE ( 'NONE', *, *, #31121, .F. ) ;
#4569=ORIENTED_EDGE ( 'NONE', *, *, #20828, .T. ) ;
#4572=ADVANCED_FACE ( 'NONE', ( #37780 ), #29303, .T. ) ;
#4582=CARTESIAN_POINT ( 'NONE',  ( 3.229232847726260403, -16.57333684275945629, 9.178419661560148768 ) ) ;
#4586=CARTESIAN_POINT ( 'NONE',  ( -10.00000000000117062, 0.7319447344825763535, 9.406212099229145807 ) ) ;
#4587=CARTESIAN_POINT ( 'NONE',  ( 32.57170742938662755, 18.58316106410423174, 7.697694107796188234 ) ) ;
#4600=CARTESIAN_POINT ( 'NONE',  ( 2.242409830259191494, -37.46921084408874947, 3.209567239418970708 ) ) ;
#4601=CARTESIAN_POINT ( 'NONE',  ( -0.3862712429686977478, 1.188820645368937390, 10.00000000000000000 ) ) ;
#4609=CARTESIAN_POINT ( 'NONE',  ( 48.99656738986517723, -11.00747004110342431, 1.847720168420772691 ) ) ;
#4631=CARTESIAN_POINT ( 'NONE',  ( -1.250000000000000222, 0.000000000000000000, 3.333333333333333481 ) ) ;
#4635=EDGE_CURVE ( 'NONE', #23429, #35155, #31705, .T. ) ;
#4648=CARTESIAN_POINT ( 'NONE',  ( -0.3862712429686977478, 1.188820645368937390, 10.00000000000000000 ) ) ;
#4656=CARTESIAN_POINT ( 'NONE',  ( -1.011271242968683426, -0.7347315653655928092, 10.00000000000000000 ) ) ;
#4662=CARTESIAN_POINT ( 'NONE',  ( -2.210477865340801706, -37.43479381012853224, -9.422646554964178023 ) ) ;
#4670=CARTESIAN_POINT ( 'NONE',  ( -13.92102703536724384, -30.85732372859812500, 8.356839323120299312 ) ) ;
#4682=CARTESIAN_POINT ( 'NONE',  ( 0.3862712429686727678, 1.188820645368945605, 10.00000000000000000 ) ) ;
#4699=CARTESIAN_POINT ( 'NONE',  ( 2.538055338523177440, 33.28424297489108596, -9.367992836599954742 ) ) ;
#4711=ORIENTED_EDGE ( 'NONE', *, *, #40067, .F. ) ;
#4713=CARTESIAN_POINT ( 'NONE',  ( 0.9494396179258391966, -9.954826186926261755, 9.646707543097345905 ) ) ;
#4726=CARTESIAN_POINT ( 'NONE',  ( -37.27397286063865778, 4.111076158911805223, 7.697694107796192675 ) ) ;
#4737=CARTESIAN_POINT ( 'NONE',  ( 7.749480817862238524, 14.85497772329518895, 9.403735324607438884 ) ) ;
#4743=CARTESIAN_POINT ( 'NONE',  ( 7.608425291889091113, -36.72004717559254772, 7.697694107796188234 ) ) ;
#4751=CARTESIAN_POINT ( 'NONE',  ( -18.69789054174323084, 27.49790346457746182, -2.408242355805840784 ) ) ;
#4754=CARTESIAN_POINT ( 'NONE',  ( 0.9870575514054733546, 1.980598328282569653, 9.881002359080278907 ) ) ;
#4766=ORIENTED_EDGE ( 'NONE', *, *, #46361, .T. ) ;
#4769=CARTESIAN_POINT ( 'NONE',  ( 1.011271242968683648, 0.7347315653655930312, -10.00000000000000000 ) ) ;
#4770=CARTESIAN_POINT ( 'NONE',  ( -0.6721397084974984892, -9.977385840602783773, 0.000000000000000000 ) ) ;
#4780=CARTESIAN_POINT ( 'NONE',  ( 1.011271242968677653, 0.7347315653656002477, 10.00000000000000000 ) ) ;
#4783=B_SPLINE_SURFACE_WITH_KNOTS ( 'NONE', 3, 3, ( 
 ( #39406, #35554, #4737, #8347 ),
 ( #395, #20890, #36060, #12186 ),
 ( #31954, #40405, #16042, #43475 ),
 ( #39908, #44223, #5241, #23990 ) ),
 .UNSPECIFIED., .F., .F., .F.,
 ( 4, 4 ),
 ( 4, 4 ),
 ( 0.000000000000000000, 1.000000000000000000 ),
 ( 0.000000000000000000, 1.000000000000000000 ),
 .UNSPECIFIED. ) ;
#4784=VERTEX_POINT ( 'NONE', #14915 ) ;
#4786=CARTESIAN_POINT ( 'NONE',  ( 45.64490844644691236, 21.32281559348795952, 8.807470649214879543 ) ) ;
#4788=CARTESIAN_POINT ( 'NONE',  ( 1.917969350850768029, -0.3547183498316657801, 9.896382706792435258 ) ) ;
#4792=ORIENTED_EDGE ( 'NONE', *, *, #4127, .F. ) ;
#4795=CARTESIAN_POINT ( 'NONE',  ( -31.44259251615275019, -38.95901822126145220, -9.367992836599954742 ) ) ;
#4799=CARTESIAN_POINT ( 'NONE',  ( -1.011271242968677875, -0.7347315653656004697, 10.00000000000000000 ) ) ;
#4814=CARTESIAN_POINT ( 'NONE',  ( 0.09523839817332763191, 1.466467394239034050, 9.958264684458713489 ) ) ;
#4823=CARTESIAN_POINT ( 'NONE',  ( 0.1287570809895630941, -0.3962735484563133515, 10.00000000000000000 ) ) ;
#4827=CARTESIAN_POINT ( 'NONE',  ( -9.998889670239194061, -0.1490146381531308739, 9.282506307616474217 ) ) ;
#4838=CARTESIAN_POINT ( 'NONE',  ( -1.011271242968688533, 0.7347315653655859258, -10.00000000000000000 ) ) ;
#4846=ORIENTED_EDGE ( 'NONE', *, *, #45236, .F. ) ;
#4866=B_SPLINE_CURVE_WITH_KNOTS ( 'NONE', 3,
 ( #18993, #31071, #39033, #22604, #15162, #22849 ),
 .UNSPECIFIED., .F., .F.,
 ( 4, 2, 4 ),
 ( 4.982613841084487634E-17, 0.009882509389272372408, 0.01976501877854469277 ),
 .UNSPECIFIED. ) ;
#4871=DIRECTION ( 'NONE',  ( 0.000000000000000000, 0.000000000000000000, -1.000000000000000000 ) ) ;
#4898=ADVANCED_FACE ( 'NONE', ( #16189 ), #24403, .F. ) ;
#4916=CARTESIAN_POINT ( 'NONE',  ( 4.641001526964561030, 50.00000000000000000, -8.016098858316205167 ) ) ;
#4943=EDGE_LOOP ( 'NONE', ( #49783, #19621, #40461 ) ) ;
#4955=CARTESIAN_POINT ( 'NONE',  ( 2.210477865340801706, 37.43479381012853224, -9.422646554964178023 ) ) ;
#4956=CARTESIAN_POINT ( 'NONE',  ( 1.249999999999999778, -0.000000000000000000, -3.333333333333333481 ) ) ;
#4958=B_SPLINE_CURVE_WITH_KNOTS ( 'NONE', 3,
 ( #46506, #43632, #5142, #42687 ),
 .UNSPECIFIED., .F., .F.,
 ( 4, 4 ),
 ( 0.9688112071879386722, 0.9724175925769219520 ),
 .UNSPECIFIED. ) ;
#4965=EDGE_CURVE ( 'NONE', #9737, #35077, #42029, .T. ) ;
#4972=ADVANCED_FACE ( 'NONE', ( #21800 ), #21088, .T. ) ;
#4978=CARTESIAN_POINT ( 'NONE',  ( -30.77287599203642188, -12.70002479445974686, 3.199614146704519602 ) ) ;
#4980=CARTESIAN_POINT ( 'NONE',  ( 9.999999999999994671, 0.04964634316242984985, 9.296265711053614211 ) ) ;
#5003=B_SPLINE_CURVE_WITH_KNOTS ( 'NONE', 3,
 ( #50365, #22954, #42206, #39143 ),
 .UNSPECIFIED., .F., .F.,
 ( 4, 4 ),
 ( 0.0001535465953326383131, 0.0005837444810855588412 ),
 .UNSPECIFIED. ) ;
#5004=CARTESIAN_POINT ( 'NONE',  ( 1.011271242968688311, -0.7347315653655855927, 10.00000000000000000 ) ) ;
#5005=FACE_OUTER_BOUND ( 'NONE', #31134, .T. ) ;
#5024=CARTESIAN_POINT ( 'NONE',  ( -1.872530400643504400, 0.3103573527827566680, 9.900811091504554184 ) ) ;
#5027=CARTESIAN_POINT ( 'NONE',  ( -1.275994128725546739, 0.1230186051320636409, 9.948547179989615685 ) ) ;
#5028=CARTESIAN_POINT ( 'NONE',  ( -48.98697415750977768, -11.03699497439218646, -8.016098858316199838 ) ) ;
#5031=EDGE_CURVE ( 'NONE', #10907, #21273, #49200, .T. ) ;
#5039=CARTESIAN_POINT ( 'NONE',  ( 4.641001526964560142, 50.00000000000000711, -8.016098858316199838 ) ) ;
#5045=EDGE_LOOP ( 'NONE', ( #35830, #8512, #6821, #35832, #38909, #31294, #7414, #40020, #46003, #49566, #30367, #37292 ) ) ;
#5049=CARTESIAN_POINT ( 'NONE',  ( -4.763548243873389154, 16.57409059453848599, 8.727788335465566760 ) ) ;
#5055=CARTESIAN_POINT ( 'NONE',  ( 23.26005729352310425, 44.90397804740356236, 7.906207997025717304 ) ) ;
#5080=B_SPLINE_CURVE_WITH_KNOTS ( 'NONE', 3,
 ( #48756, #13648, #29307, #44913 ),
 .UNSPECIFIED., .F., .F.,
 ( 4, 4 ),
 ( 3.397412858278222916E-17, 0.0004072981213156856356 ),
 .UNSPECIFIED. ) ;
#5093=B_SPLINE_SURFACE_WITH_KNOTS ( 'NONE', 3, 3, ( 
 ( #23002, #26363, #46066, #6860 ),
 ( #49895, #27125, #7116, #38678 ),
 ( #10958, #22502, #2998, #42258 ),
 ( #34841, #50421, #27375, #30984 ) ),
 .UNSPECIFIED., .F., .F., .F.,
 ( 4, 4 ),
 ( 4, 4 ),
 ( 0.000000000000000000, 1.000000000000000000 ),
 ( 0.000000000000000000, 1.000000000000000000 ),
 .UNSPECIFIED. ) ;
#5094=B_SPLINE_CURVE_WITH_KNOTS ( 'NONE', 3,
 ( #46591, #23550, #50437, #38957 ),
 .UNSPECIFIED., .F., .F.,
 ( 4, 4 ),
 ( 0.000000000000000000, 0.0001252128669263237850 ),
 .UNSPECIFIED. ) ;
#5105=CARTESIAN_POINT ( 'NONE',  ( -6.174150299305392053, 33.14591993373988998, 8.807470649214879543 ) ) ;
#5110=CARTESIAN_POINT ( 'NONE',  ( -8.640097307817388383, 14.29292567250791102, -9.458680755252684591 ) ) ;
#5126=CARTESIAN_POINT ( 'NONE',  ( 1.337801958641917199, 1.088266084286984015, 9.928159647716135794 ) ) ;
#5127=FACE_OUTER_BOUND ( 'NONE', #34294, .T. ) ;
#5131=ADVANCED_FACE ( 'NONE', ( #35142 ), #12027, .F. ) ;
#5135=CARTESIAN_POINT ( 'NONE',  ( -0.6108107228405769140, 1.056024183042602482, 9.963925895596188909 ) ) ;
#5142=CARTESIAN_POINT ( 'NONE',  ( -2.097926912204285177, 0.2448757052704424453, 9.890170120223997330 ) ) ;
#5145=CARTESIAN_POINT ( 'NONE',  ( -2.052549611693787135, 0.2039603569406744088, 9.894754715216729224 ) ) ;
#5161=B_SPLINE_CURVE_WITH_KNOTS ( 'NONE', 3,
 ( #19063, #34752, #47249, #4440 ),
 .UNSPECIFIED., .F., .F.,
 ( 4, 4 ),
 ( 0.000000000000000000, 0.2545280377015988749 ),
 .UNSPECIFIED. ) ;
#5166=CARTESIAN_POINT ( 'NONE',  ( -5.320787806781440921, 8.466948512633457824, -1.544988095791843818E-15 ) ) ;
#5168=B_SPLINE_CURVE_WITH_KNOTS ( 'NONE', 3,
 ( #39715, #24814, #4788, #29169 ),
 .UNSPECIFIED., .F., .F.,
 ( 4, 4 ),
 ( 2.262036551361258466E-17, 0.0004072981213155198611 ),
 .UNSPECIFIED. ) ;
#5171=CARTESIAN_POINT ( 'NONE',  ( -10.00000000000000533, 0.4417425667975929948, 5.558078895815943277 ) ) ;
#5172=CARTESIAN_POINT ( 'NONE',  ( 16.76006782980217125, -2.050259795448531541, 9.178419661560148768 ) ) ;
#5183=CARTESIAN_POINT ( 'NONE',  ( 0.000000000000000000, 0.000000000000000000, 0.000000000000000000 ) ) ;
#5189=B_SPLINE_CURVE_WITH_KNOTS ( 'NONE', 3,
 ( #35279, #27311, #42433, #34507 ),
 .UNSPECIFIED., .F., .F.,
 ( 4, 4 ),
 ( 0.000000000000000000, 0.2637263876330695478 ),
 .UNSPECIFIED. ) ;
#5197=VERTEX_POINT ( 'NONE', #46872 ) ;
#5199=VERTEX_POINT ( 'NONE', #19716 ) ;
#5204=EDGE_CURVE ( 'NONE', #49960, #8523, #49876, .T. ) ;
#5216=CARTESIAN_POINT ( 'NONE',  ( 13.59579750444771307, -10.60877755095900632, 8.727788335465566760 ) ) ;
#5218=B_SPLINE_SURFACE_WITH_KNOTS ( 'NONE', 3, 3, ( 
 ( #28915, #45039, #5049, #13754 ),
 ( #28663, #32534, #24820, #44791 ),
 ( #29414, #1229, #41210, #9913 ),
 ( #44530, #9662, #44043, #20710 ) ),
 .UNSPECIFIED., .F., .F., .F.,
 ( 4, 4 ),
 ( 4, 4 ),
 ( 0.000000000000000000, 1.000000000000000000 ),
 ( 0.000000000000000000, 1.000000000000000000 ),
 .UNSPECIFIED. ) ;
#5233=CARTESIAN_POINT ( 'NONE',  ( 24.39427009665985224, 44.07992421011656603, 8.807470649214879543 ) ) ;
#5240=CARTESIAN_POINT ( 'NONE',  ( -6.408332700304190332, -7.676800896350769676, 0.000000000000000000 ) ) ;
#5241=CARTESIAN_POINT ( 'NONE',  ( 5.888214538810389698, 16.20866436362417673, 8.727788335465566760 ) ) ;
#5257=ORIENTED_EDGE ( 'NONE', *, *, #3608, .T. ) ;
#5258=CARTESIAN_POINT ( 'NONE',  ( -15.73090589902298042, -29.60029367929041655, 1.847720168420772691 ) ) ;
#5259=EDGE_CURVE ( 'NONE', #38406, #13052, #15736, .T. ) ;
#5265=FACE_OUTER_BOUND ( 'NONE', #42762, .T. ) ;
#5276=DIRECTION ( 'NONE',  ( 0.8090169943749465631, 0.5877852522924742473, 0.000000000000000000 ) ) ;
#5278=EDGE_CURVE ( 'NONE', #46833, #29795, #28929, .T. ) ;
#5288=CARTESIAN_POINT ( 'NONE',  ( -32.57170742938676256, -18.58316106410400437, 7.697694107796192675 ) ) ;
#5295=CARTESIAN_POINT ( 'NONE',  ( -1.553222296440334826, 1.431397764604077860, 9.884520316594374023 ) ) ;
#5297=CARTESIAN_POINT ( 'NONE',  ( -33.86622497129646092, 3.037805405905158462, 7.906207997025717304 ) ) ;
#5301=CARTESIAN_POINT ( 'NONE',  ( -5.505322767148756569, 37.09368438467003415, 8.914903342594564961 ) ) ;
#5309=CARTESIAN_POINT ( 'NONE',  ( 0.3862712429686894211, -1.188820645368940276, 9.972675548442463622 ) ) ;
#5311=CARTESIAN_POINT ( 'NONE',  ( -25.60949810002096783, -43.19700938445173932, 1.847720168420772691 ) ) ;
#5315=CARTESIAN_POINT ( 'NONE',  ( 12.78770032058947237, 31.68259716188277864, 7.455576670931136185 ) ) ;
#5332=CARTESIAN_POINT ( 'NONE',  ( 25.63461350838963426, -43.17876197216376966, -8.016098858316199838 ) ) ;
#5336=CARTESIAN_POINT ( 'NONE',  ( 15.57957361750251302, 5.755602074545510760, 3.266473740018926541 ) ) ;
#5339=CARTESIAN_POINT ( 'NONE',  ( -11.73320209285699889, 11.96063479729179768, 9.403735324607438884 ) ) ;
#5354=CARTESIAN_POINT ( 'NONE',  ( -0.4402948852767746279, 2.015117899693936732, 9.894754715216722118 ) ) ;
#5359=EDGE_LOOP ( 'NONE', ( #4141, #20638, #11759, #36577, #24083, #2743, #17002, #41325, #14180, #1513, #25332, #49327 ) ) ;
#5361=MANIFOLD_SOLID_BREP ( 'CirPattern1', #23649 ) ;
#5364=CARTESIAN_POINT ( 'NONE',  ( -6.875132362119187768, 50.00000000000000711, 8.356839323120299312 ) ) ;
#5367=CARTESIAN_POINT ( 'NONE',  ( 0.8433491450857230065, -0.9182416014173362395, 9.981352469109934233 ) ) ;
#5396=CARTESIAN_POINT ( 'NONE',  ( -14.52758583651993618, -8.922352469211071835, 8.953103998512858652 ) ) ;
#5400=CARTESIAN_POINT ( 'NONE',  ( 25.40454589245968364, 27.58367357691700406, -8.192531242611265085 ) ) ;
#5401=CARTESIAN_POINT ( 'NONE',  ( -48.33712804702535948, -13.03701565032741527, -9.367992836599954742 ) ) ;
#5421=CARTESIAN_POINT ( 'NONE',  ( 0.7604583772899720095, -1.297021979204312725, 9.944962737616615200 ) ) ;
#5425=CARTESIAN_POINT ( 'NONE',  ( 30.12518629743562926, 14.70074613238908157, 1.847720168420772691 ) ) ;
#5434=ORIENTED_EDGE ( 'NONE', *, *, #16175, .T. ) ;
#5448=CARTESIAN_POINT ( 'NONE',  ( 48.34672127938079456, -13.00749071703866555, 3.199614146704519602 ) ) ;
#5451=CARTESIAN_POINT ( 'NONE',  ( -8.277096487746778308, 50.00000000000000711, 7.455576670931136185 ) ) ;
#5452=B_SPLINE_CURVE_WITH_KNOTS ( 'NONE', 3,
 ( #42868, #35726, #19013, #308 ),
 .UNSPECIFIED., .F., .F.,
 ( 4, 4 ),
 ( 0.0004536450142761632299, 0.006592155078637213644 ),
 .UNSPECIFIED. ) ;
#5459=CARTESIAN_POINT ( 'NONE',  ( 7.303894382572782007, -3.196591120352752835, -1.423015351387224570E-15 ) ) ;
#5468=CARTESIAN_POINT ( 'NONE',  ( -1.104213410210672430, -0.6509177773818179968, 9.976582533991678048 ) ) ;
#5474=CARTESIAN_POINT ( 'NONE',  ( 9.174209336589868258, 3.979181203266223488, 9.646707543097347681 ) ) ;
#5482=CARTESIAN_POINT ( 'NONE',  ( -0.3370904143228978245, 0.2449105217885259589, 10.00000000000000000 ) ) ;
#5483=CARTESIAN_POINT ( 'NONE',  ( 9.221081804193270059, 13.81382350053991104, 3.266473740018926541 ) ) ;
#5491=CARTESIAN_POINT ( 'NONE',  ( -5.083187235775261215, -8.611690166631138510, 9.646707543097347681 ) ) ;
#5493=CARTESIAN_POINT ( 'NONE',  ( 32.43949840348898306, 7.871562655726499713, -9.367992836599954742 ) ) ;
#5495=ORIENTED_EDGE ( 'NONE', *, *, #21814, .F. ) ;
#5516=CARTESIAN_POINT ( 'NONE',  ( 33.64889274059390090, -3.704246042440748621, 8.356839323120299312 ) ) ;
#5524=VERTEX_POINT ( 'NONE', #11704 ) ;
#5526=CARTESIAN_POINT ( 'NONE',  ( -16.69947034530963847, 2.312583065866374632, 2.590526750877053086 ) ) ;
#5527=CARTESIAN_POINT ( 'NONE',  ( 2.052581215100350853, -0.2042358160480859663, 9.886433018048069954 ) ) ;
#5529=DIRECTION ( 'NONE',  ( -0.000000000000000000, -0.000000000000000000, -1.000000000000000000 ) ) ;
#5531=B_SPLINE_CURVE_WITH_KNOTS ( 'NONE', 3,
 ( #24050, #20184, #9140, #686 ),
 .UNSPECIFIED., .F., .F.,
 ( 4, 4 ),
 ( 0.0006669682284780770491, 0.0007799402130932136645 ),
 .UNSPECIFIED. ) ;
#5537=CARTESIAN_POINT ( 'NONE',  ( 25.40454589245968364, 27.58367357691700406, -8.192531242611265085 ) ) ;
#5539=ADVANCED_FACE ( 'NONE', ( #20156 ), #49336, .T. ) ;
#5543=CARTESIAN_POINT ( 'NONE',  ( 36.08557433729230723, -35.58569447144768105, 7.455576670931136185 ) ) ;
#5549=CARTESIAN_POINT ( 'NONE',  ( -49.89397392339119364, 8.245536726717011433, 7.906207997025717304 ) ) ;
#5561=CARTESIAN_POINT ( 'NONE',  ( 35.51958307830769002, -12.13749199045042282, -6.568693074176326085 ) ) ;
#5573=CARTESIAN_POINT ( 'NONE',  ( -0.3334286742303091411, -1.332255019526853435, 9.946805383069623474 ) ) ;
#5580=CARTESIAN_POINT ( 'NONE',  ( 1.011271242968683648, 0.7347315653655930312, 9.972675548442463622 ) ) ;
#5581=CARTESIAN_POINT ( 'NONE',  ( 16.73672383626881199, 2.341008440548111302, -9.008049429158100807 ) ) ;
#5594=CARTESIAN_POINT ( 'NONE',  ( -1.468446590252919348, -0.3226319952343834063, 9.953784399990620813 ) ) ;
#5595=ORIENTED_EDGE ( 'NONE', *, *, #15505, .T. ) ;
#5596=CARTESIAN_POINT ( 'NONE',  ( -22.75063655912460447, -24.61040335498469389, -8.466730184410787174 ) ) ;
#5603=ORIENTED_EDGE ( 'NONE', *, *, #31809, .F. ) ;
#5624=EDGE_LOOP ( 'NONE', ( #47004, #28637, #40172 ) ) ;
#5628=B_SPLINE_SURFACE_WITH_KNOTS ( 'NONE', 3, 3, ( 
 ( #30951, #7850, #31196, #50632 ),
 ( #39654, #43483, #400, #7327 ),
 ( #46784, #8354, #19378, #23495 ),
 ( #19630, #42968, #42461, #47302 ) ),
 .UNSPECIFIED., .F., .F., .F.,
 ( 4, 4 ),
 ( 4, 4 ),
 ( 0.000000000000000000, 1.000000000000000000 ),
 ( 0.000000000000000000, 1.000000000000000000 ),
 .UNSPECIFIED. ) ;
#5629=VERTEX_POINT ( 'NONE', #2672 ) ;
#5638=CARTESIAN_POINT ( 'NONE',  ( -0.5107275442771143092, -1.175643901748072873, 9.976582533991681601 ) ) ;
#5647=CARTESIAN_POINT ( 'NONE',  ( -27.33593271309441519, 41.94268121623345991, -9.367992836599954742 ) ) ;
#5660=CARTESIAN_POINT ( 'NONE',  ( -0.09523839817533703844, -1.466467394240187350, 9.958264684458541183 ) ) ;
#5672=CARTESIAN_POINT ( 'NONE',  ( 2.769912820522884456, -9.621098677754085671, 6.185594734181534271 ) ) ;
#5676=CARTESIAN_POINT ( 'NONE',  ( 46.10908423965007330, 19.89422939639137766, 1.847720168420772691 ) ) ;
#5691=CARTESIAN_POINT ( 'NONE',  ( 1.231029138816503110, 0.08486683738666057908, 9.969907237807635880 ) ) ;
#5692=FACE_OUTER_BOUND ( 'NONE', #17024, .T. ) ;
#5700=CARTESIAN_POINT ( 'NONE',  ( -4.135284104686786393E-15, 0.4183134307191331280, 9.992713367193012175 ) ) ;
#5703=CARTESIAN_POINT ( 'NONE',  ( 2.538055338523177440, 50.00000000000000711, -9.367992836599954742 ) ) ;
#5710=CARTESIAN_POINT ( 'NONE',  ( -1.377636575563021992, 0.6021164824561227036, 9.953784399990620813 ) ) ;
#5728=CARTESIAN_POINT ( 'NONE',  ( 15.80799809827372648, -29.65358618225706522, -8.016098858316205167 ) ) ;
#5731=CARTESIAN_POINT ( 'NONE',  ( 23.82716369509147825, 44.49195112876006419, 8.356839323120299312 ) ) ;
#5734=CARTESIAN_POINT ( 'NONE',  ( -8.277096487746778308, 45.55573069994827051, 7.455576670931136185 ) ) ;
#5738=CARTESIAN_POINT ( 'NONE',  ( -2.538055338523173443, -50.00000000000000711, -9.367992836599951190 ) ) ;
#5744=PLANE ( 'NONE',  #19042 ) ;
#5751=VECTOR ( 'NONE', #15847, 1000.000000000000114 ) ;
#5762=CARTESIAN_POINT ( 'NONE',  ( -0.1287570809895658697, 0.3962735484563123523, 10.00000000000000000 ) ) ;
#5765=EDGE_CURVE ( 'NONE', #50249, #43903, #15704, .T. ) ;
#5767=CARTESIAN_POINT ( 'NONE',  ( -2.277966102372183776, 9.750758063795943897, 3.092157797347716119 ) ) ;
#5785=CARTESIAN_POINT ( 'NONE',  ( -1.437255894074058515, 3.713052624461494755, 6.606856988583542645E-16 ) ) ;
#5788=CARTESIAN_POINT ( 'NONE',  ( 4.763548243873389154, -16.57409059453848599, 8.727788335465566760 ) ) ;
#5795=CARTESIAN_POINT ( 'NONE',  ( -24.39427009666018265, -44.07992421011638129, 8.807470649214879543 ) ) ;
#5799=CARTESIAN_POINT ( 'NONE',  ( -18.38319608353667434, 32.68498281710182596, -8.192531242611268638 ) ) ;
#5802=B_SPLINE_CURVE_WITH_KNOTS ( 'NONE', 3,
 ( #3353, #14404, #10547, #49510 ),
 .UNSPECIFIED., .F., .F.,
 ( 4, 4 ),
 ( 2.954445946614352819E-17, 0.0004072981213157676555 ),
 .UNSPECIFIED. ) ;
#5807=EDGE_CURVE ( 'NONE', #15843, #17906, #45660, .T. ) ;
#5817=CARTESIAN_POINT ( 'NONE',  ( 7.359817328027030925, 15.16751262232805431, 2.590526750877053086 ) ) ;
#5844=CARTESIAN_POINT ( 'NONE',  ( -8.277096487746778308, 50.00000000000000000, 7.455576670931136185 ) ) ;
#5850=CARTESIAN_POINT ( 'NONE',  ( -0.1287570809895632329, 0.3962735484563137400, 10.00000000000000000 ) ) ;
#5855=CARTESIAN_POINT ( 'NONE',  ( -2.210477865340801706, -37.43479381012853224, -9.422646554964178023 ) ) ;
#5868=CARTESIAN_POINT ( 'NONE',  ( -13.92102703536724384, -30.85732372859812500, 8.356839323120299312 ) ) ;
#5883=CARTESIAN_POINT ( 'NONE',  ( -1.193089574352124149, -0.2545860991493743564, 9.963925895596188909 ) ) ;
#5885=EDGE_LOOP ( 'NONE', ( #39929, #19884, #19687, #34576 ) ) ;
#5886=CARTESIAN_POINT ( 'NONE',  ( 0.7606162131530698201, -1.296876929034913140, 9.953784399990620813 ) ) ;
#5887=CARTESIAN_POINT ( 'NONE',  ( -2.462075149652696027, 16.57295996686994499, 9.403735324607438884 ) ) ;
#5897=VERTEX_POINT ( 'NONE', #16966 ) ;
#5901=CARTESIAN_POINT ( 'NONE',  ( -1.011271242968677875, -0.7347315653656004697, -10.00000000000000000 ) ) ;
#5903=CARTESIAN_POINT ( 'NONE',  ( -26.18032376592659105, 21.95228666728381128, 7.455576670931136185 ) ) ;
#5904=VERTEX_POINT ( 'NONE', #38503 ) ;
#5913=CARTESIAN_POINT ( 'NONE',  ( -7.576114424932982594, 50.00000000000000711, 7.906207997025717304 ) ) ;
#5931=CARTESIAN_POINT ( 'NONE',  ( 0.3862712429686810944, 1.188820645368943607, 10.00000000000000000 ) ) ;
#5939=B_SPLINE_CURVE_WITH_KNOTS ( 'NONE', 3,
 ( #50163, #18407, #25869, #2257 ),
 .UNSPECIFIED., .F., .F.,
 ( 4, 4 ),
 ( 0.000000000000000000, 0.002368422649471296423 ),
 .UNSPECIFIED. ) ;
#5960=( LENGTH_UNIT ( ) NAMED_UNIT ( * ) SI_UNIT ( .MILLI., .METRE. ) );
#5974=B_SPLINE_CURVE_WITH_KNOTS ( 'NONE', 3,
 ( #25220, #18009, #14155, #5710 ),
 .UNSPECIFIED., .F., .F.,
 ( 4, 4 ),
 ( 0.0002936521407493293328, 0.0006663369986113973614 ),
 .UNSPECIFIED. ) ;
#5976=CARTESIAN_POINT ( 'NONE',  ( 16.76006782980217125, -2.050259795448531541, 9.178419661560148768 ) ) ;
#5979=CARTESIAN_POINT ( 'NONE',  ( -27.31081730472607561, -41.96092862852123773, 3.199614146704519602 ) ) ;
#5986=CARTESIAN_POINT ( 'NONE',  ( 1.250000000000000222, 0.000000000000000000, -10.00000000000000000 ) ) ;
#6004=CARTESIAN_POINT ( 'NONE',  ( 48.98697415750967821, 11.03699497439252220, -8.016098858316205167 ) ) ;
#6007=VERTEX_POINT ( 'NONE', #42323 ) ;
#6016=DIRECTION ( 'NONE',  ( 1.000000000000000000, 0.000000000000000000, -0.000000000000000000 ) ) ;
#6022=CARTESIAN_POINT ( 'NONE',  ( -6.408332700304190332, -7.676800896350769676, 0.000000000000000000 ) ) ;
#6026=CARTESIAN_POINT ( 'NONE',  ( 0.3862712429686727678, 1.188820645368945605, 3.333333333333333481 ) ) ;
#6030=CARTESIAN_POINT ( 'NONE',  ( -37.27397286063865778, 4.111076158911805223, 7.697694107796192675 ) ) ;
#6035=CARTESIAN_POINT ( 'NONE',  ( -1.424725715586989239, 0.8249487629949916467, 9.927568724237804787 ) ) ;
#6042=ORIENTED_EDGE ( 'NONE', *, *, #7705, .F. ) ;
#6044=CARTESIAN_POINT ( 'NONE',  ( -30.12518629743573584, -14.70074613238887551, 1.847720168420772691 ) ) ;
#6046=CARTESIAN_POINT ( 'NONE',  ( 27.33593271309472073, -41.94268121623323964, -9.367992836599954742 ) ) ;
#6050=B_SPLINE_SURFACE_WITH_KNOTS ( 'NONE', 3, 3, ( 
 ( #5451, #21103, #44683, #45176 ),
 ( #33183, #21607, #21874, #9561 ),
 ( #25210, #9800, #25463, #40857 ),
 ( #5703, #21353, #37041, #48767 ) ),
 .UNSPECIFIED., .F., .F., .F.,
 ( 4, 4 ),
 ( 4, 4 ),
 ( 0.000000000000000000, 1.000000000000000000 ),
 ( 0.000000000000000000, 1.000000000000000000 ),
 .UNSPECIFIED. ) ;
#6075=CARTESIAN_POINT ( 'NONE',  ( -0.3862712429686809279, -1.188820645368943163, -10.00000000000000000 ) ) ;
#6078=ADVANCED_FACE ( 'NONE', ( #16390 ), #22347, .T. ) ;
#6081=CARTESIAN_POINT ( 'NONE',  ( -36.32827987961121607, 9.445964435369075929, 3.209567239418972928 ) ) ;
#6083=ADVANCED_FACE ( 'NONE', ( #27694 ), #34255, .T. ) ;
#6084=CARTESIAN_POINT ( 'NONE',  ( 2.052560157877110658, -0.2040521727611157299, 9.891980816076525684 ) ) ;
#6085=CARTESIAN_POINT ( 'NONE',  ( 0.8285222815141930486, 1.889008401827334094, 9.886433018048068178 ) ) ;
#6097=CARTESIAN_POINT ( 'NONE',  ( 0.000000000000000000, 0.000000000000000000, 0.000000000000000000 ) ) ;
#6105=AXIS2_PLACEMENT_3D ( 'NONE', #16237, #24449, #36257 ) ;
#6114=EDGE_CURVE ( 'NONE', #31257, #49939, #4078, .T. ) ;
#6121=ORIENTED_EDGE ( 'NONE', *, *, #25589, .F. ) ;
#6143=CARTESIAN_POINT ( 'NONE',  ( 21.61731705588930907, 25.43568671410602278, -9.367992836599954742 ) ) ;
#6147=CARTESIAN_POINT ( 'NONE',  ( 31.44259251615245887, 38.95901822126168668, -9.367992836599954742 ) ) ;
#6154=CARTESIAN_POINT ( 'NONE',  ( -28.96803024440907137, -18.11533787072017176, 7.455576670931136185 ) ) ;
#6155=B_SPLINE_CURVE_WITH_KNOTS ( 'NONE', 3,
 ( #34668, #22087, #30055, #45909 ),
 .UNSPECIFIED., .F., .F.,
 ( 4, 4 ),
 ( 0.7998230999345287140, 0.9869080488566183140 ),
 .UNSPECIFIED. ) ;
#6167=CARTESIAN_POINT ( 'NONE',  ( -14.86945752723352498, -7.944783388878907004, 2.590526750877053086 ) ) ;
#6182=ORIENTED_EDGE ( 'NONE', *, *, #1354, .F. ) ;
#6230=CARTESIAN_POINT ( 'NONE',  ( -13.92102703536724384, -30.85732372859812500, 8.356839323120299312 ) ) ;
#6258=CARTESIAN_POINT ( 'NONE',  ( 33.64889274059390090, -3.704246042440748621, 8.356839323120299312 ) ) ;
#6261=ORIENTED_EDGE ( 'NONE', *, *, #5765, .T. ) ;
#6263=CARTESIAN_POINT ( 'NONE',  ( -0.3862712429686977478, 1.188820645368937390, -3.333333333333333481 ) ) ;
#6268=B_SPLINE_CURVE_WITH_KNOTS ( 'NONE', 3,
 ( #22816, #14609, #30030, #3309 ),
 .UNSPECIFIED., .F., .F.,
 ( 4, 4 ),
 ( 0.8097120833243680593, 0.9322955464061821740 ),
 .UNSPECIFIED. ) ;
#6275=DIRECTION ( 'NONE',  ( -0.000000000000000000, 0.000000000000000000, -1.000000000000000000 ) ) ;
#6276=EDGE_CURVE ( 'NONE', #24192, #31155, #35261, .T. ) ;
#6277=VERTEX_POINT ( 'NONE', #41506 ) ;
#6286=B_SPLINE_CURVE_WITH_KNOTS ( 'NONE', 3,
 ( #46170, #3356, #11063, #26723 ),
 .UNSPECIFIED., .F., .F.,
 ( 4, 4 ),
 ( 2.278501876322824808E-17, 0.0004301978946275286349 ),
 .UNSPECIFIED. ) ;
#6299=DIRECTION ( 'NONE',  ( -0.000000000000000000, -0.000000000000000000, 1.000000000000000000 ) ) ;
#6309=VERTEX_POINT ( 'NONE', #29704 ) ;
#6310=CARTESIAN_POINT ( 'NONE',  ( 6.604186672497970534, -1.848482776016330043, 9.753789706659947711 ) ) ;
#6311=CARTESIAN_POINT ( 'NONE',  ( 0.3862712429686894766, -1.188820645368940276, 3.333333333333333481 ) ) ;
#6312=CARTESIAN_POINT ( 'NONE',  ( -12.78770032058971395, -31.68259716188267916, 7.455576670931136185 ) ) ;
#6321=CARTESIAN_POINT ( 'NONE',  ( 7.576114424932982594, -50.00000000000000711, 7.906207997025717304 ) ) ;
#6323=ORIENTED_EDGE ( 'NONE', *, *, #35100, .T. ) ;
#6370=CARTESIAN_POINT ( 'NONE',  ( -34.08355720199904226, 2.371364769369340042, 7.455576670931136185 ) ) ;
#6374=CARTESIAN_POINT ( 'NONE',  ( 3.951902928218917754, 0.4322042478607662219, 3.247139300358769631 ) ) ;
#6382=EDGE_LOOP ( 'NONE', ( #10105, #18619, #25690 ) ) ;
#6394=CARTESIAN_POINT ( 'NONE',  ( 1.035950918207909632, 33.23661552194049307, -2.408242355805840784 ) ) ;
#6397=CARTESIAN_POINT ( 'NONE',  ( 25.40454589245968364, 27.58367357691700406, -8.192531242611265085 ) ) ;
#6398=CARTESIAN_POINT ( 'NONE',  ( -1.011271242968677875, -0.7347315653656004697, -3.333333333333333481 ) ) ;
#6402=ORIENTED_EDGE ( 'NONE', *, *, #18737, .T. ) ;
#6406=EDGE_CURVE ( 'NONE', #3893, #16542, #2785, .T. ) ;
#6411=CARTESIAN_POINT ( 'NONE',  ( 28.05568344207340203, 30.90646677863635716, -8.080361901872242569 ) ) ;
#6413=EDGE_CURVE ( 'NONE', #33857, #20200, #47080, .T. ) ;
#6419=B_SPLINE_CURVE_WITH_KNOTS ( 'NONE', 3,
 ( #16994, #1100, #13384, #47741 ),
 .UNSPECIFIED., .F., .F.,
 ( 4, 4 ),
 ( 0.001152428489661398063, 0.001623376834731057655 ),
 .UNSPECIFIED. ) ;
#6429=EDGE_CURVE ( 'NONE', #39174, #10463, #40159, .T. ) ;
#6430=CARTESIAN_POINT ( 'NONE',  ( -23.83799721022572982, 28.99517291086380411, 3.209567239418972040 ) ) ;
#6431=EDGE_CURVE ( 'NONE', #323, #12448, #34527, .T. ) ;
#6432=EDGE_LOOP ( 'NONE', ( #13371, #27149, #26578, #334, #24816, #23393, #40631, #49460, #28788, #30289, #4792, #3098 ) ) ;
#6435=CARTESIAN_POINT ( 'NONE',  ( -24.47767542868268364, 23.18653802921800278, 8.807470649214879543 ) ) ;
#6442=CARTESIAN_POINT ( 'NONE',  ( 36.63544619771723632, 20.34968343020639381, 7.544061037322998153 ) ) ;
#6448=FACE_OUTER_BOUND ( 'NONE', #48613, .T. ) ;
#6456=CARTESIAN_POINT ( 'NONE',  ( 30.21887974406487487, -14.69854701517530060, -8.016098858316199838 ) ) ;
#6474=B_SPLINE_SURFACE_WITH_KNOTS ( 'NONE', 3, 3, ( 
 ( #35743, #31632, #12604, #7770 ),
 ( #46711, #11863, #35224, #36237 ),
 ( #31880, #1074, #28272, #39321 ),
 ( #27262, #4414, #8268, #42887 ) ),
 .UNSPECIFIED., .F., .F., .F.,
 ( 4, 4 ),
 ( 4, 4 ),
 ( 0.000000000000000000, 1.000000000000000000 ),
 ( 0.000000000000000000, 1.000000000000000000 ),
 .UNSPECIFIED. ) ;
#6476=CARTESIAN_POINT ( 'NONE',  ( 0.9989200098981507736, 1.123829893718967687, 9.927319414211233095 ) ) ;
#6477=EDGE_CURVE ( 'NONE', #12217, #38289, #12228, .T. ) ;
#6478=CARTESIAN_POINT ( 'NONE',  ( -0.1287570809895576818, -0.3962735484563154609, 10.00000000000000000 ) ) ;
#6484=EDGE_CURVE ( 'NONE', #36910, #30921, #39531, .T. ) ;
#6486=ORIENTED_EDGE ( 'NONE', *, *, #43350, .F. ) ;
#6487=AXIS2_PLACEMENT_3D ( 'NONE', #3897, #47218, #19798 ) ;
#6489=EDGE_CURVE ( 'NONE', #40379, #30326, #41958, .T. ) ;
#6498=CARTESIAN_POINT ( 'NONE',  ( -28.05568344207363296, -30.90646677863614045, -8.080361901872242569 ) ) ;
#6503=CARTESIAN_POINT ( 'NONE',  ( -0.2773062244624664441, 1.251557370488897813, 9.948547179989621014 ) ) ;
#6507=CARTESIAN_POINT ( 'NONE',  ( -0.9989200098981521059, -1.123829893718962802, 9.927319414211225990 ) ) ;
#6509=B_SPLINE_CURVE_WITH_KNOTS ( 'NONE', 3,
 ( #28239, #12081, #27726, #16429 ),
 .UNSPECIFIED., .F., .F.,
 ( 4, 4 ),
 ( 0.000000000000000000, 0.002458791966311101550 ),
 .UNSPECIFIED. ) ;
#6512=B_SPLINE_CURVE_WITH_KNOTS ( 'NONE', 3,
 ( #8907, #1226, #37585, #14714 ),
 .UNSPECIFIED., .F., .F.,
 ( 4, 4 ),
 ( 0.7998230999345288250, 0.9869080488566185361 ),
 .UNSPECIFIED. ) ;
#6515=CARTESIAN_POINT ( 'NONE',  ( -1.104477492316108256, -0.6506302558160915739, 9.957892297621011579 ) ) ;
#6517=EDGE_LOOP ( 'NONE', ( #2795, #32012, #44075 ) ) ;
#6531=EDGE_CURVE ( 'NONE', #25811, #35155, #15658, .T. ) ;
#6533=ORIENTED_EDGE ( 'NONE', *, *, #10801, .T. ) ;
#6551=ORIENTED_EDGE ( 'NONE', *, *, #5031, .F. ) ;
#6552=CARTESIAN_POINT ( 'NONE',  ( 22.75063655912441973, 24.61040335498486442, -8.466730184410787174 ) ) ;
#6553=CARTESIAN_POINT ( 'NONE',  ( -32.43949840348904701, -7.871562655726274116, -9.367992836599954742 ) ) ;
#6570=B_SPLINE_CURVE_WITH_KNOTS ( 'NONE', 3,
 ( #31205, #18860, #23227, #11689 ),
 .UNSPECIFIED., .F., .F.,
 ( 4, 4 ),
 ( 0.0002936521407521901629, 0.0006663369986142733160 ),
 .UNSPECIFIED. ) ;
#6572=EDGE_CURVE ( 'NONE', #24636, #4376, #47472, .T. ) ;
#6577=ORIENTED_EDGE ( 'NONE', *, *, #46007, .F. ) ;
#6581=VERTEX_POINT ( 'NONE', #16588 ) ;
#6584=DIRECTION ( 'NONE',  ( -0.000000000000000000, 0.000000000000000000, -1.000000000000000000 ) ) ;
#6589=CARTESIAN_POINT ( 'NONE',  ( 1.655785408456140084, 0.7536129375913136474, 9.903764339332061795 ) ) ;
#6591=CARTESIAN_POINT ( 'NONE',  ( -2.945500763482279627, -16.64098165802040086, -9.008049429158100807 ) ) ;
#6596=CARTESIAN_POINT ( 'NONE',  ( -36.01122090644304308, -10.59066248886169070, -2.490396854064194532 ) ) ;
#6602=EDGE_CURVE ( 'NONE', #22111, #11547, #7718, .T. ) ;
#6605=CARTESIAN_POINT ( 'NONE',  ( -29.39982726364978660, -16.78152490921149109, 8.356839323120299312 ) ) ;
#6609=B_SPLINE_CURVE_WITH_KNOTS ( 'NONE', 3,
 ( #9277, #31884, #13369, #47480 ),
 .UNSPECIFIED., .F., .F.,
 ( 4, 4 ),
 ( 5.641302087946644680E-05, 0.0003272669002642551728 ),
 .UNSPECIFIED. ) ;
#6616=ORIENTED_EDGE ( 'NONE', *, *, #8597, .F. ) ;
#6618=EDGE_LOOP ( 'NONE', ( #14587, #14269, #12096 ) ) ;
#6623=CARTESIAN_POINT ( 'NONE',  ( -48.99656738986512039, 11.00747004110376182, 1.847720168420772691 ) ) ;
#6626=CARTESIAN_POINT ( 'NONE',  ( 29.38926261462312439, 40.45084971874776159, 0.000000000000000000 ) ) ;
#6627=B_SPLINE_CURVE_WITH_KNOTS ( 'NONE', 3,
 ( #11920, #12658, #19853, #31427 ),
 .UNSPECIFIED., .F., .F.,
 ( 4, 4 ),
 ( 0.7998230999345287140, 0.9869080488566183140 ),
 .UNSPECIFIED. ) ;
#6632=AXIS2_PLACEMENT_3D ( 'NONE', #26765, #42396, #27013 ) ;
#6635=ORIENTED_EDGE ( 'NONE', *, *, #10833, .T. ) ;
#6646=FACE_OUTER_BOUND ( 'NONE', #1275, .T. ) ;
#6650=CARTESIAN_POINT ( 'NONE',  ( 1.073226156958098532, 0.6788500330460306431, 9.975314328424618182 ) ) ;
#6654=CARTESIAN_POINT ( 'NONE',  ( 8.470991794550016607, 5.371644396275345734, 9.390253821402620105 ) ) ;
#6659=CARTESIAN_POINT ( 'NONE',  ( -40.76831105797795374, -21.94948152812802178, 7.455576670931137073 ) ) ;
#6667=CARTESIAN_POINT ( 'NONE',  ( -3.996390545799824334, 16.57371371864897469, 8.953103998512858652 ) ) ;
#6680=ORIENTED_EDGE ( 'NONE', *, *, #18204, .F. ) ;
#6683=CARTESIAN_POINT ( 'NONE',  ( -13.59579750444763668, 10.60877755095910935, 8.727788335465566760 ) ) ;
#6688=EDGE_CURVE ( 'NONE', #16962, #38289, #43772, .T. ) ;
#6693=ADVANCED_FACE ( 'NONE', ( #40949 ), #48912, .T. ) ;
#6695=CARTESIAN_POINT ( 'NONE',  ( 33.57695195286775913, 16.69845195084893064, 8.914903342594561408 ) ) ;
#6697=VERTEX_POINT ( 'NONE', #18585 ) ;
#6698=CARTESIAN_POINT ( 'NONE',  ( -0.9494396179258391966, 9.954826186926261755, 9.646707543097345905 ) ) ;
#6703=CARTESIAN_POINT ( 'NONE',  ( 0.000000000000000000, 0.000000000000000000, 10.00000000000000000 ) ) ;
#6704=CARTESIAN_POINT ( 'NONE',  ( 34.38425513258721367, -36.82177522737821107, 8.807470649214879543 ) ) ;
#6718=CARTESIAN_POINT ( 'NONE',  ( -22.69295089195507487, -45.31600496604688999, 7.455576670931136185 ) ) ;
#6722=CARTESIAN_POINT ( 'NONE',  ( -1.437255894074058515, 3.713052624461494755, 6.606856988583542645E-16 ) ) ;
#6725=CARTESIAN_POINT ( 'NONE',  ( 1.025617443043004062, 1.003000432358625238, 9.950105812514292936 ) ) ;
#6744=FACE_OUTER_BOUND ( 'NONE', #37353, .T. ) ;
#6750=CARTESIAN_POINT ( 'NONE',  ( -4.190612935961002705, -4.237468719480293800, 5.692061405548898279E-16 ) ) ;
#6769=ORIENTED_EDGE ( 'NONE', *, *, #36702, .T. ) ;
#6776=CARTESIAN_POINT ( 'NONE',  ( 0.8510287611193416701, 1.787020300839067932, 9.897807938190497978 ) ) ;
#6782=CARTESIAN_POINT ( 'NONE',  ( -34.38425513258695077, 36.82177522737848108, 8.807470649214879543 ) ) ;
#6784=FACE_OUTER_BOUND ( 'NONE', #19902, .T. ) ;
#6791=B_SPLINE_SURFACE_WITH_KNOTS ( 'NONE', 3, 3, ( 
 ( #21183, #17838, #29147, #40946 ),
 ( #36873, #17084, #29895, #9389 ),
 ( #45516, #25542, #14231, #33263 ),
 ( #25048, #33006, #5788, #10400 ) ),
 .UNSPECIFIED., .F., .F., .F.,
 ( 4, 4 ),
 ( 4, 4 ),
 ( 0.000000000000000000, 1.000000000000000000 ),
 ( 0.000000000000000000, 1.000000000000000000 ),
 .UNSPECIFIED. ) ;
#6793=CARTESIAN_POINT ( 'NONE',  ( 1.011271242968683648, 0.7347315653655930312, 3.333333333333333481 ) ) ;
#6803=CARTESIAN_POINT ( 'NONE',  ( 30.25247992116058526, -39.82368563463805344, -3.760136334089591248 ) ) ;
#6805=CARTESIAN_POINT ( 'NONE',  ( -5.888214538810513154, -16.20866436362413410, 8.727788335465566760 ) ) ;
#6811=CARTESIAN_POINT ( 'NONE',  ( 1.250000000000000222, 0.000000000000000000, 10.00000000000000000 ) ) ;
#6818=CARTESIAN_POINT ( 'NONE',  ( 3.996390545799824334, -16.57371371864897469, 8.953103998512858652 ) ) ;
#6821=ORIENTED_EDGE ( 'NONE', *, *, #12059, .T. ) ;
#6829=CARTESIAN_POINT ( 'NONE',  ( 25.60949810002064098, 43.19700938445193827, 1.847720168420772691 ) ) ;
#6840=EDGE_CURVE ( 'NONE', #18355, #18198, #23726, .T. ) ;
#6846=CARTESIAN_POINT ( 'NONE',  ( -1.290940757015139662, 0.08848829412237076142, 9.947020512645400103 ) ) ;
#6855=CARTESIAN_POINT ( 'NONE',  ( -33.57695195286787282, -16.69845195084869616, 8.914903342594564961 ) ) ;
#6857=CARTESIAN_POINT ( 'NONE',  ( 33.08717642956893457, 5.870837526465158440, -8.016098858316205167 ) ) ;
#6860=CARTESIAN_POINT ( 'NONE',  ( -1.250000000000000222, 0.000000000000000000, 10.00000000000000000 ) ) ;
#6876=VERTEX_POINT ( 'NONE', #50098 ) ;
#6883=CARTESIAN_POINT ( 'NONE',  ( -0.3862712429686977478, 1.188820645368937390, 10.00000000000000000 ) ) ;
#6888=DIRECTION ( 'NONE',  ( -0.4374820812098861866, 0.3178493372392685590, 0.8411784753765543243 ) ) ;
#6899=CARTESIAN_POINT ( 'NONE',  ( 1.250000000000000222, 0.000000000000000000, 10.00000000000000000 ) ) ;
#6902=B_SPLINE_SURFACE_WITH_KNOTS ( 'NONE', 3, 3, ( 
 ( #43430, #19829, #35774, #47250 ),
 ( #32151, #47744, #8806, #35507 ),
 ( #23941, #12634, #16499, #23693 ),
 ( #32403, #4699, #19574, #8300 ) ),
 .UNSPECIFIED., .F., .F., .F.,
 ( 4, 4 ),
 ( 4, 4 ),
 ( 0.000000000000000000, 1.000000000000000000 ),
 ( 0.000000000000000000, 1.000000000000000000 ),
 .UNSPECIFIED. ) ;
#6912=CARTESIAN_POINT ( 'NONE',  ( -7.359817328027146388, -15.16751262232800102, 2.590526750877053086 ) ) ;
#6913=B_SPLINE_CURVE_WITH_KNOTS ( 'NONE', 3,
 ( #3113, #43316, #31549, #38041 ),
 .UNSPECIFIED., .F., .F.,
 ( 4, 4 ),
 ( 3.806883176665572679E-16, 0.009762429722931321996 ),
 .UNSPECIFIED. ) ;
#6916=CARTESIAN_POINT ( 'NONE',  ( -1.011271242968677875, -0.7347315653656004697, -3.333333333333333481 ) ) ;
#6921=CARTESIAN_POINT ( 'NONE',  ( 1.448406091252584238, -0.9360325558322883932, 9.928159647716132241 ) ) ;
#6932=CARTESIAN_POINT ( 'NONE',  ( -6.174150299305392053, 50.00000000000000711, 8.807470649214879543 ) ) ;
#6934=CARTESIAN_POINT ( 'NONE',  ( 1.275927284277173834, -0.1224368140627448004, 9.976582533991679824 ) ) ;
#6948=ORIENTED_EDGE ( 'NONE', *, *, #27087, .F. ) ;
#6951=CARTESIAN_POINT ( 'NONE',  ( -0.6677345994471270973, 1.504830332936299975, 9.927568724237746167 ) ) ;
#6957=CARTESIAN_POINT ( 'NONE',  ( 0.8155877869298099325, 0.9072449372238458043, 9.963925895597341764 ) ) ;
#6967=CARTESIAN_POINT ( 'NONE',  ( -23.26005729352344176, -44.90397804740339183, 7.906207997025717304 ) ) ;
#6968=CARTESIAN_POINT ( 'NONE',  ( -0.3370904143228943828, -0.2449105217885308716, 10.00000000000000000 ) ) ;
#6969=CARTESIAN_POINT ( 'NONE',  ( 36.08557433729230723, -35.58569447144768105, 7.455576670931136185 ) ) ;
#6984=CARTESIAN_POINT ( 'NONE',  ( -17.23491422248386584, 0.5912720620001978844, 8.727788335465566760 ) ) ;
#6986=EDGE_CURVE ( 'NONE', #49939, #4452, #900, .T. ) ;
#6991=CARTESIAN_POINT ( 'NONE',  ( 13.35436367797824353, 31.26996044524050333, 7.906207997025717304 ) ) ;
#6994=CARTESIAN_POINT ( 'NONE',  ( 1.288422560825904783, -0.1812466941682506494, 9.986087673579199020 ) ) ;
#6999=EDGE_LOOP ( 'NONE', ( #43685, #44081, #35669 ) ) ;
#7000=CARTESIAN_POINT ( 'NONE',  ( -1.173396789973005783, -0.3425192899591036344, 9.969517326150320713 ) ) ;
#7002=CARTESIAN_POINT ( 'NONE',  ( 31.28234235046230793, 11.28615439405779064, -3.760136334089591248 ) ) ;
#7008=CARTESIAN_POINT ( 'NONE',  ( 0.4266413953668419246, 1.250184266969606162, 9.943883492372851407 ) ) ;
#7009=B_SPLINE_CURVE_WITH_KNOTS ( 'NONE', 3,
 ( #15795, #16996, #46798, #35324 ),
 .UNSPECIFIED., .F., .F.,
 ( 4, 4 ),
 ( 4.165368725351569974E-18, 0.0004170521429101314869 ),
 .UNSPECIFIED. ) ;
#7028=CARTESIAN_POINT ( 'NONE',  ( 4.672045878990125800, -33.19353511768168374, 1.847720168420772691 ) ) ;
#7037=CARTESIAN_POINT ( 'NONE',  ( -36.76598589393961447, -7.383243274241610088, -8.192531242611266862 ) ) ;
#7038=ORIENTED_EDGE ( 'NONE', *, *, #10197, .F. ) ;
#7044=CARTESIAN_POINT ( 'NONE',  ( -36.08557433729205144, 35.58569447144795816, 7.455576670931136185 ) ) ;
#7046=CARTESIAN_POINT ( 'NONE',  ( -46.76852358249002606, 17.86468378716741512, -9.367992836599954742 ) ) ;
#7051=CARTESIAN_POINT ( 'NONE',  ( 0.4830800013901592194, 1.200413232422924192, 9.947020512645421420 ) ) ;
#7053=CARTESIAN_POINT ( 'NONE',  ( -30.21887974406478250, 14.69854701517550666, -8.016098858316199838 ) ) ;
#7054=EDGE_CURVE ( 'NONE', #18098, #24636, #23525, .T. ) ;
#7058=CARTESIAN_POINT ( 'NONE',  ( -49.46074318306826001, 9.578883844007169301, 8.807470649214879543 ) ) ;
#7060=CARTESIAN_POINT ( 'NONE',  ( 0.3862712429686894766, -1.188820645368940276, 10.00000000000000000 ) ) ;
#7068=CARTESIAN_POINT ( 'NONE',  ( -22.69295089195507487, -45.31600496604688999, 7.455576670931136185 ) ) ;
#7092=CARTESIAN_POINT ( 'NONE',  ( 1.133908876584335257, 0.5183204401656757998, 9.981352469109932457 ) ) ;
#7116=CARTESIAN_POINT ( 'NONE',  ( 3.229232847726260403, -16.57333684275945629, 9.178419661560148768 ) ) ;
#7128=CARTESIAN_POINT ( 'NONE',  ( 0.6440276692615867216, 16.64212148744554298, -9.683996418299976483 ) ) ;
#7133=CARTESIAN_POINT ( 'NONE',  ( -7.749480817862350435, -14.85497772329513211, 9.403735324607438884 ) ) ;
#7135=ORIENTED_EDGE ( 'NONE', *, *, #24647, .F. ) ;
#7140=CARTESIAN_POINT ( 'NONE',  ( -17.23491422248386584, 0.5912720620001978844, 8.727788335465566760 ) ) ;
#7144=VERTEX_POINT ( 'NONE', #45199 ) ;
#7148=ORIENTED_EDGE ( 'NONE', *, *, #25295, .T. ) ;
#7149=CARTESIAN_POINT ( 'NONE',  ( 0.3862712429686815385, 1.188820645368943385, 9.972675548442461846 ) ) ;
#7157=ORIENTED_EDGE ( 'NONE', *, *, #45119, .F. ) ;
#7167=LINE ( 'NONE', #18694, #25939 ) ;
#7168=CARTESIAN_POINT ( 'NONE',  ( -10.30302290646040575, -13.08520913973572419, -9.683996418299976483 ) ) ;
#7171=CARTESIAN_POINT ( 'NONE',  ( 1.228394325311184421, -1.341866297401743235, 9.903764339332088440 ) ) ;
#7172=ADVANCED_FACE ( 'NONE', ( #10584 ), #45254, .T. ) ;
#7176=ORIENTED_EDGE ( 'NONE', *, *, #48271, .T. ) ;
#7178=CARTESIAN_POINT ( 'NONE',  ( -0.3862712429686889770, 1.188820645368940720, 9.972675548442463622 ) ) ;
#7180=CARTESIAN_POINT ( 'NONE',  ( 0.3862712429686727678, 1.188820645368945605, -3.333333333333333481 ) ) ;
#7191=FACE_OUTER_BOUND ( 'NONE', #24159, .T. ) ;
#7195=ORIENTED_EDGE ( 'NONE', *, *, #31485, .F. ) ;
#7207=B_SPLINE_CURVE_WITH_KNOTS ( 'NONE', 3,
 ( #1374, #39615, #16009, #12399 ),
 .UNSPECIFIED., .F., .F.,
 ( 4, 4 ),
 ( 3.388966592816271738E-16, 0.009782300387714822770 ),
 .UNSPECIFIED. ) ;
#7209=ORIENTED_EDGE ( 'NONE', *, *, #13339, .F. ) ;
#7216=B_SPLINE_SURFACE_WITH_KNOTS ( 'NONE', 3, 3, ( 
 ( #24822, #40475, #44793, #48116 ),
 ( #5311, #48369, #35880, #12999 ),
 ( #28916, #13508, #29178, #20211 ),
 ( #4795, #9666, #16359, #39979 ) ),
 .UNSPECIFIED., .F., .F., .F.,
 ( 4, 4 ),
 ( 4, 4 ),
 ( 0.000000000000000000, 1.000000000000000000 ),
 ( 0.000000000000000000, 1.000000000000000000 ),
 .UNSPECIFIED. ) ;
#7224=CARTESIAN_POINT ( 'NONE',  ( 16.69947034530964913, -2.312583065866261389, 2.590526750877053086 ) ) ;
#7226=CARTESIAN_POINT ( 'NONE',  ( 27.33593271309472073, -41.94268121623323964, -9.367992836599954742 ) ) ;
#7236=FACE_OUTER_BOUND ( 'NONE', #16008, .T. ) ;
#7244=CARTESIAN_POINT ( 'NONE',  ( -1.011271242968693862, 0.7347315653655780432, 10.00000000000000000 ) ) ;
#7251=B_SPLINE_CURVE_WITH_KNOTS ( 'NONE', 3,
 ( #1802, #9490, #45370, #48695 ),
 .UNSPECIFIED., .F., .F.,
 ( 4, 4 ),
 ( 0.7491799374948677759, 1.000000000000000000 ),
 .UNSPECIFIED. ) ;
#7260=CARTESIAN_POINT ( 'NONE',  ( -0.8965959638259611841, -1.582931917743307215, 9.903764339332084887 ) ) ;
#7280=CARTESIAN_POINT ( 'NONE',  ( -0.2458784654125648617, -0.3384226744270785181, 9.992713367193012175 ) ) ;
#7286=ORIENTED_EDGE ( 'NONE', *, *, #17752, .F. ) ;
#7289=CARTESIAN_POINT ( 'NONE',  ( -0.3862712429686809279, -1.188820645368943163, 10.00000000000000000 ) ) ;
#7293=CARTESIAN_POINT ( 'NONE',  ( -0.7601424845489993531, 1.297311920617006065, 9.927319414211224213 ) ) ;
#7301=CARTESIAN_POINT ( 'NONE',  ( -45.64490844644706868, -21.32281559348764333, 8.807470649214879543 ) ) ;
#7321=CARTESIAN_POINT ( 'NONE',  ( -2.569099690548740877, 50.00000000000000711, 3.199614146704519602 ) ) ;
#7327=CARTESIAN_POINT ( 'NONE',  ( 0.4166666666666669072, 0.000000000000000000, 10.00000000000000000 ) ) ;
#7330=ORIENTED_EDGE ( 'NONE', *, *, #10247, .T. ) ;
#7356=DIRECTION ( 'NONE',  ( 0.000000000000000000, 0.000000000000000000, 1.000000000000000000 ) ) ;
#7370=ORIENTED_EDGE ( 'NONE', *, *, #41631, .F. ) ;
#7373=CARTESIAN_POINT ( 'NONE',  ( -2.569099690548740877, 33.19126772784019153, 3.199614146704519602 ) ) ;
#7374=B_SPLINE_CURVE_WITH_KNOTS ( 'NONE', 3,
 ( #43757, #932, #16575, #47824 ),
 .UNSPECIFIED., .F., .F.,
 ( 4, 4 ),
 ( 4.123618687664377220E-17, 0.0004072981213155453940 ),
 .UNSPECIFIED. ) ;
#7376=CARTESIAN_POINT ( 'NONE',  ( -0.8965959638259611841, -1.582931917743307215, 9.903764339332084887 ) ) ;
#7385=CARTESIAN_POINT ( 'NONE',  ( 2.945500763482280959, 16.64098165802040086, -9.008049429158102583 ) ) ;
#7388=CARTESIAN_POINT ( 'NONE',  ( -0.4426377647354682865, -1.666766018367764834, 9.928159647716134018 ) ) ;
#7391=CARTESIAN_POINT ( 'NONE',  ( -1.011271242968688533, 0.7347315653655859258, 3.333333333333333481 ) ) ;
#7395=CARTESIAN_POINT ( 'NONE',  ( 0.9989200098981507736, 1.123829893718967687, 9.927319414211233095 ) ) ;
#7400=EDGE_CURVE ( 'NONE', #2423, #21356, #1532, .T. ) ;
#7401=CARTESIAN_POINT ( 'NONE',  ( 28.96803024440893992, 18.11533787072037072, 7.455576670931136185 ) ) ;
#7411=CARTESIAN_POINT ( 'NONE',  ( -3.525518877594380207, 1.771455644630627102, 6.494306115487987086 ) ) ;
#7414=ORIENTED_EDGE ( 'NONE', *, *, #10312, .T. ) ;
#7422=CARTESIAN_POINT ( 'NONE',  ( -1.158497635116737312, 16.61944452314319420, -3.546734833711462365 ) ) ;
#7425=CARTESIAN_POINT ( 'NONE',  ( -6.875132362119187768, 33.14667368551891258, 8.356839323120299312 ) ) ;
#7430=CARTESIAN_POINT ( 'NONE',  ( 0.02998614097967981437, 1.600097392939184182, 9.919954280166516369 ) ) ;
#7434=ORIENTED_EDGE ( 'NONE', *, *, #7955, .T. ) ;
#7440=ORIENTED_EDGE ( 'NONE', *, *, #47570, .T. ) ;
#7441=CARTESIAN_POINT ( 'NONE',  ( -20.37409433808010562, -26.28007012093468475, -2.408242355805840784 ) ) ;
#7442=CARTESIAN_POINT ( 'NONE',  ( -25.40454589245989325, -27.58367357691681931, -8.192531242611266862 ) ) ;
#7450=CARTESIAN_POINT ( 'NONE',  ( -0.1287570809895576818, -0.3962735484563154609, 10.00000000000000000 ) ) ;
#7459=ORIENTED_EDGE ( 'NONE', *, *, #16580, .T. ) ;
#7462=ORIENTED_EDGE ( 'NONE', *, *, #34779, .F. ) ;
#7471=EDGE_CURVE ( 'NONE', #12617, #3137, #34517, .T. ) ;
#7490=CARTESIAN_POINT ( 'NONE',  ( 17.51065725283126895, -28.41934970907778890, -9.367992836599954742 ) ) ;
#7491=ORIENTED_EDGE ( 'NONE', *, *, #8703, .F. ) ;
#7503=CARTESIAN_POINT ( 'NONE',  ( 34.08406891383362591, -15.63733501198463038, -8.192531242611266862 ) ) ;
#7506=CARTESIAN_POINT ( 'NONE',  ( -1.275927284277175167, 0.1224368140627496299, 9.976582533991679824 ) ) ;
#7509=CARTESIAN_POINT ( 'NONE',  ( -14.48769039275601145, -30.44468701195584970, 8.807470649214879543 ) ) ;
#7518=CARTESIAN_POINT ( 'NONE',  ( 49.46074318306830975, -9.578883844006833570, 8.807470649214879543 ) ) ;
#7534=CARTESIAN_POINT ( 'NONE',  ( -21.61731705588949737, -25.43568671410585935, -9.367992836599954742 ) ) ;
#7541=ORIENTED_EDGE ( 'NONE', *, *, #41067, .T. ) ;
#7546=CARTESIAN_POINT ( 'NONE',  ( -21.17460298198278323, -30.99364813079819214, -3.721387749823083624 ) ) ;
#7553=CARTESIAN_POINT ( 'NONE',  ( 7.749480817862238524, 14.85497772329518895, 9.403735324607438884 ) ) ;
#7558=CARTESIAN_POINT ( 'NONE',  ( -0.9162543521530380763, 1.312131394983868660, 9.919954280166516369 ) ) ;
#7563=B_SPLINE_CURVE_WITH_KNOTS ( 'NONE', 3,
 ( #25337, #6846, #29194, #48884 ),
 .UNSPECIFIED., .F., .F.,
 ( 4, 4 ),
 ( 0.0006669682284780769407, 0.0007799402130932229886 ),
 .UNSPECIFIED. ) ;
#7565=CARTESIAN_POINT ( 'NONE',  ( -2.892039187329358718, 1.502206308778131882, 9.799352050262546854 ) ) ;
#7569=CARTESIAN_POINT ( 'NONE',  ( -50.11058929355264979, 7.578863168071929834, 7.455576670931136185 ) ) ;
#7579=CARTESIAN_POINT ( 'NONE',  ( 0.4166666666666664631, 0.000000000000000000, 10.00000000000000000 ) ) ;
#7582=ORIENTED_EDGE ( 'NONE', *, *, #11419, .F. ) ;
#7587=ORIENTED_EDGE ( 'NONE', *, *, #19618, .T. ) ;
#7597=CARTESIAN_POINT ( 'NONE',  ( 15.42815683172628738, 34.17926237904582365, 7.697694107796191787 ) ) ;
#7608=LINE ( 'NONE', #35335, #49508 ) ;
#7611=CARTESIAN_POINT ( 'NONE',  ( 24.39427009665984869, 44.07992421011656603, 8.807470649214879543 ) ) ;
#7619=CARTESIAN_POINT ( 'NONE',  ( 0.09523839817332763191, 1.466467394239034050, 9.958264684458713489 ) ) ;
#7622=CARTESIAN_POINT ( 'NONE',  ( 15.62858259096121216, -5.755205073598614440, -9.683996418299976483 ) ) ;
#7625=CARTESIAN_POINT ( 'NONE',  ( 6.906133693021909714, 3.984196388068609096, -1.219727444046192488E-16 ) ) ;
#7642=B_SPLINE_SURFACE_WITH_KNOTS ( 'NONE', 3, 3, ( 
 ( #28161, #24320, #41464, #33520 ),
 ( #17853, #49853, #14512, #29659 ),
 ( #10660, #2461, #30164, #2217 ),
 ( #2954, #14254, #21447, #21963 ) ),
 .UNSPECIFIED., .F., .F., .F.,
 ( 4, 4 ),
 ( 4, 4 ),
 ( 0.000000000000000000, 1.000000000000000000 ),
 ( 0.000000000000000000, 1.000000000000000000 ),
 .UNSPECIFIED. ) ;
#7649=CARTESIAN_POINT ( 'NONE',  ( 0.3905129037392675584, -2.126717070043174562, 9.885585981620943485 ) ) ;
#7669=CARTESIAN_POINT ( 'NONE',  ( -1.249999999999999778, 0.000000000000000000, 3.333333333333333481 ) ) ;
#7673=CARTESIAN_POINT ( 'NONE',  ( 1.133908876584335257, 0.5183204401656757998, 9.981352469109932457 ) ) ;
#7678=CARTESIAN_POINT ( 'NONE',  ( 0.1475726264153646716, 1.496347932843221429, 9.927319414211224213 ) ) ;
#7693=CARTESIAN_POINT ( 'NONE',  ( 16.02661358026014327, 4.530191650547718218, -9.683996418299976483 ) ) ;
#7699=CARTESIAN_POINT ( 'NONE',  ( 0.1475726264153646716, 1.496347932843221429, 9.927319414211224213 ) ) ;
#7705=EDGE_CURVE ( 'NONE', #19380, #13001, #12478, .T. ) ;
#7710=B_SPLINE_CURVE_WITH_KNOTS ( 'NONE', 3,
 ( #46090, #7649, #42286, #23281 ),
 .UNSPECIFIED., .F., .F.,
 ( 4, 4 ),
 ( 0.9688112071879401155, 0.9724175925769218409 ),
 .UNSPECIFIED. ) ;
#7718=B_SPLINE_CURVE_WITH_KNOTS ( 'NONE', 3,
 ( #36876, #949, #1696, #20685 ),
 .UNSPECIFIED., .F., .F.,
 ( 4, 4 ),
 ( 0.000000000000000000, 0.2637263876330694368 ),
 .UNSPECIFIED. ) ;
#7723=ORIENTED_EDGE ( 'NONE', *, *, #45517, .T. ) ;
#7732=CARTESIAN_POINT ( 'NONE',  ( 24.34206871062956168, 28.53454467304761621, -9.011255500499641968 ) ) ;
#7741=CARTESIAN_POINT ( 'NONE',  ( -33.57695195286787282, -16.69845195084869616, 8.914903342594564961 ) ) ;
#7758=EDGE_CURVE ( 'NONE', #17745, #18968, #36350, .T. ) ;
#7766=CARTESIAN_POINT ( 'NONE',  ( 6.508636631827673824, 15.75743548351451295, 8.953103998512858652 ) ) ;
#7768=B_SPLINE_CURVE_WITH_KNOTS ( 'NONE', 3,
 ( #9424, #36138, #28672, #25331 ),
 .UNSPECIFIED., .F., .F.,
 ( 4, 4 ),
 ( 0.000000000000000000, 2.804146970187276501E-05 ),
 .UNSPECIFIED. ) ;
#7770=CARTESIAN_POINT ( 'NONE',  ( -1.011271242968693862, 0.7347315653655780432, 10.00000000000000000 ) ) ;
#7772=CARTESIAN_POINT ( 'NONE',  ( 10.92344319659198248, 12.63397777816698486, -9.458680755252684591 ) ) ;
#7775=EDGE_CURVE ( 'NONE', #449, #16032, #13049, .T. ) ;
#7794=CARTESIAN_POINT ( 'NONE',  ( -7.359817328027146388, -15.16751262232800102, 2.590526750877053086 ) ) ;
#7796=CARTESIAN_POINT ( 'NONE',  ( -1.104609456715841986, -0.6504863887005195577, 9.948547179989617462 ) ) ;
#7813=DIRECTION ( 'NONE',  ( 0.000000000000000000, 0.000000000000000000, 1.000000000000000000 ) ) ;
#7826=CARTESIAN_POINT ( 'NONE',  ( -0.1287570809895602630, -0.3962735484563142396, 10.00000000000000000 ) ) ;
#7833=ADVANCED_FACE ( 'NONE', ( #25298 ), #41603, .T. ) ;
#7834=ORIENTED_EDGE ( 'NONE', *, *, #44301, .T. ) ;
#7835=CIRCLE ( 'NONE', #44671, 10.00000000000000000 ) ;
#7838=CARTESIAN_POINT ( 'NONE',  ( -31.44259251615275019, -38.95901822126145220, -9.367992836599954742 ) ) ;
#7850=CARTESIAN_POINT ( 'NONE',  ( -6.174150299305392053, 33.14591993373988998, 8.807470649214879543 ) ) ;
#7853=DIRECTION ( 'NONE',  ( 0.000000000000000000, -0.000000000000000000, -1.000000000000000000 ) ) ;
#7862=CARTESIAN_POINT ( 'NONE',  ( -0.6440276692615888310, -16.64212148744554298, -9.683996418299976483 ) ) ;
#7876=CARTESIAN_POINT ( 'NONE',  ( -0.2050626648094178439, 1.807624707194796843, 9.903764339332081335 ) ) ;
#7885=CARTESIAN_POINT ( 'NONE',  ( 16.02661358026014327, 4.530191650547719995, -9.683996418299976483 ) ) ;
#7887=AXIS2_PLACEMENT_3D ( 'NONE', #12328, #36209, #32352 ) ;
#7889=CARTESIAN_POINT ( 'NONE',  ( 9.260964247899973856, -13.84230907185609460, -9.683996418299976483 ) ) ;
#7890=CARTESIAN_POINT ( 'NONE',  ( -34.08355720199904226, 2.371364769369340042, 7.455576670931136185 ) ) ;
#7891=CARTESIAN_POINT ( 'NONE',  ( -0.9647729474495799762, -1.276880572101795286, 9.919954280166519922 ) ) ;
#7897=VERTEX_POINT ( 'NONE', #34020 ) ;
#7904=CARTESIAN_POINT ( 'NONE',  ( 0.6126904405382156416, 1.085824959725723016, 9.981352469109932457 ) ) ;
#7905=ORIENTED_EDGE ( 'NONE', *, *, #47152, .T. ) ;
#7907=CARTESIAN_POINT ( 'NONE',  ( -0.8433491450857070193, 0.9182416014173486740, 9.981352469109932457 ) ) ;
#7923=CARTESIAN_POINT ( 'NONE',  ( 26.18032376592674737, -21.95228666728361233, 7.455576670931136185 ) ) ;
#7925=B_SPLINE_CURVE_WITH_KNOTS ( 'NONE', 3,
 ( #1624, #5459, #1377, #20606 ),
 .UNSPECIFIED., .F., .F.,
 ( 4, 4 ),
 ( 0.0008016012850907545907, 0.006940113526765079831 ),
 .UNSPECIFIED. ) ;
#7930=CARTESIAN_POINT ( 'NONE',  ( -49.46074318306825290, 9.578883844007165749, 8.807470649214879543 ) ) ;
#7934=CARTESIAN_POINT ( 'NONE',  ( 0.000000000000000000, 0.000000000000000000, 0.000000000000000000 ) ) ;
#7935=DIRECTION ( 'NONE',  ( 0.1671032855531354722, -0.5142910309547729097, 0.8411784753765541023 ) ) ;
#7937=CARTESIAN_POINT ( 'NONE',  ( -1.045807400993774339, 0.6549210616167606691, 9.969907203203804968 ) ) ;
#7940=CARTESIAN_POINT ( 'NONE',  ( 1.148889881503678545, 0.6106841242174666506, 9.986087673579140400 ) ) ;
#7955=EDGE_CURVE ( 'NONE', #16183, #12977, #34177, .T. ) ;
#7975=EDGE_CURVE ( 'NONE', #17766, #23241, #21897, .T. ) ;
#7985=ADVANCED_FACE ( 'NONE', ( #2451 ), #45674, .T. ) ;
#7996=CARTESIAN_POINT ( 'NONE',  ( -1.782521105131510186, 0.3635605703594341209, 9.903764339332088440 ) ) ;
#7998=FACE_OUTER_BOUND ( 'NONE', #19370, .T. ) ;
#8002=ORIENTED_EDGE ( 'NONE', *, *, #45371, .T. ) ;
#8015=ORIENTED_EDGE ( 'NONE', *, *, #46886, .T. ) ;
#8025=B_SPLINE_CURVE_WITH_KNOTS ( 'NONE', 3,
 ( #43057, #7937, #31541, #47128 ),
 .UNSPECIFIED., .F., .F.,
 ( 4, 4 ),
 ( 0.000000000000000000, 0.0002610106747150578552 ),
 .UNSPECIFIED. ) ;
#8030=ORIENTED_EDGE ( 'NONE', *, *, #47446, .F. ) ;
#8032=CARTESIAN_POINT ( 'NONE',  ( 3.087186397306452612, 2.514307945609885131, -2.642742795433417058E-16 ) ) ;
#8059=CARTESIAN_POINT ( 'NONE',  ( 3.566525152641073504, -1.569997364302916809, 9.741991644047246268 ) ) ;
#8072=CARTESIAN_POINT ( 'NONE',  ( 4.763548243873389154, -16.57409059453848599, 8.727788335465566760 ) ) ;
#8076=B_SPLINE_SURFACE_WITH_KNOTS ( 'NONE', 3, 3, ( 
 ( #25750, #48036, #17034, #41136 ),
 ( #33458, #1648, #21381, #13685 ),
 ( #36569, #17289, #5483, #44956 ),
 ( #5233, #13926, #37069, #32962 ) ),
 .UNSPECIFIED., .F., .F., .F.,
 ( 4, 4 ),
 ( 4, 4 ),
 ( 0.000000000000000000, 1.000000000000000000 ),
 ( 0.000000000000000000, 1.000000000000000000 ),
 .UNSPECIFIED. ) ;
#8079=CARTESIAN_POINT ( 'NONE',  ( -16.52264463346130796, 2.779753662172870232, 9.403735324607438884 ) ) ;
#8081=CARTESIAN_POINT ( 'NONE',  ( -29.18392875402943432, -17.44843138996582965, 7.906207997025717304 ) ) ;
#8087=CARTESIAN_POINT ( 'NONE',  ( -10.30302290646040575, -13.08520913973572419, -9.683996418299976483 ) ) ;
#8106=CARTESIAN_POINT ( 'NONE',  ( 3.229232847726260403, -16.57333684275945629, 9.178419661560148768 ) ) ;
#8107=EDGE_CURVE ( 'NONE', #5904, #36298, #25241, .T. ) ;
#8109=CARTESIAN_POINT ( 'NONE',  ( -49.46074318306825290, 9.578883844007165749, 8.807470649214879543 ) ) ;
#8123=ADVANCED_FACE ( 'NONE', ( #898 ), #29719, .T. ) ;
#8128=CARTESIAN_POINT ( 'NONE',  ( 2.210477865340801706, 37.43479381012853224, -9.422646554964178023 ) ) ;
#8141=CARTESIAN_POINT ( 'NONE',  ( -0.9306598006161299619, -1.429916298923569862, 9.912102921405038458 ) ) ;
#8151=EDGE_LOOP ( 'NONE', ( #29381, #32027, #44052, #18604 ) ) ;
#8152=CARTESIAN_POINT ( 'NONE',  ( 15.57957361750251302, 5.755602074545510760, 3.266473740018926541 ) ) ;
#8163=ORIENTED_EDGE ( 'NONE', *, *, #21130, .F. ) ;
#8165=CARTESIAN_POINT ( 'NONE',  ( -21.85563210430627024, -40.58578877481918568, 8.807470649214879543 ) ) ;
#8170=LINE ( 'NONE', #19949, #43335 ) ;
#8173=ORIENTED_EDGE ( 'NONE', *, *, #5807, .F. ) ;
#8178=DIRECTION ( 'NONE',  ( 0.000000000000000000, 0.000000000000000000, -1.000000000000000000 ) ) ;
#8186=CARTESIAN_POINT ( 'NONE',  ( 1.424123654779712922, 0.3625862473308184009, 9.958264684458541183 ) ) ;
#8201=CARTESIAN_POINT ( 'NONE',  ( 0.8811857040074689840, 1.919576306124735510, 9.890170120223995553 ) ) ;
#8206=CARTESIAN_POINT ( 'NONE',  ( -0.9987333402973620489, -1.123935354445870338, 9.936141075690079205 ) ) ;
#8231=VERTEX_POINT ( 'NONE', #33710 ) ;
#8232=CARTESIAN_POINT ( 'NONE',  ( 1.637520033018233345, 0.1700351954323681691, 9.927568724237806563 ) ) ;
#8248=CARTESIAN_POINT ( 'NONE',  ( 5.505322767148756569, -37.09368438467003415, 8.914903342594564961 ) ) ;
#8249=CARTESIAN_POINT ( 'NONE',  ( -1.133908876584336367, -0.5183204401656656968, 9.981352469109934233 ) ) ;
#8250=CARTESIAN_POINT ( 'NONE',  ( -20.40054609052957701, 26.26366202847989229, -3.760136334089591248 ) ) ;
#8260=EDGE_CURVE ( 'NONE', #12550, #26328, #48195, .T. ) ;
#8268=CARTESIAN_POINT ( 'NONE',  ( 10.30302290646030627, 13.08520913973580058, -9.683996418299976483 ) ) ;
#8270=EDGE_CURVE ( 'NONE', #40331, #44892, #49793, .T. ) ;
#8291=PLANE ( 'NONE',  #28087 ) ;
#8294=CARTESIAN_POINT ( 'NONE',  ( 1.011271242968688311, -0.7347315653655855927, 3.333333333333333481 ) ) ;
#8300=CARTESIAN_POINT ( 'NONE',  ( -1.249999999999999778, 0.000000000000000000, -10.00000000000000000 ) ) ;
#8304=VERTEX_POINT ( 'NONE', #18037 ) ;
#8322=CARTESIAN_POINT ( 'NONE',  ( -26.76431201374261093, 26.27596734087715902, 8.506357886886741326 ) ) ;
#8338=CARTESIAN_POINT ( 'NONE',  ( 1.249999999999999778, 0.000000000000000000, 10.00000000000000000 ) ) ;
#8347=CARTESIAN_POINT ( 'NONE',  ( 1.011271242968694084, -0.7347315653655782652, 10.00000000000000000 ) ) ;
#8349=B_SPLINE_CURVE_WITH_KNOTS ( 'NONE', 3,
 ( #38961, #213, #38458, #49925 ),
 .UNSPECIFIED., .F., .F.,
 ( 4, 4 ),
 ( 0.0006669682284780766154, 0.0007799402130919628204 ),
 .UNSPECIFIED. ) ;
#8354=CARTESIAN_POINT ( 'NONE',  ( -7.576114424932982594, 33.14742743729794938, 7.906207997025717304 ) ) ;
#8355=CARTESIAN_POINT ( 'NONE',  ( 0.1287570809895660084, -0.3962735484563127408, 10.00000000000000000 ) ) ;
#8367=CARTESIAN_POINT ( 'NONE',  ( 1.810969182959398571, -3.505385724216245169, 6.494306115488114983 ) ) ;
#8374=CARTESIAN_POINT ( 'NONE',  ( 17.23491422248386584, -0.5912720620000816441, 8.727788335465566760 ) ) ;
#8380=CARTESIAN_POINT ( 'NONE',  ( 3.630679331413954714, 37.33064849398144958, -8.600750091277037157 ) ) ;
#8385=CARTESIAN_POINT ( 'NONE',  ( -4.412346620047150836, -9.007664521157030535, 9.516222621873129839 ) ) ;
#8389=CARTESIAN_POINT ( 'NONE',  ( -0.6126904405382037622, -1.085824959725731231, 9.981352469109934233 ) ) ;
#8395=VECTOR ( 'NONE', #40986, 1000.000000000000114 ) ;
#8398=DIRECTION ( 'NONE',  ( 0.000000000000000000, 0.000000000000000000, -1.000000000000000000 ) ) ;
#8415=ORIENTED_EDGE ( 'NONE', *, *, #11779, .F. ) ;
#8425=ORIENTED_EDGE ( 'NONE', *, *, #42446, .T. ) ;
#8426=ORIENTED_EDGE ( 'NONE', *, *, #9952, .T. ) ;
#8427=EDGE_LOOP ( 'NONE', ( #44341, #48561, #17065, #32635, #35333 ) ) ;
#8434=CARTESIAN_POINT ( 'NONE',  ( -29.39982726364978660, -16.78152490921149109, 8.356839323120299312 ) ) ;
#8437=CARTESIAN_POINT ( 'NONE',  ( 4.763548243873389154, -16.57409059453848599, 8.727788335465566760 ) ) ;
#8445=CARTESIAN_POINT ( 'NONE',  ( -1.738880908827836524, -0.9455076376091113843, 9.897807938190497978 ) ) ;
#8446=ADVANCED_FACE ( 'NONE', ( #42646 ), #37944, .T. ) ;
#8461=CARTESIAN_POINT ( 'NONE',  ( -31.44259251615275019, -38.95901822126145220, -9.367992836599951190 ) ) ;
#8478=FACE_OUTER_BOUND ( 'NONE', #15897, .T. ) ;
#8479=CARTESIAN_POINT ( 'NONE',  ( -1.011271242968683426, -0.7347315653655928092, -10.00000000000000000 ) ) ;
#8480=ORIENTED_EDGE ( 'NONE', *, *, #46007, .T. ) ;
#8490=B_SPLINE_SURFACE_WITH_KNOTS ( 'NONE', 3, 3, ( 
 ( #5332, #20991, #17384, #36672 ),
 ( #17137, #32798, #48387, #28934 ),
 ( #25340, #14026, #49647, #29950 ),
 ( #10691, #45806, #15052, #26605 ) ),
 .UNSPECIFIED., .F., .F., .F.,
 ( 4, 4 ),
 ( 4, 4 ),
 ( 0.000000000000000000, 1.000000000000000000 ),
 ( 0.000000000000000000, 1.000000000000000000 ),
 .UNSPECIFIED. ) ;
#8491=ORIENTED_EDGE ( 'NONE', *, *, #3088, .T. ) ;
#8493=CARTESIAN_POINT ( 'NONE',  ( -32.65539107884902847, -7.204654279305827913, -8.917361510505369182 ) ) ;
#8502=CARTESIAN_POINT ( 'NONE',  ( 29.18392875402930997, 17.44843138996603216, 7.906207997025717304 ) ) ;
#8505=EDGE_LOOP ( 'NONE', ( #4303, #28064, #30740, #1772, #41018, #49478, #50576, #36324, #14338, #7286, #5257, #21628 ) ) ;
#8509=CARTESIAN_POINT ( 'NONE',  ( -36.08557433729205144, 35.58569447144795816, 7.455576670931136185 ) ) ;
#8511=CARTESIAN_POINT ( 'NONE',  ( -1.011271242968693862, 0.7347315653655780432, 3.333333333333333481 ) ) ;
#8512=ORIENTED_EDGE ( 'NONE', *, *, #21185, .T. ) ;
#8523=VERTEX_POINT ( 'NONE', #20322 ) ;
#8529=VECTOR ( 'NONE', #27631, 1000.000000000000000 ) ;
#8550=B_SPLINE_CURVE_WITH_KNOTS ( 'NONE', 3,
 ( #45515, #40505, #34259, #25107 ),
 .UNSPECIFIED., .F., .F.,
 ( 4, 4 ),
 ( 1.734723475976807094E-18, 2.804146970186756761E-05 ),
 .UNSPECIFIED. ) ;
#8558=CARTESIAN_POINT ( 'NONE',  ( -1.249999999999999778, 0.000000000000000000, 10.00000000000000000 ) ) ;
#8565=ORIENTED_EDGE ( 'NONE', *, *, #26877, .F. ) ;
#8567=CARTESIAN_POINT ( 'NONE',  ( -1.011271242968683426, -0.7347315653655928092, 10.00000000000000000 ) ) ;
#8588=CARTESIAN_POINT ( 'NONE',  ( 3.239037401336969602, 50.00000000000000711, -8.917361510505369182 ) ) ;
#8595=EDGE_CURVE ( 'NONE', #4376, #47214, #30524, .T. ) ;
#8597=EDGE_CURVE ( 'NONE', #9976, #18218, #18870, .T. ) ;
#8601=CARTESIAN_POINT ( 'NONE',  ( -9.999999999999994671, 2.168404344971008375E-16, 8.340239149799208107 ) ) ;
#8603=CARTESIAN_POINT ( 'NONE',  ( 29.39982726364966581, 16.78152490921169360, 8.356839323120299312 ) ) ;
#8609=CARTESIAN_POINT ( 'NONE',  ( -16.99749102614300966, 1.320765928724422222, 8.953103998512858652 ) ) ;
#8616=CARTESIAN_POINT ( 'NONE',  ( 45.42829307628542779, 21.98948915213303579, 8.356839323120299312 ) ) ;
#8619=ADVANCED_FACE ( 'NONE', ( #41588 ), #33836, .T. ) ;
#8622=CARTESIAN_POINT ( 'NONE',  ( 0.3862712429686727678, 1.188820645368945605, 10.00000000000000000 ) ) ;
#8631=ORIENTED_EDGE ( 'NONE', *, *, #9250, .T. ) ;
#8642=CARTESIAN_POINT ( 'NONE',  ( 0.9494396179258391966, -9.954826186926261755, 9.646707543097345905 ) ) ;
#8644=CARTESIAN_POINT ( 'NONE',  ( 47.87295225382209907, 14.46560184742433641, -2.408242355805840784 ) ) ;
#8651=CARTESIAN_POINT ( 'NONE',  ( -34.10310225234756132, -15.68274378628470345, 1.982731392810465287 ) ) ;
#8656=DIRECTION ( 'NONE',  ( 0.000000000000000000, 0.000000000000000000, -1.000000000000000000 ) ) ;
#8664=CARTESIAN_POINT ( 'NONE',  ( -0.2458784654125698022, 0.3384226744270473208, 9.992713367193012175 ) ) ;
#8667=DIRECTION ( 'NONE',  ( -0.4374820812098793033, -0.3178493372392781624, -0.8411784753765542133 ) ) ;
#8688=DIRECTION ( 'NONE',  ( -1.000000000000000000, 0.000000000000000000, -0.000000000000000000 ) ) ;
#8692=CARTESIAN_POINT ( 'NONE',  ( 0.7601424845489945792, -1.297311920616997627, 9.927319414211225990 ) ) ;
#8703=EDGE_CURVE ( 'NONE', #16759, #12798, #21427, .T. ) ;
#8709=FACE_OUTER_BOUND ( 'NONE', #48185, .T. ) ;
#8711=CARTESIAN_POINT ( 'NONE',  ( 0.8282505383454039638, 1.889063466747038289, 9.894754715216722118 ) ) ;
#8713=CARTESIAN_POINT ( 'NONE',  ( -50.11058929355266400, 7.578863168071933387, 7.455576670931136185 ) ) ;
#8720=CARTESIAN_POINT ( 'NONE',  ( 0.3862712429686727678, 1.188820645368945605, 3.333333333333333481 ) ) ;
#8726=ORIENTED_EDGE ( 'NONE', *, *, #41819, .T. ) ;
#8731=VERTEX_POINT ( 'NONE', #11045 ) ;
#8738=CARTESIAN_POINT ( 'NONE',  ( 7.574282714737766931, -6.549555713337890772, 3.092310436554633224 ) ) ;
#8747=CARTESIAN_POINT ( 'NONE',  ( -11.73320209285699889, 11.96063479729179768, 9.403735324607438884 ) ) ;
#8756=ADVANCED_FACE ( 'NONE', ( #42582 ), #25622, .T. ) ;
#8779=CARTESIAN_POINT ( 'NONE',  ( -1.011271242968677875, -0.7347315653656004697, 10.00000000000000000 ) ) ;
#8793=ORIENTED_EDGE ( 'NONE', *, *, #9890, .T. ) ;
#8805=CARTESIAN_POINT ( 'NONE',  ( -0.7849184246622071814, 1.242376769534369041, 9.958264684458713489 ) ) ;
#8806=CARTESIAN_POINT ( 'NONE',  ( -2.961022939495062900, 16.59676755884084187, 2.590526750877053086 ) ) ;
#8818=CARTESIAN_POINT ( 'NONE',  ( 1.512516825103249918, -0.5229758018505162864, 9.919954280166518146 ) ) ;
#8823=CARTESIAN_POINT ( 'NONE',  ( 8.277096487746778308, -33.14818118907697198, 7.455576670931136185 ) ) ;
#8828=CARTESIAN_POINT ( 'NONE',  ( -0.1475726264153620626, -1.496347932843211215, 9.927319414211227766 ) ) ;
#8842=CARTESIAN_POINT ( 'NONE',  ( -3.239037401336969602, -50.00000000000000711, -8.917361510505369182 ) ) ;
#8843=CARTESIAN_POINT ( 'NONE',  ( 16.52264463346132572, -2.779753662172757878, 9.403735324607438884 ) ) ;
#8848=CARTESIAN_POINT ( 'NONE',  ( -0.1287570809895658697, 0.3962735484563123523, 10.00000000000000000 ) ) ;
#8854=CARTESIAN_POINT ( 'NONE',  ( -49.89397392339119364, 8.245536726717011433, 7.906207997025717304 ) ) ;
#8858=CARTESIAN_POINT ( 'NONE',  ( -2.945500763482279627, -16.64098165802040086, -9.008049429158100807 ) ) ;
#8863=CARTESIAN_POINT ( 'NONE',  ( -14.91630425054805187, 7.943683830272226132, -9.008049429158102583 ) ) ;
#8871=CARTESIAN_POINT ( 'NONE',  ( -0.3862712429686809279, -1.188820645368943163, 10.00000000000000000 ) ) ;
#8877=B_SPLINE_CURVE_WITH_KNOTS ( 'NONE', 3,
 ( #15988, #46731, #43181, #16496 ),
 .UNSPECIFIED., .F., .F.,
 ( 4, 4 ),
 ( 0.9895749839358303213, 1.000000000000000000 ),
 .UNSPECIFIED. ) ;
#8884=ORIENTED_EDGE ( 'NONE', *, *, #22024, .F. ) ;
#8892=CARTESIAN_POINT ( 'NONE',  ( 1.011271242968683648, 0.7347315653655930312, 10.00000000000000000 ) ) ;
#8893=B_SPLINE_SURFACE_WITH_KNOTS ( 'NONE', 3, 3, ( 
 ( #31987, #178, #12463, #50661 ),
 ( #11458, #42736, #23246, #22989 ),
 ( #39436, #672, #27362, #27114 ),
 ( #38666, #4519, #46564, #39183 ) ),
 .UNSPECIFIED., .F., .F., .F.,
 ( 4, 4 ),
 ( 4, 4 ),
 ( 0.000000000000000000, 1.000000000000000000 ),
 ( 0.000000000000000000, 1.000000000000000000 ),
 .UNSPECIFIED. ) ;
#8898=CARTESIAN_POINT ( 'NONE',  ( -0.3862712429686809279, -1.188820645368943163, 10.00000000000000000 ) ) ;
#8904=EDGE_LOOP ( 'NONE', ( #50306, #32455 ) ) ;
#8905=ORIENTED_EDGE ( 'NONE', *, *, #17405, .T. ) ;
#8907=CARTESIAN_POINT ( 'NONE',  ( 5.083187235775197266, 8.611690166631179366, 9.646707543097347681 ) ) ;
#8919=ORIENTED_EDGE ( 'NONE', *, *, #18737, .F. ) ;
#8924=B_SPLINE_CURVE_WITH_KNOTS ( 'NONE', 3,
 ( #27366, #15324, #27882, #11713 ),
 .UNSPECIFIED., .F., .F.,
 ( 4, 4 ),
 ( 0.001403500796105017863, 0.001586656765098935253 ),
 .UNSPECIFIED. ) ;
#8925=CARTESIAN_POINT ( 'NONE',  ( 0.9602803029231544718, -0.8490247040095941777, 9.976582533991681601 ) ) ;
#8930=CARTESIAN_POINT ( 'NONE',  ( -0.3522231071495601773, 1.258647432227772534, 9.945465957785110334 ) ) ;
#8931=DIRECTION ( 'NONE',  ( 1.000000000000000000, 0.000000000000000000, 0.000000000000000000 ) ) ;
#8937=CARTESIAN_POINT ( 'NONE',  ( 0.9989200098981507736, 1.123829893718967687, 9.927319414211233095 ) ) ;
#8942=VERTEX_POINT ( 'NONE', #41027 ) ;
#8945=PLANE ( 'NONE',  #25321 ) ;
#8956=CARTESIAN_POINT ( 'NONE',  ( 15.62858259096121216, -5.755205073598614440, -9.683996418299976483 ) ) ;
#8959=CARTESIAN_POINT ( 'NONE',  ( 0.9489147763962141324, -2.465022012281490760, 9.847478953136988622 ) ) ;
#8962=EDGE_LOOP ( 'NONE', ( #24262, #42024, #22097 ) ) ;
#8966=VERTEX_POINT ( 'NONE', #33588 ) ;
#8968=CARTESIAN_POINT ( 'NONE',  ( -0.3370904143228963812, 0.2449105217885287067, 10.00000000000000000 ) ) ;
#8975=CARTESIAN_POINT ( 'NONE',  ( -15.80799809827351154, 29.65358618225718956, -8.016098858316205167 ) ) ;
#8979=ORIENTED_EDGE ( 'NONE', *, *, #27450, .F. ) ;
#8980=B_SPLINE_CURVE_WITH_KNOTS ( 'NONE', 3,
 ( #1089, #37022, #13633, #28789 ),
 .UNSPECIFIED., .F., .F.,
 ( 4, 4 ),
 ( 0.8097120833243712790, 0.9322955464062560038 ),
 .UNSPECIFIED. ) ;
#8988=CARTESIAN_POINT ( 'NONE',  ( -0.3862712429686809279, -1.188820645368943163, 3.333333333333333481 ) ) ;
#8994=ADVANCED_FACE ( 'NONE', ( #14319 ), #26045, .T. ) ;
#8998=CARTESIAN_POINT ( 'NONE',  ( -12.97493236725075683, 11.05939663307000664, 8.953103998512858652 ) ) ;
#9001=ORIENTED_EDGE ( 'NONE', *, *, #21786, .T. ) ;
#9027=CARTESIAN_POINT ( 'NONE',  ( -5.781580041793970004, 8.177378108131215129, 3.215106848023555397 ) ) ;
#9028=EDGE_CURVE ( 'NONE', #16183, #21718, #24447, .T. ) ;
#9035=CARTESIAN_POINT ( 'NONE',  ( 31.28234235046230793, 11.28615439405779064, -3.760136334089591248 ) ) ;
#9037=EDGE_LOOP ( 'NONE', ( #25071, #39852, #6769, #38512 ) ) ;
#9045=CARTESIAN_POINT ( 'NONE',  ( 1.019713130072856355, 3.848720492505100843, 4.370690007832189750E-16 ) ) ;
#9065=ORIENTED_EDGE ( 'NONE', *, *, #2594, .T. ) ;
#9084=CARTESIAN_POINT ( 'NONE',  ( 1.841192853132477492, 1.035021892307843583, 9.890170120223997330 ) ) ;
#9085=CARTESIAN_POINT ( 'NONE',  ( -9.998889670239194061, -0.1490146381531308739, 9.282506307616474217 ) ) ;
#9092=CARTESIAN_POINT ( 'NONE',  ( -44.99506233596264337, -23.32283626942287214, 7.455576670931136185 ) ) ;
#9096=VERTEX_POINT ( 'NONE', #30749 ) ;
#9106=CARTESIAN_POINT ( 'NONE',  ( -0.1287570809895658697, 0.3962735484563123523, 10.00000000000000000 ) ) ;
#9113=CARTESIAN_POINT ( 'NONE',  ( -33.64889274059387958, 3.704246042440976439, 8.356839323120299312 ) ) ;
#9114=CARTESIAN_POINT ( 'NONE',  ( 1.011271242968683648, 0.7347315653655930312, -3.333333333333333481 ) ) ;
#9115=ORIENTED_EDGE ( 'NONE', *, *, #3523, .T. ) ;
#9117=CARTESIAN_POINT ( 'NONE',  ( 14.52758583651987223, 8.922352469211173087, 8.953103998512858652 ) ) ;
#9129=CARTESIAN_POINT ( 'NONE',  ( 33.01266944765062306, -5.813986777101467496, 1.847720168420772691 ) ) ;
#9131=CARTESIAN_POINT ( 'NONE',  ( -34.91952936320829792, 13.67027684621028349, -9.422646554964178023 ) ) ;
#9133=AXIS2_PLACEMENT_3D ( 'NONE', #989, #32297, #8931 ) ;
#9139=CARTESIAN_POINT ( 'NONE',  ( -23.82716369509181575, -44.49195112875988656, 8.356839323120299312 ) ) ;
#9140=CARTESIAN_POINT ( 'NONE',  ( 0.3522231071503528765, -1.258647432227843588, 9.945465957785078359 ) ) ;
#9142=CARTESIAN_POINT ( 'NONE',  ( -4.641001526964561030, -50.00000000000000000, -8.016098858316205167 ) ) ;
#9153=VERTEX_POINT ( 'NONE', #6030 ) ;
#9160=CARTESIAN_POINT ( 'NONE',  ( -17.34922095635781147, -33.24536858281880569, 8.914903342594564961 ) ) ;
#9165=CARTESIAN_POINT ( 'NONE',  ( 1.011271242968694084, -0.7347315653655782652, 10.00000000000000000 ) ) ;
#9174=CARTESIAN_POINT ( 'NONE',  ( 0.9599924130074096729, -0.8495346730527926216, 9.948547179989617462 ) ) ;
#9198=ORIENTED_EDGE ( 'NONE', *, *, #16194, .F. ) ;
#9204=B_SPLINE_SURFACE_WITH_KNOTS ( 'NONE', 3, 3, ( 
 ( #41583, #456, #4039, #39964 ),
 ( #16097, #47095, #47856, #4300 ),
 ( #27652, #23549, #8152, #43284 ),
 ( #4786, #19691, #11998, #3075 ) ),
 .UNSPECIFIED., .F., .F., .F.,
 ( 4, 4 ),
 ( 4, 4 ),
 ( 0.000000000000000000, 1.000000000000000000 ),
 ( 0.000000000000000000, 1.000000000000000000 ),
 .UNSPECIFIED. ) ;
#9212=CARTESIAN_POINT ( 'NONE',  ( -6.508636631827791064, -15.75743548351446854, 8.953103998512858652 ) ) ;
#9219=ORIENTED_EDGE ( 'NONE', *, *, #14281, .F. ) ;
#9250=EDGE_CURVE ( 'NONE', #18218, #12217, #29343, .T. ) ;
#9252=B_SPLINE_CURVE_WITH_KNOTS ( 'NONE', 3,
 ( #10639, #34007, #26049, #5785 ),
 .UNSPECIFIED., .F., .F.,
 ( 4, 4 ),
 ( 0.000000000000000000, 0.009762429722931321996 ),
 .UNSPECIFIED. ) ;
#9254=CARTESIAN_POINT ( 'NONE',  ( -14.76429217231967428, -8.192625680377590314, 9.178419661560148768 ) ) ;
#9260=CARTESIAN_POINT ( 'NONE',  ( -15.44803555374685189, -6.237487519713257100, -3.546734833711462365 ) ) ;
#9264=CARTESIAN_POINT ( 'NONE',  ( 0.02889939370645888336, -1.394750214494760110, 9.955131761384823363 ) ) ;
#9266=B_SPLINE_CURVE_WITH_KNOTS ( 'NONE', 3,
 ( #33570, #26102, #14301, #26368 ),
 .UNSPECIFIED., .F., .F.,
 ( 4, 4 ),
 ( 0.001403500796105015260, 0.001586656765099030012 ),
 .UNSPECIFIED. ) ;
#9277=CARTESIAN_POINT ( 'NONE',  ( 0.6108107228405675881, -1.056024183042613140, 9.963925895596188909 ) ) ;
#9283=CARTESIAN_POINT ( 'NONE',  ( -0.4426377647354682865, -1.666766018367764834, 9.928159647716134018 ) ) ;
#9305=CARTESIAN_POINT ( 'NONE',  ( 47.23269937569327226, -16.43609759007049931, -2.408242355805840784 ) ) ;
#9312=ORIENTED_EDGE ( 'NONE', *, *, #29658, .F. ) ;
#9313=CARTESIAN_POINT ( 'NONE',  ( -0.4166666666666664631, 0.000000000000000000, 10.00000000000000000 ) ) ;
#9316=EDGE_CURVE ( 'NONE', #27141, #30805, #42387, .T. ) ;
#9340=CARTESIAN_POINT ( 'NONE',  ( -2.595273106918313033, -2.906811120256372671, 9.741991644047246268 ) ) ;
#9344=CARTESIAN_POINT ( 'NONE',  ( 16.76006782980217125, -2.050259795448531541, 9.178419661560148768 ) ) ;
#9350=EDGE_LOOP ( 'NONE', ( #45241, #15611, #45527, #27875 ) ) ;
#9363=CARTESIAN_POINT ( 'NONE',  ( 45.21167770612395742, 22.65616271077811206, 7.906207997025717304 ) ) ;
#9364=ORIENTED_EDGE ( 'NONE', *, *, #21761, .F. ) ;
#9365=B_SPLINE_CURVE_WITH_KNOTS ( 'NONE', 3,
 ( #29010, #48950, #6411, #5400 ),
 .UNSPECIFIED., .F., .F.,
 ( 4, 4 ),
 ( 0.000000000000000000, 0.2545280377015988749 ),
 .UNSPECIFIED. ) ;
#9367=CARTESIAN_POINT ( 'NONE',  ( 1.377594142017867673, -0.6023266041008059624, 9.944962737616616977 ) ) ;
#9370=CARTESIAN_POINT ( 'NONE',  ( 0.4166666666666664631, 0.000000000000000000, 10.00000000000000000 ) ) ;
#9376=CARTESIAN_POINT ( 'NONE',  ( 26.25702031264353664, -26.77347351953840615, 8.914903342594564961 ) ) ;
#9380=CARTESIAN_POINT ( 'NONE',  ( 16.69947034530964913, -2.312583065866261389, 2.590526750877053086 ) ) ;
#9382=CARTESIAN_POINT ( 'NONE',  ( 25.45361382821543828, -27.58774327458490916, 1.982731392810412441 ) ) ;
#9385=EDGE_CURVE ( 'NONE', #8942, #47543, #48190, .T. ) ;
#9389=CARTESIAN_POINT ( 'NONE',  ( -0.4166666666666669072, 0.000000000000000000, 10.00000000000000000 ) ) ;
#9392=CARTESIAN_POINT ( 'NONE',  ( 1.540526284687965264, -1.371707213411490267, 9.886433018048071730 ) ) ;
#9396=CARTESIAN_POINT ( 'NONE',  ( 0.3862712429686894766, -1.188820645368940276, 10.00000000000000000 ) ) ;
#9398=CARTESIAN_POINT ( 'NONE',  ( -20.21530556545279111, 31.58467066308232063, -9.422646554964174470 ) ) ;
#9404=CARTESIAN_POINT ( 'NONE',  ( -50.11058929355266400, 7.578863168071933387, 7.455576670931136185 ) ) ;
#9410=EDGE_LOOP ( 'NONE', ( #18706, #38084, #1019 ) ) ;
#9414=EDGE_CURVE ( 'NONE', #26571, #50487, #6609, .T. ) ;
#9416=CARTESIAN_POINT ( 'NONE',  ( 17.23491422248386584, -0.5912720620000816441, 8.727788335465566760 ) ) ;
#9424=CARTESIAN_POINT ( 'NONE',  ( -1.275927284277175167, 0.1224368140627496299, 9.976582533991679824 ) ) ;
#9426=CARTESIAN_POINT ( 'NONE',  ( -30.25247992116029394, 39.82368563463828792, -3.760136334089591248 ) ) ;
#9427=CARTESIAN_POINT ( 'NONE',  ( -36.97942854200451990, 6.226705766838657397, 8.914903342594564961 ) ) ;
#9454=CARTESIAN_POINT ( 'NONE',  ( 0.4400426740873927822, -2.015233077865103972, 9.886433018048071730 ) ) ;
#9459=B_SPLINE_CURVE_WITH_KNOTS ( 'NONE', 3,
 ( #30434, #2964, #2718, #50126 ),
 .UNSPECIFIED., .F., .F.,
 ( 4, 4 ),
 ( 0.7491799374948677759, 1.000000000000000000 ),
 .UNSPECIFIED. ) ;
#9466=CARTESIAN_POINT ( 'NONE',  ( 29.39982726364966581, 16.78152490921169360, 8.356839323120299312 ) ) ;
#9468=CARTESIAN_POINT ( 'NONE',  ( -0.9602803029231570253, 0.8490247040095960651, 9.976582533991679824 ) ) ;
#9476=EDGE_LOOP ( 'NONE', ( #39624, #46789, #19400 ) ) ;
#9485=CARTESIAN_POINT ( 'NONE',  ( -1.222012661920452326, 0.2471648704738776681, 9.981352469109934233 ) ) ;
#9487=CARTESIAN_POINT ( 'NONE',  ( -1.011271242968693862, 0.7347315653655780432, -10.00000000000000000 ) ) ;
#9490=CARTESIAN_POINT ( 'NONE',  ( 40.32982405930692948, 10.56057144604287146, -9.387872844313825738 ) ) ;
#9496=CARTESIAN_POINT ( 'NONE',  ( 1.552956552085973607, 0.2464513101957388486, 9.945241992664932695 ) ) ;
#9505=EDGE_CURVE ( 'NONE', #30045, #38616, #31723, .T. ) ;
#9522=CARTESIAN_POINT ( 'NONE',  ( 24.87155650802130680, -38.55075836233088893, -9.367992836599951190 ) ) ;
#9527=CARTESIAN_POINT ( 'NONE',  ( -0.4266413953668892756, -1.250184266969579294, 9.943883492372849631 ) ) ;
#9534=EDGE_CURVE ( 'NONE', #16032, #31922, #26256, .T. ) ;
#9540=CARTESIAN_POINT ( 'NONE',  ( -0.1265591857321690383, -1.213367045380180809, 9.963925895596192461 ) ) ;
#9544=EDGE_CURVE ( 'NONE', #46997, #23241, #46390, .T. ) ;
#9550=CARTESIAN_POINT ( 'NONE',  ( 0.3862712429686810944, 1.188820645368943607, 3.333333333333333481 ) ) ;
#9559=CARTESIAN_POINT ( 'NONE',  ( -0.3862712429686729343, -1.188820645368946050, 10.00000000000000000 ) ) ;
#9561=CARTESIAN_POINT ( 'NONE',  ( -1.249999999999999778, 0.000000000000000000, 3.333333333333333481 ) ) ;
#9566=ORIENTED_EDGE ( 'NONE', *, *, #47719, .T. ) ;
#9579=CARTESIAN_POINT ( 'NONE',  ( 33.86622497129647513, -3.037805405904928868, 7.906207997025717304 ) ) ;
#9589=CARTESIAN_POINT ( 'NONE',  ( 0.000000000000000000, 0.000000000000000000, 0.000000000000000000 ) ) ;
#9593=CARTESIAN_POINT ( 'NONE',  ( 50.11058929355270664, -7.578863168071591438, 7.455576670931136185 ) ) ;
#9601=ORIENTED_EDGE ( 'NONE', *, *, #38117, .T. ) ;
#9604=CARTESIAN_POINT ( 'NONE',  ( 1.721971274562253740, 0.09408549481334846365, 9.928159647716247704 ) ) ;
#9608=EDGE_LOOP ( 'NONE', ( #23657, #44296, #28053, #44120 ) ) ;
#9610=ADVANCED_FACE ( 'NONE', ( #2327 ), #9204, .T. ) ;
#9611=EDGE_CURVE ( 'NONE', #50205, #12217, #47020, .T. ) ;
#9614=CARTESIAN_POINT ( 'NONE',  ( 0.8995557326246120811, 5.891360083018336802, 4.370690007832189750E-16 ) ) ;
#9620=B_SPLINE_CURVE_WITH_KNOTS ( 'NONE', 3,
 ( #9889, #20682, #36357, #1200 ),
 .UNSPECIFIED., .F., .F.,
 ( 4, 4 ),
 ( 0.000000000000000000, 0.0002520763768916309180 ),
 .UNSPECIFIED. ) ;
#9625=CARTESIAN_POINT ( 'NONE',  ( -7.896046458374534893, 6.155518428822186472, 6.185594734181544929 ) ) ;
#9635=B_SPLINE_SURFACE_WITH_KNOTS ( 'NONE', 3, 3, ( 
 ( #2497, #21996, #18138, #37668 ),
 ( #17391, #33057, #21485, #37176 ),
 ( #3491, #42498, #46823, #18889 ),
 ( #3240, #34568, #7622, #19149 ) ),
 .UNSPECIFIED., .F., .F., .F.,
 ( 4, 4 ),
 ( 4, 4 ),
 ( 0.000000000000000000, 1.000000000000000000 ),
 ( 0.000000000000000000, 1.000000000000000000 ),
 .UNSPECIFIED. ) ;
#9640=DIRECTION ( 'NONE',  ( 1.000000000000000000, 0.000000000000000000, 0.000000000000000000 ) ) ;
#9642=DIRECTION ( 'NONE',  ( 0.000000000000000000, 0.000000000000000000, -1.000000000000000000 ) ) ;
#9646=CARTESIAN_POINT ( 'NONE',  ( -0.3862712429686895876, 1.188820645368940720, -10.00000000000000000 ) ) ;
#9653=CARTESIAN_POINT ( 'NONE',  ( 0.1287570809895604018, 0.3962735484563146282, 10.00000000000000000 ) ) ;
#9656=EDGE_CURVE ( 'NONE', #12217, #37517, #14607, .T. ) ;
#9662=CARTESIAN_POINT ( 'NONE',  ( 2.538055338523177440, 33.28424297489108596, -9.367992836599954742 ) ) ;
#9666=CARTESIAN_POINT ( 'NONE',  ( -21.61731705588949737, -25.43568671410585935, -9.367992836599954742 ) ) ;
#9672=ORIENTED_EDGE ( 'NONE', *, *, #24972, .F. ) ;
#9675=B_SPLINE_CURVE_WITH_KNOTS ( 'NONE', 3,
 ( #18654, #14817, #49165, #46343 ),
 .UNSPECIFIED., .F., .F.,
 ( 4, 4 ),
 ( 0.000000000000000000, 0.0002610106747150124813 ),
 .UNSPECIFIED. ) ;
#9690=B_SPLINE_CURVE_WITH_KNOTS ( 'NONE', 3,
 ( #18929, #7411, #50184, #38222 ),
 .UNSPECIFIED., .F., .F.,
 ( 4, 4 ),
 ( 5.208685977958201486E-18, 0.009762429722931323731 ),
 .UNSPECIFIED. ) ;
#9691=CARTESIAN_POINT ( 'NONE',  ( 46.75893035013449861, 17.89420872045614885, 3.199614146704519602 ) ) ;
#9725=ORIENTED_EDGE ( 'NONE', *, *, #36299, .T. ) ;
#9732=VERTEX_POINT ( 'NONE', #961 ) ;
#9733=DIRECTION ( 'NONE',  ( 0.000000000000000000, 0.000000000000000000, 1.000000000000000000 ) ) ;
#9734=CARTESIAN_POINT ( 'NONE',  ( 1.275971930252332243, -0.1228246474626390333, 9.957892297621015132 ) ) ;
#9737=VERTEX_POINT ( 'NONE', #44031 ) ;
#9740=CARTESIAN_POINT ( 'NONE',  ( -15.44803555374685189, -6.237487519713257100, -3.546734833711462365 ) ) ;
#9745=CARTESIAN_POINT ( 'NONE',  ( 1.365263087672787590, -0.5437404457008400138, 9.958264684458717042 ) ) ;
#9747=CARTESIAN_POINT ( 'NONE',  ( -12.15085308559838317, 11.68662139125813226, 2.590526750877053086 ) ) ;
#9761=DIRECTION ( 'NONE',  ( -0.6805276818820399365, -0.4944323023722067556, -0.5407575913134975432 ) ) ;
#9771=CARTESIAN_POINT ( 'NONE',  ( 0.8590960553269455513, 0.9801595984304427578, 9.961915419665690052 ) ) ;
#9775=VERTEX_POINT ( 'NONE', #21199 ) ;
#9782=DIRECTION ( 'NONE',  ( 0.4374820812098837997, -0.3178493372392718341, 0.8411784753765542133 ) ) ;
#9786=EDGE_LOOP ( 'NONE', ( #7195, #23163, #23264, #7541 ) ) ;
#9800=CARTESIAN_POINT ( 'NONE',  ( -1.066995270233474624, 33.23888904628638841, -3.760136334089591248 ) ) ;
#9804=( NAMED_UNIT ( * ) SI_UNIT ( $, .STERADIAN. ) SOLID_ANGLE_UNIT ( ) );
#9805=ADVANCED_FACE ( 'NONE', ( #17352 ), #2261, .T. ) ;
#9806=CARTESIAN_POINT ( 'NONE',  ( -8.277096487746778308, 33.14818118907697198, 7.455576670931136185 ) ) ;
#9825=CARTESIAN_POINT ( 'NONE',  ( -10.69268279052439574, -12.77266927778454964, -2.870787844569587133 ) ) ;
#9837=CARTESIAN_POINT ( 'NONE',  ( -8.277096487746778308, 50.00000000000000000, 7.455576670931136185 ) ) ;
#9841=ADVANCED_FACE ( 'NONE', ( #40205 ), #36264, .T. ) ;
#9848=CARTESIAN_POINT ( 'NONE',  ( 0.000000000000000000, 0.000000000000000000, 0.000000000000000000 ) ) ;
#9851=VERTEX_POINT ( 'NONE', #10908 ) ;
#9869=CARTESIAN_POINT ( 'NONE',  ( -15.39115647749013505, 6.484697992489888208, -9.458680755252684591 ) ) ;
#9871=CARTESIAN_POINT ( 'NONE',  ( 0.000000000000000000, 0.000000000000000000, 10.00000000000000000 ) ) ;
#9879=CARTESIAN_POINT ( 'NONE',  ( 0.3862712429686727678, 1.188820645368945605, 10.00000000000000000 ) ) ;
#9880=CARTESIAN_POINT ( 'NONE',  ( 1.011271242968683648, 0.7347315653655930312, 10.00000000000000000 ) ) ;
#9881=CARTESIAN_POINT ( 'NONE',  ( 44.99506233596246574, 23.32283626942318477, 7.455576670931136185 ) ) ;
#9889=CARTESIAN_POINT ( 'NONE',  ( -0.9390173899430289683, -1.130417317737636651, 9.958264684458541183 ) ) ;
#9890=EDGE_CURVE ( 'NONE', #35501, #32520, #28070, .T. ) ;
#9891=CARTESIAN_POINT ( 'NONE',  ( 16.15814872688565984, 4.048305257546810587, -2.870787844569587133 ) ) ;
#9896=CARTESIAN_POINT ( 'NONE',  ( 3.345242017215822372, -2.159124855890657724, -4.878909776184769953E-16 ) ) ;
#9898=CARTESIAN_POINT ( 'NONE',  ( 23.29043492822826167, -24.10797434788167948, 1.847720168420772691 ) ) ;
#9913=CARTESIAN_POINT ( 'NONE',  ( -1.249999999999999778, 0.000000000000000000, -3.333333333333333481 ) ) ;
#9919=CARTESIAN_POINT ( 'NONE',  ( 24.39427009665985224, 44.07992421011656603, 8.807470649214879543 ) ) ;
#9930=CARTESIAN_POINT ( 'NONE',  ( -36.08557433729204433, 35.58569447144795106, 7.455576670931136185 ) ) ;
#9938=CARTESIAN_POINT ( 'NONE',  ( 1.011271242968694084, -0.7347315653655782652, -10.00000000000000000 ) ) ;
#9952=EDGE_CURVE ( 'NONE', #35009, #339, #26147, .T. ) ;
#9954=B_SPLINE_CURVE_WITH_KNOTS ( 'NONE', 3,
 ( #21306, #6659, #29766, #14364 ),
 .UNSPECIFIED., .F., .F.,
 ( 4, 4 ),
 ( 0.000000000000000000, 0.2637263876330693813 ),
 .UNSPECIFIED. ) ;
#9955=CARTESIAN_POINT ( 'NONE',  ( -0.6108107228405769140, 1.056024183042602482, 9.963925895596188909 ) ) ;
#9968=EDGE_LOOP ( 'NONE', ( #35188, #31710, #6042, #18245 ) ) ;
#9976=VERTEX_POINT ( 'NONE', #3972 ) ;
#9982=B_SPLINE_CURVE_WITH_KNOTS ( 'NONE', 3,
 ( #42087, #6951, #38279, #3089 ),
 .UNSPECIFIED., .F., .F.,
 ( 4, 4 ),
 ( 2.424349759030540154E-19, 0.0003407397535652242774 ),
 .UNSPECIFIED. ) ;
#9995=CARTESIAN_POINT ( 'NONE',  ( -0.9494396179258391966, 9.954826186926261755, 9.646707543097345905 ) ) ;
#9999=CARTESIAN_POINT ( 'NONE',  ( 1.222012661920449439, -0.2471648704738783342, 9.981352469109934233 ) ) ;
#10001=FACE_OUTER_BOUND ( 'NONE', #20278, .T. ) ;
#10005=CARTESIAN_POINT ( 'NONE',  ( 11.73320209285708415, -11.96063479729170886, 9.403735324607438884 ) ) ;
#10009=CARTESIAN_POINT ( 'NONE',  ( -1.456734136747265929, 2.915208416222881294, 9.799352050262545077 ) ) ;
#10015=CARTESIAN_POINT ( 'NONE',  ( -6.875132362119187768, 33.14667368551891258, 8.356839323120299312 ) ) ;
#10017=B_SPLINE_CURVE_WITH_KNOTS ( 'NONE', 3,
 ( #18288, #30369, #45217, #38078 ),
 .UNSPECIFIED., .F., .F.,
 ( 4, 4 ),
 ( 0.0007271047118230567798, 0.006865190725605201105 ),
 .UNSPECIFIED. ) ;
#10034=CARTESIAN_POINT ( 'NONE',  ( -9.999999999999994671, 2.168404344971008375E-16, 8.340239149799208107 ) ) ;
#10050=B_SPLINE_SURFACE_WITH_KNOTS ( 'NONE', 3, 3, ( 
 ( #5738, #1902, #48548, #17549 ),
 ( #8842, #29101, #44720, #24498 ),
 ( #33221, #48805, #13691, #12927 ),
 ( #28587, #36578, #1407, #17042 ) ),
 .UNSPECIFIED., .F., .F., .F.,
 ( 4, 4 ),
 ( 4, 4 ),
 ( 0.000000000000000000, 1.000000000000000000 ),
 ( 0.000000000000000000, 1.000000000000000000 ),
 .UNSPECIFIED. ) ;
#10053=EDGE_CURVE ( 'NONE', #3893, #13210, #37808, .T. ) ;
#10059=ORIENTED_EDGE ( 'NONE', *, *, #15093, .T. ) ;
#10075=CARTESIAN_POINT ( 'NONE',  ( 1.052829316634732892, 0.8818324942345726614, 9.946805383069621698 ) ) ;
#10081=ORIENTED_EDGE ( 'NONE', *, *, #32277, .T. ) ;
#10083=B_SPLINE_CURVE_WITH_KNOTS ( 'NONE', 3,
 ( #16296, #28593, #39653, #17048 ),
 .UNSPECIFIED., .F., .F.,
 ( 4, 4 ),
 ( 3.824224708052577823E-16, 0.009762429722931321996 ),
 .UNSPECIFIED. ) ;
#10084=CARTESIAN_POINT ( 'NONE',  ( -12.16428377685542017, -11.73151505502925929, -9.008049429158100807 ) ) ;
#10090=CARTESIAN_POINT ( 'NONE',  ( 24.39427009665985224, 44.07992421011656603, 8.807470649214879543 ) ) ;
#10091=ORIENTED_EDGE ( 'NONE', *, *, #49304, .T. ) ;
#10092=CARTESIAN_POINT ( 'NONE',  ( -0.7142790906314216981, 1.400791805248629895, 9.945241992664895392 ) ) ;
#10093=CARTESIAN_POINT ( 'NONE',  ( -1.721971274562257515, -0.09408549481333014497, 9.928159647716187308 ) ) ;
#10105=ORIENTED_EDGE ( 'NONE', *, *, #6531, .F. ) ;
#10106=LINE ( 'NONE', #18553, #14497 ) ;
#10113=ORIENTED_EDGE ( 'NONE', *, *, #37510, .F. ) ;
#10127=VECTOR ( 'NONE', #28868, 1000.000000000000114 ) ;
#10139=FACE_OUTER_BOUND ( 'NONE', #16870, .T. ) ;
#10142=DIRECTION ( 'NONE',  ( -1.000000000000000000, 0.000000000000000000, 0.000000000000000000 ) ) ;
#10156=PRODUCT ( 'fan', 'fan', '', ( #39299 ) ) ;
#10162=CARTESIAN_POINT ( 'NONE',  ( 6.875132362119187768, -33.14667368551891258, 8.356839323120299312 ) ) ;
#10167=B_SPLINE_CURVE_WITH_KNOTS ( 'NONE', 3,
 ( #8642, #40447, #47838, #31750 ),
 .UNSPECIFIED., .F., .F.,
 ( 4, 4 ),
 ( 0.7998230999345287140, 0.9869080488566184250 ),
 .UNSPECIFIED. ) ;
#10171=CARTESIAN_POINT ( 'NONE',  ( 0.3862712429686727678, 1.188820645368945605, 10.00000000000000000 ) ) ;
#10175=EDGE_CURVE ( 'NONE', #8966, #48305, #50542, .T. ) ;
#10184=LINE ( 'NONE', #37910, #48800 ) ;
#10187=VERTEX_POINT ( 'NONE', #36315 ) ;
#10197=EDGE_CURVE ( 'NONE', #25811, #16425, #23051, .T. ) ;
#10201=ADVANCED_FACE ( 'NONE', ( #32198 ), #10050, .T. ) ;
#10203=CARTESIAN_POINT ( 'NONE',  ( -31.46770792452106846, 38.94077080897363885, 3.199614146704519602 ) ) ;
#10207=CARTESIAN_POINT ( 'NONE',  ( -14.52758583651993618, -8.922352469211071835, 8.953103998512858652 ) ) ;
#10239=EDGE_CURVE ( 'NONE', #27847, #36062, #2244, .T. ) ;
#10240=CARTESIAN_POINT ( 'NONE',  ( 1.305659100530805361, -0.2632760600745564505, 9.951893257060017817 ) ) ;
#10245=ORIENTED_EDGE ( 'NONE', *, *, #49756, .F. ) ;
#10247=EDGE_CURVE ( 'NONE', #1790, #10360, #45114, .T. ) ;
#10250=CARTESIAN_POINT ( 'NONE',  ( 0.3862712429686894766, -1.188820645368940276, 10.00000000000000000 ) ) ;
#10266=EDGE_CURVE ( 'NONE', #25811, #23429, #17605, .T. ) ;
#10267=CARTESIAN_POINT ( 'NONE',  ( -33.16902712922616558, 37.70469005304312304, 1.847720168420772691 ) ) ;
#10312=EDGE_CURVE ( 'NONE', #10463, #29819, #16977, .T. ) ;
#10337=CARTESIAN_POINT ( 'NONE',  ( 1.249999999999999778, -0.000000000000000000, -10.00000000000000000 ) ) ;
#10342=B_SPLINE_CURVE_WITH_KNOTS ( 'NONE', 3,
 ( #34356, #41781, #31017, #49694 ),
 .UNSPECIFIED., .F., .F.,
 ( 4, 4 ),
 ( 0.000000000000000000, 0.0001252128669263171713 ),
 .UNSPECIFIED. ) ;
#10354=CARTESIAN_POINT ( 'NONE',  ( 0.1287570809895575430, 0.3962735484563150168, -10.00000000000000000 ) ) ;
#10360=VERTEX_POINT ( 'NONE', #47239 ) ;
#10365=ORIENTED_EDGE ( 'NONE', *, *, #18666, .T. ) ;
#10381=ORIENTED_EDGE ( 'NONE', *, *, #50390, .F. ) ;
#10397=CARTESIAN_POINT ( 'NONE',  ( -48.34672127938071640, 13.00749071703899773, 3.199614146704519602 ) ) ;
#10398=DIRECTION ( 'NONE',  ( -0.6805276818820364948, -0.4944323023722119737, 0.5407575913134972101 ) ) ;
#10400=CARTESIAN_POINT ( 'NONE',  ( 1.249999999999999778, 0.000000000000000000, 10.00000000000000000 ) ) ;
#10405=CARTESIAN_POINT ( 'NONE',  ( 33.14391172085758086, 37.72293746533119219, -8.016098858316205167 ) ) ;
#10406=CARTESIAN_POINT ( 'NONE',  ( -14.86945752723352498, -7.944783388878907004, 2.590526750877053086 ) ) ;
#10407=CARTESIAN_POINT ( 'NONE',  ( 1.011271242968688311, -0.7347315653655855927, 10.00000000000000000 ) ) ;
#10409=CARTESIAN_POINT ( 'NONE',  ( 0.4402948852767718524, -2.015117899693914527, 9.894754715216725671 ) ) ;
#10416=CARTESIAN_POINT ( 'NONE',  ( -1.250000000000000222, 0.000000000000000000, 10.00000000000000000 ) ) ;
#10419=ORIENTED_EDGE ( 'NONE', *, *, #41882, .T. ) ;
#10422=CARTESIAN_POINT ( 'NONE',  ( -1.769963848780949478, 9.842115015280430868, 0.000000000000000000 ) ) ;
#10423=CARTESIAN_POINT ( 'NONE',  ( 28.52604530808654815, 41.07801380285680892, -3.760136334089591248 ) ) ;
#10463=VERTEX_POINT ( 'NONE', #84 ) ;
#10471=ORIENTED_EDGE ( 'NONE', *, *, #9611, .T. ) ;
#10472=ORIENTED_EDGE ( 'NONE', *, *, #9611, .F. ) ;
#10476=CARTESIAN_POINT ( 'NONE',  ( 0.3862712429686978033, -1.188820645368937834, 10.00000000000000000 ) ) ;
#10480=ORIENTED_EDGE ( 'NONE', *, *, #2418, .F. ) ;
#10481=CARTESIAN_POINT ( 'NONE',  ( 25.04522487443081502, -22.77512090857307925, 8.356839323120299312 ) ) ;
#10487=CARTESIAN_POINT ( 'NONE',  ( -1.057156451998854996, 0.7920882637787067804, 9.943883492372851407 ) ) ;
#10489=EDGE_LOOP ( 'NONE', ( #37756, #30420, #2589, #21081 ) ) ;
#10493=EDGE_CURVE ( 'NONE', #21514, #24866, #8980, .T. ) ;
#10501=ORIENTED_EDGE ( 'NONE', *, *, #1979, .T. ) ;
#10505=CARTESIAN_POINT ( 'NONE',  ( 10.28825587112223161, -13.03847615613158517, 3.266473740018926541 ) ) ;
#10508=EDGE_LOOP ( 'NONE', ( #8425, #18349, #48223, #39121 ) ) ;
#10511=CARTESIAN_POINT ( 'NONE',  ( 1.543575086786857176, -5.756316005467325247, -1.301042606982605321E-15 ) ) ;
#10516=EDGE_CURVE ( 'NONE', #30605, #8966, #32895, .T. ) ;
#10518=ORIENTED_EDGE ( 'NONE', *, *, #21829, .F. ) ;
#10519=CARTESIAN_POINT ( 'NONE',  ( 0.000000000000000000, 0.000000000000000000, 0.000000000000000000 ) ) ;
#10533=CARTESIAN_POINT ( 'NONE',  ( -0.3370904143228943828, -0.2449105217885308716, 10.00000000000000000 ) ) ;
#10539=B_SPLINE_CURVE_WITH_KNOTS ( 'NONE', 3,
 ( #40371, #8818, #20353, #36029 ),
 .UNSPECIFIED., .F., .F.,
 ( 4, 4 ),
 ( 0.001152428489661395028, 0.001623376834729682886 ),
 .UNSPECIFIED. ) ;
#10542=CARTESIAN_POINT ( 'NONE',  ( -18.79997501618753830, -32.48828710620296789, 6.057468652304065060 ) ) ;
#10543=CARTESIAN_POINT ( 'NONE',  ( 0.3656201545664388708, -2.182515578491310393, 9.881002359080277131 ) ) ;
#10547=CARTESIAN_POINT ( 'NONE',  ( -1.917969350850688315, 0.3547183498317107442, 9.896382706792438810 ) ) ;
#10549=CARTESIAN_POINT ( 'NONE',  ( -1.011271242968677875, -0.7347315653656004697, 10.00000000000000000 ) ) ;
#10562=ORIENTED_EDGE ( 'NONE', *, *, #46361, .F. ) ;
#10577=ORIENTED_EDGE ( 'NONE', *, *, #10053, .T. ) ;
#10578=DIRECTION ( 'NONE',  ( -0.2599384441937612200, -0.8000082703740950540, -0.5407575913134975432 ) ) ;
#10584=FACE_OUTER_BOUND ( 'NONE', #13014, .T. ) ;
#10589=B_SPLINE_CURVE_WITH_KNOTS ( 'NONE', 3,
 ( #225, #50457, #38715, #27667 ),
 .UNSPECIFIED., .F., .F.,
 ( 4, 4 ),
 ( 0.9890644561682319091, 1.000000000000000000 ),
 .UNSPECIFIED. ) ;
#10602=VECTOR ( 'NONE', #45462, 1000.000000000000000 ) ;
#10603=EDGE_LOOP ( 'NONE', ( #14283, #22505, #36317, #16123, #41540, #50252, #49482, #14904, #27974, #50566, #14044, #36094, #4274, #18683, #35581 ) ) ;
#10616=CARTESIAN_POINT ( 'NONE',  ( -0.4500758073841509277, -0.7003689023519117374, 9.985686052694763504 ) ) ;
#10621=EDGE_LOOP ( 'NONE', ( #11422, #7723, #18595 ) ) ;
#10635=CARTESIAN_POINT ( 'NONE',  ( -2.143303323993650533, 0.2858885274054065451, 9.882710035074774524 ) ) ;
#10639=CARTESIAN_POINT ( 'NONE',  ( -1.962558162477761714, 3.366505435501197407, 9.741991644046970933 ) ) ;
#10646=EDGE_CURVE ( 'NONE', #15843, #38289, #35991, .T. ) ;
#10648=FACE_OUTER_BOUND ( 'NONE', #9608, .T. ) ;
#10649=CARTESIAN_POINT ( 'NONE',  ( 17.51065725283126895, -28.41934970907778890, -9.367992836599954742 ) ) ;
#10651=ADVANCED_FACE ( 'NONE', ( #13867 ), #37526, .T. ) ;
#10653=CARTESIAN_POINT ( 'NONE',  ( -0.8431937073480634259, 1.111389989012122825, 9.955131761384899747 ) ) ;
#10660=CARTESIAN_POINT ( 'NONE',  ( -35.51846793572368455, 35.99772139009146343, 7.906207997025717304 ) ) ;
#10666=ORIENTED_EDGE ( 'NONE', *, *, #3543, .F. ) ;
#10668=ORIENTED_EDGE ( 'NONE', *, *, #27087, .T. ) ;
#10672=CARTESIAN_POINT ( 'NONE',  ( 18.67411147745603373, 27.51799019669827473, -3.760136334089591248 ) ) ;
#10674=EDGE_LOOP ( 'NONE', ( #25649, #44963, #20366 ) ) ;
#10681=CARTESIAN_POINT ( 'NONE',  ( -48.99656738986512039, 11.00747004110376182, 1.847720168420772691 ) ) ;
#10689=CARTESIAN_POINT ( 'NONE',  ( -1.250000000000000222, 0.000000000000000000, 10.00000000000000000 ) ) ;
#10691=CARTESIAN_POINT ( 'NONE',  ( 34.38425513258721367, -36.82177522737821107, 8.807470649214879543 ) ) ;
#10701=CARTESIAN_POINT ( 'NONE',  ( -45.21167770612412085, -22.65616271077779942, 7.906207997025717304 ) ) ;
#10724=CARTESIAN_POINT ( 'NONE',  ( 3.893440183625898054, 0.6391102933654070339, 6.494306319013603890 ) ) ;
#10725=EDGE_LOOP ( 'NONE', ( #914, #47443, #43739 ) ) ;
#10728=AXIS2_PLACEMENT_3D ( 'NONE', #17800, #37576, #2400 ) ;
#10734=ORIENTED_EDGE ( 'NONE', *, *, #4524, .T. ) ;
#10735=ORIENTED_EDGE ( 'NONE', *, *, #45665, .F. ) ;
#10739=CARTESIAN_POINT ( 'NONE',  ( 31.44259251615245887, 38.95901822126168668, -9.367992836599954742 ) ) ;
#10748=ORIENTED_EDGE ( 'NONE', *, *, #46572, .F. ) ;
#10750=CARTESIAN_POINT ( 'NONE',  ( 15.80799809827373004, -29.65358618225706522, -8.016098858316199838 ) ) ;
#10751=CARTESIAN_POINT ( 'NONE',  ( -22.69295089195507487, -45.31600496604688999, 7.455576670931136185 ) ) ;
#10758=VERTEX_POINT ( 'NONE', #22844 ) ;
#10760=CARTESIAN_POINT ( 'NONE',  ( 7.749480817862238524, 14.85497772329518895, 9.403735324607438884 ) ) ;
#10762=CARTESIAN_POINT ( 'NONE',  ( 15.62858259096121216, -5.755205073598614440, -9.683996418299976483 ) ) ;
#10786=ORIENTED_EDGE ( 'NONE', *, *, #18236, .T. ) ;
#10787=CARTESIAN_POINT ( 'NONE',  ( 1.011271242968683648, 0.7347315653655930312, 10.00000000000000000 ) ) ;
#10792=CARTESIAN_POINT ( 'NONE',  ( -0.3862712429686809279, -1.188820645368943163, 10.00000000000000000 ) ) ;
#10797=CARTESIAN_POINT ( 'NONE',  ( -1.052829316634559920, -0.8818324942353437113, 9.946805383069644790 ) ) ;
#10799=B_SPLINE_CURVE_WITH_KNOTS ( 'NONE', 3,
 ( #4348, #39507, #38743, #43584 ),
 .UNSPECIFIED., .F., .F.,
 ( 4, 4 ),
 ( 0.003717747231047226469, 0.009855833117593325310 ),
 .UNSPECIFIED. ) ;
#10801=EDGE_CURVE ( 'NONE', #4426, #21356, #29154, .T. ) ;
#10814=CARTESIAN_POINT ( 'NONE',  ( -35.51846793572368455, 35.99772139009146343, 7.906207997025717304 ) ) ;
#10816=CARTESIAN_POINT ( 'NONE',  ( 12.15085308559846844, -11.68662139125803989, 2.590526750877053086 ) ) ;
#10833=EDGE_CURVE ( 'NONE', #44983, #20782, #35255, .T. ) ;
#10845=CARTESIAN_POINT ( 'NONE',  ( -0.3862712429686977478, 1.188820645368937390, 3.333333333333333481 ) ) ;
#10850=EDGE_LOOP ( 'NONE', ( #15242, #15535, #34405 ) ) ;
#10853=VERTEX_POINT ( 'NONE', #28228 ) ;
#10858=ADVANCED_FACE ( 'NONE', ( #36445 ), #33002, .T. ) ;
#10865=CARTESIAN_POINT ( 'NONE',  ( 1.249999999999999778, 0.000000000000000000, 10.00000000000000000 ) ) ;
#10873=CARTESIAN_POINT ( 'NONE',  ( -45.42829307628559832, -21.98948915213271960, 8.356839323120299312 ) ) ;
#10876=DIRECTION ( 'NONE',  ( 0.000000000000000000, 0.000000000000000000, 1.000000000000000000 ) ) ;
#10893=B_SPLINE_SURFACE_WITH_KNOTS ( 'NONE', 3, 3, ( 
 ( #28310, #32420, #48015, #44192 ),
 ( #24723, #40370, #20856, #36539 ),
 ( #48264, #28816, #44437, #9313 ),
 ( #24975, #9806, #45183, #18004 ) ),
 .UNSPECIFIED., .F., .F., .F.,
 ( 4, 4 ),
 ( 4, 4 ),
 ( 0.000000000000000000, 1.000000000000000000 ),
 ( 0.000000000000000000, 1.000000000000000000 ),
 .UNSPECIFIED. ) ;
#10901=CARTESIAN_POINT ( 'NONE',  ( 3.441214337941712387, -1.549069628443871860, 9.865049507598753209 ) ) ;
#10907=VERTEX_POINT ( 'NONE', #20516 ) ;
#10908=CARTESIAN_POINT ( 'NONE',  ( -10.00000000000000000, 0.000000000000000000, 0.000000000000000000 ) ) ;
#10923=CARTESIAN_POINT ( 'NONE',  ( -15.42815683172655028, -34.17926237904570996, 7.697694107796190899 ) ) ;
#10927=EDGE_CURVE ( 'NONE', #50487, #40728, #14424, .T. ) ;
#10939=CARTESIAN_POINT ( 'NONE',  ( 14.29087950072012170, 9.652079258044652832, 8.727788335465566760 ) ) ;
#10948=EDGE_CURVE ( 'NONE', #34658, #10187, #40782, .T. ) ;
#10955=CARTESIAN_POINT ( 'NONE',  ( 16.73672383626881199, 2.341008440548109970, -9.008049429158102583 ) ) ;
#10958=CARTESIAN_POINT ( 'NONE',  ( 7.576114424932982594, -50.00000000000000711, 7.906207997025717304 ) ) ;
#10959=CARTESIAN_POINT ( 'NONE',  ( -6.174150299305392053, 33.14591993373988998, 8.807470649214879543 ) ) ;
#10970=CARTESIAN_POINT ( 'NONE',  ( 26.25702031264353664, -26.77347351953840615, 8.914903342594564961 ) ) ;
#10981=CARTESIAN_POINT ( 'NONE',  ( -47.88254548617756967, 14.43607691413558669, -3.760136334089591248 ) ) ;
#10983=CARTESIAN_POINT ( 'NONE',  ( 14.29087950072012170, 9.652079258044652832, 8.727788335465566760 ) ) ;
#10988=CARTESIAN_POINT ( 'NONE',  ( 0.4400426740873927822, -2.015233077865103972, 9.886433018048071730 ) ) ;
#10998=CARTESIAN_POINT ( 'NONE',  ( 1.011271242968694084, -0.7347315653655782652, -10.00000000000000000 ) ) ;
#11000=B_SPLINE_SURFACE_WITH_KNOTS ( 'NONE', 3, 3, ( 
 ( #7058, #27579, #8079, #2929 ),
 ( #26550, #11663, #49833, #18581 ),
 ( #19089, #50092, #31173, #7826 ),
 ( #27315, #15757, #15006, #43214 ) ),
 .UNSPECIFIED., .F., .F., .F.,
 ( 4, 4 ),
 ( 4, 4 ),
 ( 0.000000000000000000, 1.000000000000000000 ),
 ( 0.000000000000000000, 1.000000000000000000 ),
 .UNSPECIFIED. ) ;
#11004=CARTESIAN_POINT ( 'NONE',  ( 7.216980890441427654, -6.922079660550236824, 0.000000000000000000 ) ) ;
#11005=VECTOR ( 'NONE', #11214, 1000.000000000000114 ) ;
#11006=CARTESIAN_POINT ( 'NONE',  ( 1.250000000000000222, 0.000000000000000000, 10.00000000000000000 ) ) ;
#11008=CARTESIAN_POINT ( 'NONE',  ( 9.999626982420835475, 0.09954095390207136351, 8.968381510274435087 ) ) ;
#11009=CARTESIAN_POINT ( 'NONE',  ( 7.398363427652525637, -15.19415887381133246, -9.008049429158100807 ) ) ;
#11022=CARTESIAN_POINT ( 'NONE',  ( -29.61572577327014955, -16.11461842845715253, 8.807470649214879543 ) ) ;
#11023=CARTESIAN_POINT ( 'NONE',  ( 0.8285222815141930486, 1.889008401827334094, 9.886433018048068178 ) ) ;
#11025=B_SPLINE_CURVE_WITH_KNOTS ( 'NONE', 3,
 ( #23797, #43530, #28151, #8892 ),
 .UNSPECIFIED., .F., .F.,
 ( 4, 4 ),
 ( 0.9895749839358304323, 1.000000000000000000 ),
 .UNSPECIFIED. ) ;
#11029=CARTESIAN_POINT ( 'NONE',  ( -6.619412807845042046, 7.495556955913086128, 9.646707543097347681 ) ) ;
#11045=CARTESIAN_POINT ( 'NONE',  ( -8.001683061421429599, -5.997755262142646870, 9.282506307616484875 ) ) ;
#11057=CARTESIAN_POINT ( 'NONE',  ( -1.025617443042918353, -1.003000432359008487, 9.950105812514305370 ) ) ;
#11063=CARTESIAN_POINT ( 'NONE',  ( 0.6538612634419860292, 1.160398818844859958, 9.951893257059996500 ) ) ;
#11075=CARTESIAN_POINT ( 'NONE',  ( -1.697332391510605554, -0.8495613812372067031, 9.900811091504550632 ) ) ;
#11083=CARTESIAN_POINT ( 'NONE',  ( 15.98719783915691650, -4.501063718205879916, 3.266473740018926541 ) ) ;
#11086=CARTESIAN_POINT ( 'NONE',  ( -33.01266944765060174, 5.813986777101691317, 1.847720168420772691 ) ) ;
#11093=CARTESIAN_POINT ( 'NONE',  ( -1.011271242968688533, 0.7347315653655859258, 3.333333333333333481 ) ) ;
#11099=EDGE_CURVE ( 'NONE', #47768, #16759, #46825, .T. ) ;
#11107=CARTESIAN_POINT ( 'NONE',  ( 6.619412807845094449, -7.495556955913033725, 9.646707543097347681 ) ) ;
#11110=DIRECTION ( 'NONE',  ( 0.6805276818820362728, 0.4944323023722117516, -0.5407575913134976542 ) ) ;
#11134=VERTEX_POINT ( 'NONE', #39213 ) ;
#11140=VERTEX_POINT ( 'NONE', #42775 ) ;
#11148=CARTESIAN_POINT ( 'NONE',  ( -25.04522487443065160, 22.77512090857326754, 8.356839323120299312 ) ) ;
#11150=CARTESIAN_POINT ( 'NONE',  ( 6.508636631827673824, 15.75743548351451295, 8.953103998512858652 ) ) ;
#11157=CARTESIAN_POINT ( 'NONE',  ( -16.52264463346130796, 2.779753662172870232, 9.403735324607438884 ) ) ;
#11158=EDGE_CURVE ( 'NONE', #26037, #26846, #7710, .T. ) ;
#11162=EDGE_CURVE ( 'NONE', #36434, #16542, #37457, .T. ) ;
#11164=FACE_OUTER_BOUND ( 'NONE', #10725, .T. ) ;
#11170=EDGE_CURVE ( 'NONE', #42215, #38406, #8349, .T. ) ;
#11174=CARTESIAN_POINT ( 'NONE',  ( 0.3443084382174765312, 1.609917862996832705, 9.927568724237749720 ) ) ;
#11207=CARTESIAN_POINT ( 'NONE',  ( 3.888415560953717431, 9.227494953140064737, 3.092310436554745134 ) ) ;
#11210=CARTESIAN_POINT ( 'NONE',  ( 14.86945752723346637, 7.944783388879009145, 2.590526750877053086 ) ) ;
#11214=DIRECTION ( 'NONE',  ( -0.8411784753765542133, -0.000000000000000000, -0.5407575913134976542 ) ) ;
#11220=CARTESIAN_POINT ( 'NONE',  ( 0.7849184246612691540, -1.242376769536456704, 9.958264684458541183 ) ) ;
#11223=CARTESIAN_POINT ( 'NONE',  ( -2.637606039711253736, -0.1407378881970645645, 9.847478953136990398 ) ) ;
#11233=ORIENTED_EDGE ( 'NONE', *, *, #47464, .T. ) ;
#11240=CARTESIAN_POINT ( 'NONE',  ( -10.69268279052439574, -12.77266927778454964, -2.870787844569587133 ) ) ;
#11243=EDGE_CURVE ( 'NONE', #30326, #9775, #18139, .T. ) ;
#11245=EDGE_CURVE ( 'NONE', #28209, #17293, #37703, .T. ) ;
#11264=CARTESIAN_POINT ( 'NONE',  ( -1.249999999999999778, 0.000000000000000000, -3.333333333333333481 ) ) ;
#11273=CARTESIAN_POINT ( 'NONE',  ( 1.104213410210670876, 0.6509177773818231039, 9.976582533991679824 ) ) ;
#11283=CARTESIAN_POINT ( 'NONE',  ( 46.11867747200574286, -19.86470446310233129, -8.016098858316205167 ) ) ;
#11284=CARTESIAN_POINT ( 'NONE',  ( 17.23491422248386584, -0.5912720620000816441, 8.727788335465566760 ) ) ;
#11286=B_SPLINE_CURVE_WITH_KNOTS ( 'NONE', 3,
 ( #7293, #7558, #38617, #31167 ),
 .UNSPECIFIED., .F., .F.,
 ( 4, 4 ),
 ( 0.001152428489661412592, 0.001623376834729782633 ),
 .UNSPECIFIED. ) ;
#11307=ORIENTED_EDGE ( 'NONE', *, *, #49756, .T. ) ;
#11308=CARTESIAN_POINT ( 'NONE',  ( 1.193089574352119264, 0.2545860991493882342, 9.963925895596188909 ) ) ;
#11316=B_SPLINE_SURFACE_WITH_KNOTS ( 'NONE', 3, 3, ( 
 ( #22726, #50638, #15541, #3207 ),
 ( #26835, #9113, #47559, #39660 ),
 ( #8854, #47049, #8609, #1172 ),
 ( #4499, #655, #31454, #11955 ) ),
 .UNSPECIFIED., .F., .F., .F.,
 ( 4, 4 ),
 ( 4, 4 ),
 ( 0.000000000000000000, 1.000000000000000000 ),
 ( 0.000000000000000000, 1.000000000000000000 ),
 .UNSPECIFIED. ) ;
#11323=CARTESIAN_POINT ( 'NONE',  ( -0.3370904143228963812, 0.2449105217885287067, 10.00000000000000000 ) ) ;
#11333=B_SPLINE_CURVE_WITH_KNOTS ( 'NONE', 3,
 ( #6698, #46164, #38533, #34423 ),
 .UNSPECIFIED., .F., .F.,
 ( 4, 4 ),
 ( 0.7998230999345287140, 0.9869080488566183140 ),
 .UNSPECIFIED. ) ;
#11338=CARTESIAN_POINT ( 'NONE',  ( 45.88383801556798147, -6.205508426776791708, 7.455576670931136185 ) ) ;
#11340=CARTESIAN_POINT ( 'NONE',  ( 0.5280496040173446870, -0.6453736966177778811, 9.985671801905168010 ) ) ;
#11345=CARTESIAN_POINT ( 'NONE',  ( 0.3370904143228981575, -0.2449105217885261532, 10.00000000000000000 ) ) ;
#11347=CARTESIAN_POINT ( 'NONE',  ( -13.35436367797847801, -31.26996044524040741, 7.906207997025717304 ) ) ;
#11369=CARTESIAN_POINT ( 'NONE',  ( 1.011271242968688311, -0.7347315653655855927, 10.00000000000000000 ) ) ;
#11371=EDGE_CURVE ( 'NONE', #28673, #9737, #6512, .T. ) ;
#11382=CARTESIAN_POINT ( 'NONE',  ( -18.37190376999613761, -32.73290680288455690, 1.982731392810413773 ) ) ;
#11384=CARTESIAN_POINT ( 'NONE',  ( 0.000000000000000000, 0.000000000000000000, 10.00000000000000000 ) ) ;
#11400=CARTESIAN_POINT ( 'NONE',  ( -26.25702031264333058, 26.77347351953860155, 8.914903342594559632 ) ) ;
#11401=CARTESIAN_POINT ( 'NONE',  ( -33.43156050989129824, 4.370686678976795747, 8.807470649214879543 ) ) ;
#11407=ORIENTED_EDGE ( 'NONE', *, *, #21373, .T. ) ;
#11419=EDGE_CURVE ( 'NONE', #39174, #50425, #18043, .T. ) ;
#11422=ORIENTED_EDGE ( 'NONE', *, *, #15552, .F. ) ;
#11423=CARTESIAN_POINT ( 'NONE',  ( 2.595273106918288164, 2.906811120256387326, 9.741991644047248045 ) ) ;
#11424=EDGE_CURVE ( 'NONE', #5524, #1440, #10106, .T. ) ;
#11425=CARTESIAN_POINT ( 'NONE',  ( -4.395207584381336297, -3.942437227415910073, 9.586754400234161366 ) ) ;
#11428=CARTESIAN_POINT ( 'NONE',  ( 0.2257686176849521831, -1.281370980887823974, 9.986087673579140400 ) ) ;
#11430=CARTESIAN_POINT ( 'NONE',  ( -1.249999999999999778, 0.000000000000000000, 10.00000000000000000 ) ) ;
#11440=CARTESIAN_POINT ( 'NONE',  ( 2.961022939495062900, -16.59676755884084187, 2.590526750877053086 ) ) ;
#11458=CARTESIAN_POINT ( 'NONE',  ( 33.16902712922644270, -37.70469005304286725, 1.847720168420772691 ) ) ;
#11464=CARTESIAN_POINT ( 'NONE',  ( 0.9599924130074096729, -0.8495346730527926216, 9.948547179989617462 ) ) ;
#11468=CARTESIAN_POINT ( 'NONE',  ( -2.569099690548740877, 50.00000000000000711, 3.199614146704519602 ) ) ;
#11477=EDGE_LOOP ( 'NONE', ( #8173, #11902, #11646, #8726 ) ) ;
#11480=PLANE ( 'NONE',  #13358 ) ;
#11482=CARTESIAN_POINT ( 'NONE',  ( -1.011271242968687867, 0.7347315653655861478, 9.972675548442463622 ) ) ;
#11486=CARTESIAN_POINT ( 'NONE',  ( -14.48769039275601145, -30.44468701195584970, 8.807470649214879543 ) ) ;
#11495=B_SPLINE_CURVE_WITH_KNOTS ( 'NONE', 3,
 ( #40584, #5421, #21073, #36758 ),
 .UNSPECIFIED., .F., .F.,
 ( 4, 4 ),
 ( 0.000000000000000000, 2.647279941188460280E-05 ),
 .UNSPECIFIED. ) ;
#11521=EDGE_CURVE ( 'NONE', #31056, #32520, #8877, .T. ) ;
#11531=B_SPLINE_CURVE_WITH_KNOTS ( 'NONE', 3,
 ( #9999, #25402, #1306, #16954 ),
 .UNSPECIFIED., .F., .F.,
 ( 4, 4 ),
 ( 0.9895749839358307653, 1.000000000000000000 ),
 .UNSPECIFIED. ) ;
#11539=CARTESIAN_POINT ( 'NONE',  ( -30.22736451279196856, -39.84193304692609416, -2.408242355805840784 ) ) ;
#11542=CARTESIAN_POINT ( 'NONE',  ( -45.21167770612412085, -22.65616271077779942, 7.906207997025717304 ) ) ;
#11544=CARTESIAN_POINT ( 'NONE',  ( 46.10908423965007330, 19.89422939639137766, 1.847720168420772691 ) ) ;
#11547=VERTEX_POINT ( 'NONE', #36010 ) ;
#11552=ORIENTED_EDGE ( 'NONE', *, *, #31825, .F. ) ;
#11559=CARTESIAN_POINT ( 'NONE',  ( -23.79193388295331602, -28.98609808354994044, -9.422646554964178023 ) ) ;
#11561=CARTESIAN_POINT ( 'NONE',  ( -1.011271242968683426, -0.7347315653655928092, -3.333333333333333481 ) ) ;
#11562=CARTESIAN_POINT ( 'NONE',  ( -1.347864860736281756, -0.3239901621376108931, 9.960033073700792272 ) ) ;
#11571=CARTESIAN_POINT ( 'NONE',  ( -9.696760411816217839, -2.443938934554997999, 0.000000000000000000 ) ) ;
#11581=ADVANCED_FACE ( 'NONE', ( #11633 ), #2682, .T. ) ;
#11584=CARTESIAN_POINT ( 'NONE',  ( -12.78770032058971395, -31.68259716188267916, 7.455576670931136185 ) ) ;
#11585=FACE_OUTER_BOUND ( 'NONE', #44344, .T. ) ;
#11597=B_SPLINE_CURVE_WITH_KNOTS ( 'NONE', 3,
 ( #33234, #9614, #48816, #13703 ),
 .UNSPECIFIED., .F., .F.,
 ( 4, 4 ),
 ( 0.003855596587714113684, 0.009994105792438251826 ),
 .UNSPECIFIED. ) ;
#11601=CARTESIAN_POINT ( 'NONE',  ( -0.3862712429686809279, -1.188820645368943163, 10.00000000000000000 ) ) ;
#11608=FACE_OUTER_BOUND ( 'NONE', #2700, .T. ) ;
#11626=EDGE_CURVE ( 'NONE', #49290, #41616, #38534, .T. ) ;
#11633=FACE_OUTER_BOUND ( 'NONE', #32708, .T. ) ;
#11646=ORIENTED_EDGE ( 'NONE', *, *, #34991, .T. ) ;
#11652=FACE_OUTER_BOUND ( 'NONE', #18192, .T. ) ;
#11654=CARTESIAN_POINT ( 'NONE',  ( 2.961022939495062900, -16.59676755884084187, 2.590526750877053086 ) ) ;
#11657=EDGE_CURVE ( 'NONE', #15177, #11925, #1851, .T. ) ;
#11658=CARTESIAN_POINT ( 'NONE',  ( -28.97821631107938245, -35.56709536735906596, -9.367992836599951190 ) ) ;
#11661=CARTESIAN_POINT ( 'NONE',  ( -31.93002621080269421, -9.285431160462335853, -2.408242355805840784 ) ) ;
#11663=CARTESIAN_POINT ( 'NONE',  ( -33.64889274059387958, 3.704246042440976439, 8.356839323120299312 ) ) ;
#11676=CARTESIAN_POINT ( 'NONE',  ( -4.763548243873389154, 16.57409059453848599, 8.727788335465566760 ) ) ;
#11689=CARTESIAN_POINT ( 'NONE',  ( 1.468446590252912465, 0.3226319952343980058, 9.953784399990622589 ) ) ;
#11691=CARTESIAN_POINT ( 'NONE',  ( 2.462075149652696027, -16.57295996686994499, 9.403735324607438884 ) ) ;
#11704=CARTESIAN_POINT ( 'NONE',  ( -1.011271242968688533, 0.7347315653655859258, 10.00000000000000000 ) ) ;
#11712=EDGE_CURVE ( 'NONE', #48164, #16958, #6419, .T. ) ;
#11713=CARTESIAN_POINT ( 'NONE',  ( 2.188678504086826848, -0.3267089737525829540, 9.881002359080282460 ) ) ;
#11715=CARTESIAN_POINT ( 'NONE',  ( 1.024768877994822525, -0.8112356146995051143, 9.945465957785110334 ) ) ;
#11732=CARTESIAN_POINT ( 'NONE',  ( 2.538055338523173443, 33.28424297489108596, -9.367992836599951190 ) ) ;
#11736=CARTESIAN_POINT ( 'NONE',  ( 0.8155877869298099325, 0.9072449372238458043, 9.963925895597341764 ) ) ;
#11737=B_SPLINE_SURFACE_WITH_KNOTS ( 'NONE', 3, 3, ( 
 ( #41815, #17948, #2069, #45131 ),
 ( #14878, #10015, #18461, #18705 ),
 ( #2309, #42322, #13844, #33631 ),
 ( #33382, #30527, #46127, #48954 ) ),
 .UNSPECIFIED., .F., .F., .F.,
 ( 4, 4 ),
 ( 4, 4 ),
 ( 0.000000000000000000, 1.000000000000000000 ),
 ( 0.000000000000000000, 1.000000000000000000 ),
 .UNSPECIFIED. ) ;
#11748=LINE ( 'NONE', #4552, #12624 ) ;
#11749=EDGE_CURVE ( 'NONE', #40397, #13851, #49751, .T. ) ;
#11757=CARTESIAN_POINT ( 'NONE',  ( 36.08557433729230723, -35.58569447144768105, 7.455576670931136185 ) ) ;
#11759=ORIENTED_EDGE ( 'NONE', *, *, #14623, .T. ) ;
#11762=CARTESIAN_POINT ( 'NONE',  ( -26.25702031264333058, 26.77347351953860155, 8.914903342594559632 ) ) ;
#11776=LINE ( 'NONE', #27934, #21832 ) ;
#11779=EDGE_CURVE ( 'NONE', #19115, #47355, #11333, .T. ) ;
#11788=CARTESIAN_POINT ( 'NONE',  ( -1.011271242968683426, -0.7347315653655928092, 10.00000000000000000 ) ) ;
#11790=CARTESIAN_POINT ( 'NONE',  ( 0.9870575514054733546, 1.980598328282569653, 9.881002359080278907 ) ) ;
#11792=CARTESIAN_POINT ( 'NONE',  ( -0.1287570809895602630, -0.3962735484563142396, 10.00000000000000000 ) ) ;
#11795=ORIENTED_EDGE ( 'NONE', *, *, #27860, .F. ) ;
#11809=EDGE_CURVE ( 'NONE', #8304, #24192, #41322, .T. ) ;
#11814=VERTEX_POINT ( 'NONE', #6957 ) ;
#11815=CARTESIAN_POINT ( 'NONE',  ( -20.40054609052957701, 26.26366202847989229, -3.760136334089591248 ) ) ;
#11816=PLANE ( 'NONE',  #43083 ) ;
#11817=CARTESIAN_POINT ( 'NONE',  ( -27.33593271309441519, 41.94268121623345280, -9.367992836599951190 ) ) ;
#11819=EDGE_CURVE ( 'NONE', #36390, #24051, #20506, .T. ) ;
#11825=CARTESIAN_POINT ( 'NONE',  ( 2.462075149652696027, -16.57295996686994499, 9.403735324607438884 ) ) ;
#11831=CARTESIAN_POINT ( 'NONE',  ( -1.011271242968683204, -0.7347315653655928092, 9.972675548442467175 ) ) ;
#11832=CARTESIAN_POINT ( 'NONE',  ( -16.26331699892973148, -3.800463913881070077, -9.458680755252684591 ) ) ;
#11843=CIRCLE ( 'NONE', #16742, 10.00000000000000000 ) ;
#11846=CARTESIAN_POINT ( 'NONE',  ( 1.721971274562253740, 0.09408549481334846365, 9.928159647716247704 ) ) ;
#11852=CARTESIAN_POINT ( 'NONE',  ( 32.36066692128250821, -7.813306791042813337, 3.199614146704519602 ) ) ;
#11859=CARTESIAN_POINT ( 'NONE',  ( -9.998889670239194061, -0.1490146381531308739, 9.282506307616474217 ) ) ;
#11863=CARTESIAN_POINT ( 'NONE',  ( 15.73090589902275482, 29.60029367929053024, 1.847720168420772691 ) ) ;
#11868=EDGE_CURVE ( 'NONE', #40379, #43927, #49172, .T. ) ;
#11869=CARTESIAN_POINT ( 'NONE',  ( -31.44259251615275019, -38.95901822126145220, -9.367992836599951190 ) ) ;
#11882=EDGE_CURVE ( 'NONE', #39413, #1790, #23618, .T. ) ;
#11883=ORIENTED_EDGE ( 'NONE', *, *, #10175, .T. ) ;
#11888=CARTESIAN_POINT ( 'NONE',  ( -25.60949810002096783, -43.19700938445173932, 1.847720168420772691 ) ) ;
#11896=ORIENTED_EDGE ( 'NONE', *, *, #35080, .F. ) ;
#11897=ORIENTED_EDGE ( 'NONE', *, *, #15854, .T. ) ;
#11901=CARTESIAN_POINT ( 'NONE',  ( 0.1265591857323814795, 1.213367045380162823, 9.963925895596176474 ) ) ;
#11902=ORIENTED_EDGE ( 'NONE', *, *, #10646, .T. ) ;
#11914=CARTESIAN_POINT ( 'NONE',  ( 0.3370904143228924954, 0.2449105217885333141, 10.00000000000000000 ) ) ;
#11915=ORIENTED_EDGE ( 'NONE', *, *, #11371, .F. ) ;
#11920=CARTESIAN_POINT ( 'NONE',  ( -9.760995290733800900, 2.173239732351794462, 9.646707543097347681 ) ) ;
#11925=VERTEX_POINT ( 'NONE', #18995 ) ;
#11926=CARTESIAN_POINT ( 'NONE',  ( -0.2455008416098019286, -1.553107091521327865, 9.945241992664895392 ) ) ;
#11933=CARTESIAN_POINT ( 'NONE',  ( 5.880995097349652312, 0.9650023149932013267, 5.692061405548898279E-16 ) ) ;
#11934=B_SPLINE_CURVE_WITH_KNOTS ( 'NONE', 3,
 ( #238, #15877, #19969, #12273 ),
 .UNSPECIFIED., .F., .F.,
 ( 4, 4 ),
 ( 0.9895749839358302102, 1.000000000000000000 ),
 .UNSPECIFIED. ) ;
#11939=CARTESIAN_POINT ( 'NONE',  ( -1.249999999999999778, 0.000000000000000000, 10.00000000000000000 ) ) ;
#11945=CARTESIAN_POINT ( 'NONE',  ( 0.3370904143228924954, 0.2449105217885333141, 10.00000000000000000 ) ) ;
#11955=CARTESIAN_POINT ( 'NONE',  ( -0.3862712429686809279, -1.188820645368943163, 10.00000000000000000 ) ) ;
#11967=CARTESIAN_POINT ( 'NONE',  ( 15.44803555374680393, 6.237487519713364570, -3.546734833711462365 ) ) ;
#11984=CARTESIAN_POINT ( 'NONE',  ( -16.76006782980216059, 2.050259795448645228, 9.178419661560148768 ) ) ;
#11985=DIRECTION ( 'NONE',  ( 0.1671032855531390526, -0.5142910309547716885, -0.8411784753765542133 ) ) ;
#11992=CARTESIAN_POINT ( 'NONE',  ( 0.000000000000000000, 0.000000000000000000, 0.000000000000000000 ) ) ;
#11996=VERTEX_POINT ( 'NONE', #43119 ) ;
#11998=CARTESIAN_POINT ( 'NONE',  ( 15.00099850811936264, 7.462898891544210933, 9.403735324607438884 ) ) ;
#12019=ORIENTED_EDGE ( 'NONE', *, *, #26616, .F. ) ;
#12024=ORIENTED_EDGE ( 'NONE', *, *, #48200, .F. ) ;
#12026=CARTESIAN_POINT ( 'NONE',  ( -1.066995270233474624, 50.00000000000000711, -3.760136334089591248 ) ) ;
#12027=PLANE ( 'NONE',  #3302 ) ;
#12029=CARTESIAN_POINT ( 'NONE',  ( -29.18392875402943432, -17.44843138996582965, 7.906207997025717304 ) ) ;
#12032=CARTESIAN_POINT ( 'NONE',  ( 7.576114424932982594, -33.14742743729794938, 7.906207997025717304 ) ) ;
#12037=EDGE_CURVE ( 'NONE', #339, #2423, #27887, .T. ) ;
#12048=CARTESIAN_POINT ( 'NONE',  ( -44.99506233596265048, -23.32283626942287569, 7.455576670931136185 ) ) ;
#12051=VERTEX_POINT ( 'NONE', #24889 ) ;
#12059=EDGE_CURVE ( 'NONE', #2268, #36390, #31525, .T. ) ;
#12067=ORIENTED_EDGE ( 'NONE', *, *, #41213, .T. ) ;
#12069=CARTESIAN_POINT ( 'NONE',  ( 38.83486119589591112, -15.16159403945135153, -9.387872844313825738 ) ) ;
#12071=CARTESIAN_POINT ( 'NONE',  ( 0.000000000000000000, 0.000000000000000000, 0.000000000000000000 ) ) ;
#12074=CARTESIAN_POINT ( 'NONE',  ( 7.216980890441427654, -6.922079660550236824, 0.000000000000000000 ) ) ;
#12081=CARTESIAN_POINT ( 'NONE',  ( 26.76431201374280278, -26.27596734087696362, 8.506357886886739550 ) ) ;
#12082=ORIENTED_EDGE ( 'NONE', *, *, #48867, .F. ) ;
#12094=B_SPLINE_CURVE_WITH_KNOTS ( 'NONE', 3,
 ( #23133, #20302, #15693, #39567 ),
 .UNSPECIFIED., .F., .F.,
 ( 4, 4 ),
 ( 0.9688112071879413367, 0.9724175925769218409 ),
 .UNSPECIFIED. ) ;
#12096=ORIENTED_EDGE ( 'NONE', *, *, #44586, .T. ) ;
#12102=CARTESIAN_POINT ( 'NONE',  ( -30.25247992116029394, 39.82368563463828792, -3.760136334089591248 ) ) ;
#12104=ORIENTED_EDGE ( 'NONE', *, *, #6484, .T. ) ;
#12118=CARTESIAN_POINT ( 'NONE',  ( -0.3370904143228963812, 0.2449105217885287067, 10.00000000000000000 ) ) ;
#12128=CARTESIAN_POINT ( 'NONE',  ( -2.210477865340801706, -37.43479381012853224, -9.422646554964178023 ) ) ;
#12141=EDGE_LOOP ( 'NONE', ( #25897, #12580, #27329, #7209 ) ) ;
#12144=CARTESIAN_POINT ( 'NONE',  ( -8.176860274785726190, 5.756644512789648616, 9.282506307616472441 ) ) ;
#12149=EDGE_LOOP ( 'NONE', ( #47091, #30563, #25457, #30883 ) ) ;
#12167=B_SPLINE_SURFACE_WITH_KNOTS ( 'NONE', 3, 3, ( 
 ( #8461, #16396, #756, #20748 ),
 ( #40017, #21010, #48407, #40513 ),
 ( #40258, #5596, #36945, #36692 ),
 ( #32062, #12543, #1762, #4838 ) ),
 .UNSPECIFIED., .F., .F., .F.,
 ( 4, 4 ),
 ( 4, 4 ),
 ( 0.000000000000000000, 1.000000000000000000 ),
 ( 0.000000000000000000, 1.000000000000000000 ),
 .UNSPECIFIED. ) ;
#12171=EDGE_CURVE ( 'NONE', #9851, #32219, #31974, .T. ) ;
#12180=CARTESIAN_POINT ( 'NONE',  ( 1.066995270233474624, -33.23888904628638841, -3.760136334089591248 ) ) ;
#12186=CARTESIAN_POINT ( 'NONE',  ( 0.3370904143228981575, -0.2449105217885261532, 10.00000000000000000 ) ) ;
#12187=EDGE_LOOP ( 'NONE', ( #10786, #35264, #42014, #13322 ) ) ;
#12191=CARTESIAN_POINT ( 'NONE',  ( 1.011271242968677653, 0.7347315653656002477, 10.00000000000000000 ) ) ;
#12192=CARTESIAN_POINT ( 'NONE',  ( 15.00099850811936264, 7.462898891544210933, 9.403735324607438884 ) ) ;
#12194=ORIENTED_EDGE ( 'NONE', *, *, #16161, .F. ) ;
#12195=VERTEX_POINT ( 'NONE', #5883 ) ;
#12196=ORIENTED_EDGE ( 'NONE', *, *, #40589, .F. ) ;
#12200=CARTESIAN_POINT ( 'NONE',  ( -1.315487699542658984, 0.8933127557393807372, 9.933337059263839919 ) ) ;
#12206=CARTESIAN_POINT ( 'NONE',  ( 16.99749102614301677, -1.320765928724307425, 8.953103998512858652 ) ) ;
#12209=EDGE_LOOP ( 'NONE', ( #26785, #40468, #18932, #764, #49791, #32387, #42654, #29094, #1131, #23445, #35828, #38764 ) ) ;
#12212=CARTESIAN_POINT ( 'NONE',  ( -2.538055338523173443, -50.00000000000000000, -9.367992836599951190 ) ) ;
#12217=VERTEX_POINT ( 'NONE', #33602 ) ;
#12224=EDGE_CURVE ( 'NONE', #22094, #12195, #3872, .T. ) ;
#12228=LINE ( 'NONE', #27891, #44314 ) ;
#12234=PLANE ( 'NONE',  #30755 ) ;
#12236=ORIENTED_EDGE ( 'NONE', *, *, #34023, .F. ) ;
#12247=ORIENTED_EDGE ( 'NONE', *, *, #7775, .F. ) ;
#12258=B_SPLINE_CURVE_WITH_KNOTS ( 'NONE', 3,
 ( #45962, #7000, #18534, #38323 ),
 .UNSPECIFIED., .F., .F.,
 ( 4, 4 ),
 ( 5.641302087661087512E-05, 0.0003272669002613764534 ),
 .UNSPECIFIED. ) ;
#12259=CARTESIAN_POINT ( 'NONE',  ( -5.951572692819863342, 0.3107723024025113023, -2.642742795433417058E-16 ) ) ;
#12260=CARTESIAN_POINT ( 'NONE',  ( 1.437255894074055185, -3.713052624461447682, -1.301042606982605321E-15 ) ) ;
#12267=LINE ( 'NONE', #50461, #35673 ) ;
#12269=LINE ( 'NONE', #231, #32178 ) ;
#12273=CARTESIAN_POINT ( 'NONE',  ( -1.011271242968688533, 0.7347315653655859258, 10.00000000000000000 ) ) ;
#12274=CARTESIAN_POINT ( 'NONE',  ( 1.286508520038679659, 0.4866366830693329426, 9.972175347158279024 ) ) ;
#12280=CARTESIAN_POINT ( 'NONE',  ( -0.6721397084974984892, -9.977385840602783773, 0.000000000000000000 ) ) ;
#12321=VERTEX_POINT ( 'NONE', #14080 ) ;
#12326=VERTEX_POINT ( 'NONE', #49941 ) ;
#12328=CARTESIAN_POINT ( 'NONE',  ( 0.000000000000000000, 0.000000000000000000, -10.00000000000000000 ) ) ;
#12335=EDGE_CURVE ( 'NONE', #42650, #1069, #42042, .T. ) ;
#12337=CARTESIAN_POINT ( 'NONE',  ( 1.104345476778523016, 0.6507740520594131883, 9.967237415621767127 ) ) ;
#12352=CARTESIAN_POINT ( 'NONE',  ( -22.69295089195507487, -45.31600496604688999, 7.455576670931136185 ) ) ;
#12363=CARTESIAN_POINT ( 'NONE',  ( 17.23491422248386584, -0.5912720620000816441, 8.727788335465566760 ) ) ;
#12364=DIRECTION ( 'NONE',  ( -0.3090169943749515591, 0.9510565162951523099, 0.000000000000000000 ) ) ;
#12366=B_SPLINE_CURVE_WITH_KNOTS ( 'NONE', 3,
 ( #30259, #22803, #25460, #41108 ),
 .UNSPECIFIED., .F., .F.,
 ( 4, 4 ),
 ( 0.7998230999345288250, 0.9869080488566183140 ),
 .UNSPECIFIED. ) ;
#12367=EDGE_CURVE ( 'NONE', #12051, #16336, #10589, .T. ) ;
#12373=EDGE_CURVE ( 'NONE', #10907, #31922, #14315, .T. ) ;
#12393=PRODUCT_DEFINITION_CONTEXT ( 'detailed design', #13525, 'design' ) ;
#12399=CARTESIAN_POINT ( 'NONE',  ( 9.174209336589868258, 3.979181203266223488, 9.646707543097347681 ) ) ;
#12403=DIRECTION ( 'NONE',  ( 0.8411784753765542133, 0.000000000000000000, -0.5407575913134976542 ) ) ;
#12408=CARTESIAN_POINT ( 'NONE',  ( 12.97493236725083676, -11.05939663306990717, 8.953103998512858652 ) ) ;
#12428=CARTESIAN_POINT ( 'NONE',  ( 1.104609456715839766, 0.6504863887005235545, 9.948547179989622791 ) ) ;
#12434=CARTESIAN_POINT ( 'NONE',  ( -9.760995290733800900, 2.173239732351794462, 9.646707543097347681 ) ) ;
#12441=ADVANCED_FACE ( 'NONE', ( #23566 ), #28469, .T. ) ;
#12446=DIRECTION ( 'NONE',  ( 0.1671032855531318084, 0.5142910309547740200, -0.8411784753765541023 ) ) ;
#12448=VERTEX_POINT ( 'NONE', #1732 ) ;
#12450=CARTESIAN_POINT ( 'NONE',  ( -21.61731705588949737, -25.43568671410585935, -9.367992836599954742 ) ) ;
#12453=CARTESIAN_POINT ( 'NONE',  ( 14.29087950072012170, 9.652079258044652832, 8.727788335465566760 ) ) ;
#12460=CARTESIAN_POINT ( 'NONE',  ( -2.595273106918313033, -2.906811120256372671, 9.741991644047246268 ) ) ;
#12463=CARTESIAN_POINT ( 'NONE',  ( 13.59579750444771307, -10.60877755095900632, 8.727788335465566760 ) ) ;
#12465=DIRECTION ( 'NONE',  ( 0.000000000000000000, 0.000000000000000000, -1.000000000000000000 ) ) ;
#12478=LINE ( 'NONE', #19928, #17166 ) ;
#12479=CARTESIAN_POINT ( 'NONE',  ( 24.47767542868285062, -23.18653802921781448, 8.807470649214879543 ) ) ;
#12490=ORIENTED_EDGE ( 'NONE', *, *, #42891, .F. ) ;
#12494=ORIENTED_EDGE ( 'NONE', *, *, #3523, .F. ) ;
#12496=CARTESIAN_POINT ( 'NONE',  ( 0.6369768774142625656, -1.285364331396288806, 9.950105812514305370 ) ) ;
#12502=CARTESIAN_POINT ( 'NONE',  ( 0.4402948852767718524, -2.015117899693914527, 9.894754715216725671 ) ) ;
#12514=CARTESIAN_POINT ( 'NONE',  ( -48.33712804702535237, -13.03701565032741705, -9.367992836599951190 ) ) ;
#12516=CARTESIAN_POINT ( 'NONE',  ( -29.61572577327014955, -16.11461842845715253, 8.807470649214879543 ) ) ;
#12521=CARTESIAN_POINT ( 'NONE',  ( 49.46074318306830975, -9.578883844006831794, 8.807470649214879543 ) ) ;
#12523=CARTESIAN_POINT ( 'NONE',  ( 35.87018513526846419, 11.05844981164239194, -6.568693074176337632 ) ) ;
#12524=B_SPLINE_CURVE_WITH_KNOTS ( 'NONE', 3,
 ( #8805, #4190, #32400, #19828 ),
 .UNSPECIFIED., .F., .F.,
 ( 4, 4 ),
 ( 0.9890644561682322422, 1.000000000000000000 ),
 .UNSPECIFIED. ) ;
#12536=CARTESIAN_POINT ( 'NONE',  ( -2.707743684961791075, -37.43817128298309882, -5.338708898921614043 ) ) ;
#12543=CARTESIAN_POINT ( 'NONE',  ( -23.31729631074215092, -24.19776167542410406, -8.016098858316205167 ) ) ;
#12550=VERTEX_POINT ( 'NONE', #20719 ) ;
#12558=CARTESIAN_POINT ( 'NONE',  ( -7.398363427652413726, 15.19415887381139285, -9.008049429158102583 ) ) ;
#12563=CARTESIAN_POINT ( 'NONE',  ( 2.569099690548740877, -33.19126772784019153, 3.199614146704519602 ) ) ;
#12569=B_SPLINE_SURFACE_WITH_KNOTS ( 'NONE', 3, 3, ( 
 ( #10090, #41393, #29344, #37569 ),
 ( #5731, #2389, #37325, #17033 ),
 ( #40647, #33214, #18033, #5482 ),
 ( #48288, #17540, #21133, #44463 ) ),
 .UNSPECIFIED., .F., .F., .F.,
 ( 4, 4 ),
 ( 4, 4 ),
 ( 0.000000000000000000, 1.000000000000000000 ),
 ( 0.000000000000000000, 1.000000000000000000 ),
 .UNSPECIFIED. ) ;
#12572=CARTESIAN_POINT ( 'NONE',  ( -35.51846793572368455, 35.99772139009146343, 7.906207997025717304 ) ) ;
#12578=CARTESIAN_POINT ( 'NONE',  ( 0.1287570809895660084, -0.3962735484563127408, 10.00000000000000000 ) ) ;
#12579=CARTESIAN_POINT ( 'NONE',  ( -12.35406723005387875, 11.51001571518090039, 9.178419661560148768 ) ) ;
#12580=ORIENTED_EDGE ( 'NONE', *, *, #9414, .T. ) ;
#12598=ORIENTED_EDGE ( 'NONE', *, *, #41392, .T. ) ;
#12602=ORIENTED_EDGE ( 'NONE', *, *, #11424, .F. ) ;
#12604=CARTESIAN_POINT ( 'NONE',  ( 5.888214538810389698, 16.20866436362417673, 8.727788335465566760 ) ) ;
#12615=CARTESIAN_POINT ( 'NONE',  ( 1.565927753002672285, -1.491090762200744102, 9.882710035074770971 ) ) ;
#12617=VERTEX_POINT ( 'NONE', #39986 ) ;
#12624=VECTOR ( 'NONE', #8667, 1000.000000000000114 ) ;
#12626=ORIENTED_EDGE ( 'NONE', *, *, #30625, .F. ) ;
#12634=CARTESIAN_POINT ( 'NONE',  ( -1.066995270233474624, 33.23888904628638841, -3.760136334089591248 ) ) ;
#12636=ORIENTED_EDGE ( 'NONE', *, *, #24457, .T. ) ;
#12646=CARTESIAN_POINT ( 'NONE',  ( 0.3862712429686894766, -1.188820645368940276, 10.00000000000000000 ) ) ;
#12649=CARTESIAN_POINT ( 'NONE',  ( 1.249999999999999778, 0.000000000000000000, 9.972675548442463622 ) ) ;
#12654=CARTESIAN_POINT ( 'NONE',  ( -2.052581215100349521, 0.2042358160481012597, 9.886433018048073507 ) ) ;
#12658=CARTESIAN_POINT ( 'NONE',  ( -6.604186672497962540, 1.848482776016375340, 9.753789706659947711 ) ) ;
#12676=CARTESIAN_POINT ( 'NONE',  ( -15.00099850811941948, -7.462898891544107016, 9.403735324607438884 ) ) ;
#12683=CARTESIAN_POINT ( 'NONE',  ( 48.34672127938079456, -13.00749071703866555, 3.199614146704519602 ) ) ;
#12689=CARTESIAN_POINT ( 'NONE',  ( 28.96803024440893992, 18.11533787072037072, 7.455576670931136185 ) ) ;
#12698=B_SPLINE_CURVE_WITH_KNOTS ( 'NONE', 3,
 ( #4056, #23035, #27153, #15853 ),
 .UNSPECIFIED., .F., .F.,
 ( 4, 4 ),
 ( 0.000000000000000000, 0.002217981418793440844 ),
 .UNSPECIFIED. ) ;
#12700=CARTESIAN_POINT ( 'NONE',  ( -3.087186397306470820, -2.514307945609864259, -2.642742795433417058E-16 ) ) ;
#12704=CARTESIAN_POINT ( 'NONE',  ( -1.035950918207909632, -50.00000000000000711, -2.408242355805840784 ) ) ;
#12721=CARTESIAN_POINT ( 'NONE',  ( -7.398363427652414614, 15.19415887381139108, -9.008049429158100807 ) ) ;
#12722=CARTESIAN_POINT ( 'NONE',  ( 0.4183568061215536815, -10.00547810715653618, 6.429802539306306741 ) ) ;
#12732=CARTESIAN_POINT ( 'NONE',  ( 1.540571744149447309, -1.371626741452957488, 9.889206917020304743 ) ) ;
#12735=CARTESIAN_POINT ( 'NONE',  ( -7.749480817862350435, -14.85497772329513211, 9.403735324607438884 ) ) ;
#12748=CARTESIAN_POINT ( 'NONE',  ( -4.207128120815918256E-14, 3.058192377181588826E-14, 10.00000000000000000 ) ) ;
#12754=EDGE_LOOP ( 'NONE', ( #34695, #6486, #49550 ) ) ;
#12768=VERTEX_POINT ( 'NONE', #22980 ) ;
#12771=CARTESIAN_POINT ( 'NONE',  ( 22.69295089195473025, 45.31600496604705341, 7.455576670931136185 ) ) ;
#12773=CARTESIAN_POINT ( 'NONE',  ( -27.33593271309441519, 41.94268121623345991, -9.367992836599954742 ) ) ;
#12793=CARTESIAN_POINT ( 'NONE',  ( 0.9341213539222221751, 1.950087977540064577, 9.885585981620945262 ) ) ;
#12794=CARTESIAN_POINT ( 'NONE',  ( 49.46074318306830975, -9.578883844006831794, 8.807470649214879543 ) ) ;
#12798=VERTEX_POINT ( 'NONE', #4754 ) ;
#12804=CARTESIAN_POINT ( 'NONE',  ( 50.11058929355270664, -7.578863168071591438, 7.455576670931136185 ) ) ;
#12815=CARTESIAN_POINT ( 'NONE',  ( -14.48769039275601145, -30.44468701195584970, 8.807470649214879543 ) ) ;
#12819=FACE_OUTER_BOUND ( 'NONE', #27957, .T. ) ;
#12821=CARTESIAN_POINT ( 'NONE',  ( -25.63461350838931452, 43.17876197216397571, -8.016098858316205167 ) ) ;
#12833=CARTESIAN_POINT ( 'NONE',  ( 46.76852358249013264, -17.86468378716708827, -9.367992836599951190 ) ) ;
#12839=CARTESIAN_POINT ( 'NONE',  ( -2.052570692346794790, 0.2041439924650417514, 9.889206917020306520 ) ) ;
#12853=CARTESIAN_POINT ( 'NONE',  ( -0.5386300094813477601, 1.098626330213929636, 9.993783931180534097 ) ) ;
#12874=CARTESIAN_POINT ( 'NONE',  ( 0.1287570809895575430, 0.3962735484563150168, 10.00000000000000000 ) ) ;
#12875=CARTESIAN_POINT ( 'NONE',  ( -1.540617191852276413, 1.371546265746164783, 9.891980816076525684 ) ) ;
#12876=ORIENTED_EDGE ( 'NONE', *, *, #36167, .F. ) ;
#12879=ORIENTED_EDGE ( 'NONE', *, *, #6114, .F. ) ;
#12884=B_SPLINE_SURFACE_WITH_KNOTS ( 'NONE', 3, 3, ( 
 ( #6932, #22573, #41823, #2565 ),
 ( #49976, #29270, #41072, #18209 ),
 ( #5913, #37255, #6667, #33390 ),
 ( #17956, #48962, #13850, #25680 ) ),
 .UNSPECIFIED., .F., .F., .F.,
 ( 4, 4 ),
 ( 4, 4 ),
 ( 0.000000000000000000, 1.000000000000000000 ),
 ( 0.000000000000000000, 1.000000000000000000 ),
 .UNSPECIFIED. ) ;
#12886=EDGE_CURVE ( 'NONE', #31206, #41298, #27686, .T. ) ;
#12906=CARTESIAN_POINT ( 'NONE',  ( 36.08557433729230723, -35.58569447144768105, 7.455576670931136185 ) ) ;
#12920=CARTESIAN_POINT ( 'NONE',  ( -2.538055338523177440, -50.00000000000000711, -9.367992836599954742 ) ) ;
#12924=EDGE_CURVE ( 'NONE', #5904, #20782, #9954, .T. ) ;
#12927=CARTESIAN_POINT ( 'NONE',  ( -0.4166666666666669072, 0.000000000000000000, -10.00000000000000000 ) ) ;
#12932=ORIENTED_EDGE ( 'NONE', *, *, #11809, .F. ) ;
#12941=ADVANCED_FACE ( 'NONE', ( #1817 ), #20676, .T. ) ;
#12947=CARTESIAN_POINT ( 'NONE',  ( -4.641001526964560142, -50.00000000000000711, -8.016098858316199838 ) ) ;
#12975=CARTESIAN_POINT ( 'NONE',  ( -0.9989200098981521059, -1.123829893718962802, 9.927319414211225990 ) ) ;
#12977=VERTEX_POINT ( 'NONE', #2067 ) ;
#12983=B_SPLINE_SURFACE_WITH_KNOTS ( 'NONE', 3, 3, ( 
 ( #32584, #12815, #20757, #21267 ),
 ( #36439, #5868, #41263, #8968 ),
 ( #40523, #48168, #9212, #13558 ),
 ( #36955, #1774, #17419, #33087 ) ),
 .UNSPECIFIED., .F., .F., .F.,
 ( 4, 4 ),
 ( 4, 4 ),
 ( 0.000000000000000000, 1.000000000000000000 ),
 ( 0.000000000000000000, 1.000000000000000000 ),
 .UNSPECIFIED. ) ;
#12985=CARTESIAN_POINT ( 'NONE',  ( -16.52264463346130796, 2.779753662172870232, 9.403735324607438884 ) ) ;
#12993=EDGE_CURVE ( 'NONE', #12217, #43021, #50213, .T. ) ;
#12999=CARTESIAN_POINT ( 'NONE',  ( 1.011271242968688311, -0.7347315653655855927, 3.333333333333333481 ) ) ;
#13001=VERTEX_POINT ( 'NONE', #11283 ) ;
#13014=EDGE_LOOP ( 'NONE', ( #7157, #19689, #27022, #7440 ) ) ;
#13025=CARTESIAN_POINT ( 'NONE',  ( -3.975459390375366997, -0.2195152216756601216, -2.642742795433417058E-16 ) ) ;
#13029=EDGE_CURVE ( 'NONE', #27105, #39341, #15512, .T. ) ;
#13037=AXIS2_PLACEMENT_3D ( 'NONE', #10519, #21562, #41574 ) ;
#13047=VECTOR ( 'NONE', #29700, 1000.000000000000000 ) ;
#13049=B_SPLINE_CURVE_WITH_KNOTS ( 'NONE', 3,
 ( #9398, #16852, #1953, #5799 ),
 .UNSPECIFIED., .F., .F.,
 ( 4, 4 ),
 ( 0.000000000000000000, 0.002466147708923230580 ),
 .UNSPECIFIED. ) ;
#13052=VERTEX_POINT ( 'NONE', #35156 ) ;
#13057=EDGE_CURVE ( 'NONE', #48360, #10360, #27041, .T. ) ;
#13072=VERTEX_POINT ( 'NONE', #7178 ) ;
#13088=VECTOR ( 'NONE', #9782, 1000.000000000000114 ) ;
#13097=CARTESIAN_POINT ( 'NONE',  ( -31.28977333267361871, 11.25592690310926969, -2.408242355805840784 ) ) ;
#13099=CARTESIAN_POINT ( 'NONE',  ( -0.3862712429686729343, -1.188820645368946050, 10.00000000000000000 ) ) ;
#13101=CARTESIAN_POINT ( 'NONE',  ( -0.6909887759940060992, 1.008432015058918552, 9.987567862361069970 ) ) ;
#13105=VERTEX_POINT ( 'NONE', #44319 ) ;
#13120=CARTESIAN_POINT ( 'NONE',  ( 1.222012661920449439, -0.2471648704738783342, 9.981352469109934233 ) ) ;
#13142=EDGE_CURVE ( 'NONE', #46411, #41927, #36893, .T. ) ;
#13148=VERTEX_POINT ( 'NONE', #24850 ) ;
#13179=CARTESIAN_POINT ( 'NONE',  ( -3.808200756227646089, -0.8261963378076270237, 9.741991644047246268 ) ) ;
#13182=CARTESIAN_POINT ( 'NONE',  ( 14.91630425054810161, -7.943683830272123991, -9.008049429158102583 ) ) ;
#13183=CARTESIAN_POINT ( 'NONE',  ( -0.7606162131530730397, 1.296876929034918691, 9.953784399990622589 ) ) ;
#13188=B_SPLINE_CURVE_WITH_KNOTS ( 'NONE', 3,
 ( #494, #27936, #47380, #43573 ),
 .UNSPECIFIED., .F., .F.,
 ( 4, 4 ),
 ( 0.9688112071879397824, 0.9724175925769220630 ),
 .UNSPECIFIED. ) ;
#13194=CARTESIAN_POINT ( 'NONE',  ( 44.99506233596247995, 23.32283626942318833, 7.455576670931136185 ) ) ;
#13196=CARTESIAN_POINT ( 'NONE',  ( -0.3862712429686977478, 1.188820645368937390, 10.00000000000000000 ) ) ;
#13203=CARTESIAN_POINT ( 'NONE',  ( -21.58778298521296080, 25.34222074689773407, 3.199614146704519602 ) ) ;
#13210=VERTEX_POINT ( 'NONE', #744 ) ;
#13211=CARTESIAN_POINT ( 'NONE',  ( 49.89397392339123627, -8.245536726716670373, 7.906207997025717304 ) ) ;
#13216=CARTESIAN_POINT ( 'NONE',  ( -2.051144455471382688, -1.664205274803698620, 9.847478953136990398 ) ) ;
#13224=CARTESIAN_POINT ( 'NONE',  ( -5.083187235775261215, -8.611690166631138510, 9.646707543097347681 ) ) ;
#13230=CARTESIAN_POINT ( 'NONE',  ( 16.73672383626881199, 2.341008440548111302, -9.008049429158100807 ) ) ;
#13232=CARTESIAN_POINT ( 'NONE',  ( -12.78770032058971395, -31.68259716188267916, 7.455576670931136185 ) ) ;
#13235=CARTESIAN_POINT ( 'NONE',  ( 11.73320209285708415, -11.96063479729170886, 9.403735324607438884 ) ) ;
#13252=ADVANCED_FACE ( 'NONE', ( #8709 ), #16639, .F. ) ;
#13262=ORIENTED_EDGE ( 'NONE', *, *, #34934, .T. ) ;
#13282=CARTESIAN_POINT ( 'NONE',  ( 3.886636751349460628, -37.33392444503267171, 6.057468652304066836 ) ) ;
#13300=CARTESIAN_POINT ( 'NONE',  ( -0.4402108221912932051, 2.015156302359635720, 9.891980816043068003 ) ) ;
#13301=B_SPLINE_SURFACE_WITH_KNOTS ( 'NONE', 3, 3, ( 
 ( #2151, #44955, #22148, #14174 ),
 ( #25487, #32688, #45459, #10354 ),
 ( #28838, #26005, #25747, #49036 ),
 ( #40887, #1399, #13182, #25239 ) ),
 .UNSPECIFIED., .F., .F., .F.,
 ( 4, 4 ),
 ( 4, 4 ),
 ( 0.000000000000000000, 1.000000000000000000 ),
 ( 0.000000000000000000, 1.000000000000000000 ),
 .UNSPECIFIED. ) ;
#13314=ORIENTED_EDGE ( 'NONE', *, *, #43350, .T. ) ;
#13322=ORIENTED_EDGE ( 'NONE', *, *, #19405, .T. ) ;
#13328=AXIS2_PLACEMENT_3D ( 'NONE', #47712, #37499, #21560 ) ;
#13330=CARTESIAN_POINT ( 'NONE',  ( -1.114871695981121125, 0.4953159757245923500, 9.963925895596188909 ) ) ;
#13337=CARTESIAN_POINT ( 'NONE',  ( 20.21530556545302559, -31.58467066308217497, -9.422646554964174470 ) ) ;
#13339=EDGE_CURVE ( 'NONE', #8304, #40728, #34076, .T. ) ;
#13345=CARTESIAN_POINT ( 'NONE',  ( -17.51065725283106289, 28.41934970907792746, -9.367992836599954742 ) ) ;
#13346=CARTESIAN_POINT ( 'NONE',  ( -14.91630425054805187, 7.943683830272224355, -9.008049429158100807 ) ) ;
#13356=ORIENTED_EDGE ( 'NONE', *, *, #47630, .T. ) ;
#13357=CARTESIAN_POINT ( 'NONE',  ( 26.18032376592674737, -21.95228666728361233, 7.455576670931136185 ) ) ;
#13358=AXIS2_PLACEMENT_3D ( 'NONE', #11992, #8398, #39454 ) ;
#13369=CARTESIAN_POINT ( 'NONE',  ( 0.7658683902953711264, -0.9641952520609267108, 9.975326647350893694 ) ) ;
#13371=ORIENTED_EDGE ( 'NONE', *, *, #35080, .T. ) ;
#13373=CARTESIAN_POINT ( 'NONE',  ( 3.231548175622897645, -9.463461120997347820, 9.282506307616472441 ) ) ;
#13381=ADVANCED_FACE ( 'NONE', ( #34572 ), #21505, .T. ) ;
#13384=CARTESIAN_POINT ( 'NONE',  ( 0.08756411784060347259, -1.703854692067152676, 9.912102921404990497 ) ) ;
#13386=ORIENTED_EDGE ( 'NONE', *, *, #11099, .T. ) ;
#13391=ORIENTED_EDGE ( 'NONE', *, *, #33473, .F. ) ;
#13396=CARTESIAN_POINT ( 'NONE',  ( 14.91630425054810161, -7.943683830272122215, -9.008049429158100807 ) ) ;
#13399=FACE_OUTER_BOUND ( 'NONE', #20074, .T. ) ;
#13411=B_SPLINE_SURFACE_WITH_KNOTS ( 'NONE', 3, 3, ( 
 ( #15873, #12516, #47126, #15615 ),
 ( #23306, #8434, #24088, #16128 ),
 ( #42795, #12029, #27171, #4071 ),
 ( #27672, #31026, #47374, #39233 ) ),
 .UNSPECIFIED., .F., .F., .F.,
 ( 4, 4 ),
 ( 4, 4 ),
 ( 0.000000000000000000, 1.000000000000000000 ),
 ( 0.000000000000000000, 1.000000000000000000 ),
 .UNSPECIFIED. ) ;
#13414=B_SPLINE_CURVE_WITH_KNOTS ( 'NONE', 3,
 ( #17493, #25448, #6442, #44659 ),
 .UNSPECIFIED., .F., .F.,
 ( 4, 4 ),
 ( 0.000000000000000000, 0.2637263876330696033 ),
 .UNSPECIFIED. ) ;
#13418=CARTESIAN_POINT ( 'NONE',  ( -0.7603004677363125463, 1.297166976436572750, 9.936141075511203624 ) ) ;
#13426=ADVANCED_FACE ( 'NONE', ( #26863 ), #5093, .T. ) ;
#13427=CARTESIAN_POINT ( 'NONE',  ( 1.332485441698145534, -1.351730126698036827, 9.900811091504554184 ) ) ;
#13429=EDGE_CURVE ( 'NONE', #47506, #16542, #44205, .T. ) ;
#13437=CARTESIAN_POINT ( 'NONE',  ( 2.948105490344985480, 9.555557232197198658, 9.282506307616484875 ) ) ;
#13446=ORIENTED_EDGE ( 'NONE', *, *, #24457, .F. ) ;
#13450=CARTESIAN_POINT ( 'NONE',  ( -22.69295089195507131, -45.31600496604688999, 7.455576670931136185 ) ) ;
#13451=CARTESIAN_POINT ( 'NONE',  ( -1.468446590252919348, -0.3226319952343834063, 9.953784399990620813 ) ) ;
#13460=CARTESIAN_POINT ( 'NONE',  ( -25.63461350838931097, 43.17876197216396150, -8.016098858316205167 ) ) ;
#13474=ORIENTED_EDGE ( 'NONE', *, *, #11779, .T. ) ;
#13476=CARTESIAN_POINT ( 'NONE',  ( -34.08355720199904226, 2.371364769369340042, 7.455576670931136185 ) ) ;
#13486=CARTESIAN_POINT ( 'NONE',  ( -0.3370904143228963812, 0.2449105217885287067, 10.00000000000000000 ) ) ;
#13508=CARTESIAN_POINT ( 'NONE',  ( -18.67411147745623978, -27.51799019669813973, -3.760136334089591248 ) ) ;
#13520=CARTESIAN_POINT ( 'NONE',  ( 0.9600884595229846052, -0.8493647100668649808, 9.957892297621013356 ) ) ;
#13521=CARTESIAN_POINT ( 'NONE',  ( -36.70770892944847930, 7.840405911382138271, 6.057468652304065948 ) ) ;
#13524=CARTESIAN_POINT ( 'NONE',  ( -0.7479701569695257346, -0.9668092547116119428, 9.969517326150317160 ) ) ;
#13525=APPLICATION_CONTEXT ( 'automotive_design' ) ;
#13528=CARTESIAN_POINT ( 'NONE',  ( 1.780619886013945052, 1.041246721325614466, 9.886433018048068178 ) ) ;
#13531=CARTESIAN_POINT ( 'NONE',  ( 45.64490844644691236, 21.32281559348795952, 8.807470649214879543 ) ) ;
#13541=CARTESIAN_POINT ( 'NONE',  ( -9.999630309108516357, -0.09931773306744247354, 9.289350385289115053 ) ) ;
#13550=ORIENTED_EDGE ( 'NONE', *, *, #21784, .T. ) ;
#13553=ORIENTED_EDGE ( 'NONE', *, *, #37138, .F. ) ;
#13555=VECTOR ( 'NONE', #11110, 1000.000000000000227 ) ;
#13558=CARTESIAN_POINT ( 'NONE',  ( 0.3370904143228959926, -0.2449105217885284291, 10.00000000000000000 ) ) ;
#13575=CARTESIAN_POINT ( 'NONE',  ( 8.001683061421385190, 5.997755262142701937, 9.282506307616484875 ) ) ;
#13605=CARTESIAN_POINT ( 'NONE',  ( -50.11058929355264979, 7.578863168071929834, 7.455576670931136185 ) ) ;
#13623=ADVANCED_FACE ( 'NONE', ( #10139 ), #6791, .T. ) ;
#13624=CARTESIAN_POINT ( 'NONE',  ( -26.25702031264333058, 26.77347351953860155, 8.914903342594559632 ) ) ;
#13631=ORIENTED_EDGE ( 'NONE', *, *, #20926, .T. ) ;
#13633=CARTESIAN_POINT ( 'NONE',  ( 5.107674452598005566, -2.961810711067763169, 9.586754400234161366 ) ) ;
#13636=CARTESIAN_POINT ( 'NONE',  ( -24.19621561048240821, -28.69654500124497076, -5.338708898921617596 ) ) ;
#13641=B_SPLINE_CURVE_WITH_KNOTS ( 'NONE', 3,
 ( #26876, #50164, #42511, #7388 ),
 .UNSPECIFIED., .F., .F.,
 ( 4, 4 ),
 ( 0.0004299334430849200642, 0.0007706806524479787148 ),
 .UNSPECIFIED. ) ;
#13644=EDGE_CURVE ( 'NONE', #12217, #42650, #49095, .T. ) ;
#13648=CARTESIAN_POINT ( 'NONE',  ( 1.460157059060433360, -1.483633425177079745, 9.888808121373918070 ) ) ;
#13661=ORIENTED_EDGE ( 'NONE', *, *, #20982, .T. ) ;
#13664=ORIENTED_EDGE ( 'NONE', *, *, #30574, .T. ) ;
#13672=DIRECTION ( 'NONE',  ( 0.000000000000000000, 0.000000000000000000, -1.000000000000000000 ) ) ;
#13685=CARTESIAN_POINT ( 'NONE',  ( 1.011271242968694084, -0.7347315653655782652, -3.333333333333333481 ) ) ;
#13687=CARTESIAN_POINT ( 'NONE',  ( 49.67735855322978011, -8.912210285361751971, 8.356839323120299312 ) ) ;
#13691=CARTESIAN_POINT ( 'NONE',  ( -2.178343065408716139, -16.64136160116211727, -9.233365092205394475 ) ) ;
#13694=VERTEX_POINT ( 'NONE', #37375 ) ;
#13703=CARTESIAN_POINT ( 'NONE',  ( 0.6721397084974982672, 9.977385840602783773, 2.154851817814940063E-15 ) ) ;
#13710=CARTESIAN_POINT ( 'NONE',  ( -45.21167770612412085, -22.65616271077779942, 7.906207997025717304 ) ) ;
#13711=ADVANCED_FACE ( 'NONE', ( #4160 ), #35475, .F. ) ;
#13716=CARTESIAN_POINT ( 'NONE',  ( -0.1287570809895602630, -0.3962735484563142396, -10.00000000000000000 ) ) ;
#13731=CARTESIAN_POINT ( 'NONE',  ( 1.222012661920449439, -0.2471648704738783342, 9.981352469109934233 ) ) ;
#13737=CARTESIAN_POINT ( 'NONE',  ( 30.77287599203632951, 12.70002479445995824, 3.199614146704519602 ) ) ;
#13740=CARTESIAN_POINT ( 'NONE',  ( -44.99506233596265048, -23.32283626942287569, 7.455576670931136185 ) ) ;
#13742=CARTESIAN_POINT ( 'NONE',  ( 1.011271242968677653, 0.7347315653656002477, 3.333333333333333481 ) ) ;
#13748=CARTESIAN_POINT ( 'NONE',  ( 1.780619886013945052, 1.041246721325614466, 9.886433018048068178 ) ) ;
#13754=CARTESIAN_POINT ( 'NONE',  ( -1.249999999999999778, 0.000000000000000000, 10.00000000000000000 ) ) ;
#13756=CARTESIAN_POINT ( 'NONE',  ( 21.61731705588930907, 25.43568671410602278, -9.367992836599954742 ) ) ;
#13757=ORIENTED_EDGE ( 'NONE', *, *, #45371, .F. ) ;
#13764=VERTEX_POINT ( 'NONE', #7506 ) ;
#13768=EDGE_CURVE ( 'NONE', #49939, #36396, #3177, .T. ) ;
#13776=CARTESIAN_POINT ( 'NONE',  ( 33.14391172085757375, 37.72293746533119929, -8.016098858316199838 ) ) ;
#13783=B_SPLINE_CURVE_WITH_KNOTS ( 'NONE', 3,
 ( #2223, #33527, #29668, #45289, #5561, #45040 ),
 .UNSPECIFIED., .F., .F.,
 ( 4, 2, 4 ),
 ( 3.127317220692751144E-18, 0.009882509389272367203, 0.01976501877854473094 ),
 .UNSPECIFIED. ) ;
#13808=B_SPLINE_CURVE_WITH_KNOTS ( 'NONE', 3,
 ( #8186, #12274, #7940, #26912 ),
 .UNSPECIFIED., .F., .F.,
 ( 4, 4 ),
 ( 0.9890644561681873892, 1.000000000000000000 ),
 .UNSPECIFIED. ) ;
#13809=ORIENTED_EDGE ( 'NONE', *, *, #25295, .F. ) ;
#13812=VERTEX_POINT ( 'NONE', #32119 ) ;
#13820=B_SPLINE_SURFACE_WITH_KNOTS ( 'NONE', 3, 3, ( 
 ( #2292, #17193, #40294, #20781 ),
 ( #25653, #36461, #1303, #32864 ),
 ( #32604, #16950, #40544, #48188 ),
 ( #6147, #40795, #44367, #9487 ) ),
 .UNSPECIFIED., .F., .F., .F.,
 ( 4, 4 ),
 ( 4, 4 ),
 ( 0.000000000000000000, 1.000000000000000000 ),
 ( 0.000000000000000000, 1.000000000000000000 ),
 .UNSPECIFIED. ) ;
#13823=CARTESIAN_POINT ( 'NONE',  ( 1.250000000000000222, 0.000000000000000000, -10.00000000000000000 ) ) ;
#13833=CARTESIAN_POINT ( 'NONE',  ( -36.46533180484016157, -8.777022568848208195, -9.011255500499647297 ) ) ;
#13835=CARTESIAN_POINT ( 'NONE',  ( -0.9489147763969763005, 2.465022012282187536, 9.847478953136931779 ) ) ;
#13841=AXIS2_PLACEMENT_3D ( 'NONE', #43323, #32055, #47897 ) ;
#13844=CARTESIAN_POINT ( 'NONE',  ( -3.996390545799824334, 16.57371371864897469, 8.953103998512858652 ) ) ;
#13847=ORIENTED_EDGE ( 'NONE', *, *, #16062, .F. ) ;
#13850=CARTESIAN_POINT ( 'NONE',  ( -4.763548243873389154, 16.57409059453848599, 8.727788335465566760 ) ) ;
#13851=VERTEX_POINT ( 'NONE', #40572 ) ;
#13867=FACE_OUTER_BOUND ( 'NONE', #41845, .T. ) ;
#13868=VECTOR ( 'NONE', #29345, 1000.000000000000000 ) ;
#13877=B_SPLINE_CURVE_WITH_KNOTS ( 'NONE', 3,
 ( #29964, #14807, #37428, #18644 ),
 .UNSPECIFIED., .F., .F.,
 ( 4, 4 ),
 ( 8.673617379884035472E-19, 0.002458791966311098948 ),
 .UNSPECIFIED. ) ;
#13894=ADVANCED_FACE ( 'NONE', ( #48719 ), #1443, .T. ) ;
#13895=CARTESIAN_POINT ( 'NONE',  ( 0.2996946835594631597, 1.197003681518481910, 9.969907203203804968 ) ) ;
#13900=CARTESIAN_POINT ( 'NONE',  ( -14.48769039275601145, -30.44468701195584970, 8.807470649214879543 ) ) ;
#13912=CARTESIAN_POINT ( 'NONE',  ( -1.011271242968688533, 0.7347315653655859258, -10.00000000000000000 ) ) ;
#13926=CARTESIAN_POINT ( 'NONE',  ( 14.48769039275578407, 30.44468701195595983, 8.807470649214879543 ) ) ;
#13953=ORIENTED_EDGE ( 'NONE', *, *, #525, .F. ) ;
#13961=B_SPLINE_CURVE_WITH_KNOTS ( 'NONE', 3,
 ( #47634, #15619, #35401, #4332 ),
 .UNSPECIFIED., .F., .F.,
 ( 4, 4 ),
 ( 1.470203731559684877E-17, 0.0004072981213151955220 ),
 .UNSPECIFIED. ) ;
#13967=CARTESIAN_POINT ( 'NONE',  ( -0.9870575514055066613, -1.980598328282574316, 9.881002359080278907 ) ) ;
#13971=ADVANCED_FACE ( 'NONE', ( #45644 ), #14374, .F. ) ;
#13989=CARTESIAN_POINT ( 'NONE',  ( 1.011271242968688311, -0.7347315653655855927, 10.00000000000000000 ) ) ;
#14000=CARTESIAN_POINT ( 'NONE',  ( 6.875132362119187768, -50.00000000000000711, 8.356839323120299312 ) ) ;
#14004=ADVANCED_FACE ( 'NONE', ( #25422 ), #12884, .T. ) ;
#14006=CARTESIAN_POINT ( 'NONE',  ( 49.67735855322978011, -8.912210285361751971, 8.356839323120299312 ) ) ;
#14018=CARTESIAN_POINT ( 'NONE',  ( -17.23491422248386584, 0.5912720620001978844, 8.727788335465566760 ) ) ;
#14026=CARTESIAN_POINT ( 'NONE',  ( 21.58778298521313843, -25.34222074689757065, 3.199614146704519602 ) ) ;
#14044=ORIENTED_EDGE ( 'NONE', *, *, #20681, .T. ) ;
#14050=VECTOR ( 'NONE', #23242, 1000.000000000000114 ) ;
#14080=CARTESIAN_POINT ( 'NONE',  ( -0.8155877869437639927, -0.9072449372115535260, 9.963925895596188909 ) ) ;
#14082=ORIENTED_EDGE ( 'NONE', *, *, #32411, .F. ) ;
#14083=CARTESIAN_POINT ( 'NONE',  ( -8.277096487746778308, 33.14818118907697198, 7.455576670931136185 ) ) ;
#14096=CARTESIAN_POINT ( 'NONE',  ( -1.238491169206289877, -5.772936915099371014, 9.586754400234154261 ) ) ;
#14112=CARTESIAN_POINT ( 'NONE',  ( 1.104213410210670876, 0.6509177773818231039, 9.976582533991679824 ) ) ;
#14119=CARTESIAN_POINT ( 'NONE',  ( 2.277991179055260051, -9.750753554112558064, 3.092310436554651432 ) ) ;
#14121=CARTESIAN_POINT ( 'NONE',  ( -11.73320209285699889, 11.96063479729179768, 9.403735324607438884 ) ) ;
#14123=EDGE_CURVE ( 'NONE', #12977, #21718, #14765, .T. ) ;
#14134=CARTESIAN_POINT ( 'NONE',  ( -1.080000014127418639, -0.7606467978654640749, 9.943883492372872723 ) ) ;
#14137=CARTESIAN_POINT ( 'NONE',  ( -36.08557433729204433, 35.58569447144795106, 7.455576670931136185 ) ) ;
#14140=CARTESIAN_POINT ( 'NONE',  ( -31.46770792452106846, 38.94077080897363885, 3.199614146704519602 ) ) ;
#14150=ADVANCED_FACE ( 'NONE', ( #31050 ), #48080, .T. ) ;
#14154=CARTESIAN_POINT ( 'NONE',  ( -5.888214538810513154, -16.20866436362413410, 8.727788335465566760 ) ) ;
#14155=CARTESIAN_POINT ( 'NONE',  ( -1.270843316669170608, 0.6654759734677931915, 9.950105812514292936 ) ) ;
#14156=CARTESIAN_POINT ( 'NONE',  ( 0.6215990105956902267, -1.608617984725389860, 9.928159647716132241 ) ) ;
#14169=CARTESIAN_POINT ( 'NONE',  ( 1.468446590252912465, 0.3226319952343980058, 9.953784399990622589 ) ) ;
#14171=B_SPLINE_CURVE_WITH_KNOTS ( 'NONE', 3,
 ( #5855, #48651, #33072, #18402 ),
 .UNSPECIFIED., .F., .F.,
 ( 4, 4 ),
 ( 8.673617379884035472E-19, 0.002466147708923230146 ),
 .UNSPECIFIED. ) ;
#14174=CARTESIAN_POINT ( 'NONE',  ( 0.3862712429686727678, 1.188820645368945605, -10.00000000000000000 ) ) ;
#14178=CARTESIAN_POINT ( 'NONE',  ( 49.89397392339123627, -8.245536726716670373, 7.906207997025717304 ) ) ;
#14180=ORIENTED_EDGE ( 'NONE', *, *, #745, .T. ) ;
#14203=ORIENTED_EDGE ( 'NONE', *, *, #44353, .F. ) ;
#14219=EDGE_CURVE ( 'NONE', #3380, #12550, #38052, .T. ) ;
#14227=FACE_OUTER_BOUND ( 'NONE', #11477, .T. ) ;
#14231=CARTESIAN_POINT ( 'NONE',  ( 3.996390545799824334, -16.57371371864897469, 8.953103998512858652 ) ) ;
#14241=CARTESIAN_POINT ( 'NONE',  ( -29.61572577327014955, -16.11461842845715253, 8.807470649214879543 ) ) ;
#14242=CARTESIAN_POINT ( 'NONE',  ( -13.35436367797847801, -31.26996044524040741, 7.906207997025717304 ) ) ;
#14244=CARTESIAN_POINT ( 'NONE',  ( 37.19569680397832201, -4.820783179364443782, 8.100132398494510610 ) ) ;
#14247=PRODUCT_DEFINITION_SHAPE ( 'NONE', 'NONE',  #842 ) ;
#14254=CARTESIAN_POINT ( 'NONE',  ( -26.18032376592659105, 21.95228666728381128, 7.455576670931136185 ) ) ;
#14262=CARTESIAN_POINT ( 'NONE',  ( 33.86622497129647513, -3.037805405904928868, 7.906207997025717304 ) ) ;
#14263=CARTESIAN_POINT ( 'NONE',  ( -1.011271242968693862, 0.7347315653655780432, 3.333333333333333481 ) ) ;
#14265=CARTESIAN_POINT ( 'NONE',  ( 4.763548243873389154, -16.57409059453848599, 8.727788335465566760 ) ) ;
#14269=ORIENTED_EDGE ( 'NONE', *, *, #32772, .T. ) ;
#14281=EDGE_CURVE ( 'NONE', #48113, #18968, #14171, .T. ) ;
#14282=FACE_OUTER_BOUND ( 'NONE', #16402, .T. ) ;
#14283=ORIENTED_EDGE ( 'NONE', *, *, #26962, .F. ) ;
#14290=CARTESIAN_POINT ( 'NONE',  ( -3.231548175622898089, 9.463461120997347820, 9.282506307616472441 ) ) ;
#14294=VERTEX_POINT ( 'NONE', #9955 ) ;
#14301=CARTESIAN_POINT ( 'NONE',  ( -1.902009873419727048, -1.028513407865101037, 9.882710035074770971 ) ) ;
#14315=B_SPLINE_CURVE_WITH_KNOTS ( 'NONE', 3,
 ( #478, #31275, #27162, #11762 ),
 .UNSPECIFIED., .F., .F.,
 ( 4, 4 ),
 ( 0.000000000000000000, 0.2562577668812818232 ),
 .UNSPECIFIED. ) ;
#14319=FACE_OUTER_BOUND ( 'NONE', #6618, .T. ) ;
#14325=CARTESIAN_POINT ( 'NONE',  ( 11.73320209285708415, -11.96063479729170886, 9.403735324607438884 ) ) ;
#14329=ORIENTED_EDGE ( 'NONE', *, *, #7775, .T. ) ;
#14336=CARTESIAN_POINT ( 'NONE',  ( -1.193089574352124149, -0.2545860991493743564, 9.963925895596188909 ) ) ;
#14338=ORIENTED_EDGE ( 'NONE', *, *, #26656, .T. ) ;
#14348=CARTESIAN_POINT ( 'NONE',  ( 3.694521163055066282, 0.7694713829383740267, 9.865049507598753209 ) ) ;
#14349=CARTESIAN_POINT ( 'NONE',  ( 34.38425513258721367, -36.82177522737821107, 8.807470649214879543 ) ) ;
#14351=EDGE_CURVE ( 'NONE', #41656, #2158, #9266, .T. ) ;
#14352=CARTESIAN_POINT ( 'NONE',  ( -15.73090589902298042, -29.60029367929041655, 1.847720168420772691 ) ) ;
#14360=CARTESIAN_POINT ( 'NONE',  ( -1.011271242968683426, -0.7347315653655928092, -3.333333333333333481 ) ) ;
#14364=CARTESIAN_POINT ( 'NONE',  ( -32.57170742938676256, -18.58316106410400437, 7.697694107796192675 ) ) ;
#14369=B_SPLINE_CURVE_WITH_KNOTS ( 'NONE', 3,
 ( #3801, #12259, #20452, #46608 ),
 .UNSPECIFIED., .F., .F.,
 ( 4, 4 ),
 ( 0.003717760131171406711, 0.009855840391686850749 ),
 .UNSPECIFIED. ) ;
#14374=PLANE ( 'NONE',  #13037 ) ;
#14398=CARTESIAN_POINT ( 'NONE',  ( -0.8811857040074874137, -1.919576306124732401, 9.890170120223997330 ) ) ;
#14404=CARTESIAN_POINT ( 'NONE',  ( -2.053349722363707830, 0.3420258690445411864, 9.888808121373916293 ) ) ;
#14420=CARTESIAN_POINT ( 'NONE',  ( 5.781580041794017966, -8.177378108131177825, 3.215106848023477681 ) ) ;
#14424=B_SPLINE_CURVE_WITH_KNOTS ( 'NONE', 3,
 ( #5367, #36712, #28972, #21272 ),
 .UNSPECIFIED., .F., .F.,
 ( 4, 4 ),
 ( 0.9895749839358305433, 1.000000000000000000 ),
 .UNSPECIFIED. ) ;
#14431=CARTESIAN_POINT ( 'NONE',  ( -29.38926261462342993, -40.45084971874754132, 0.000000000000000000 ) ) ;
#14436=ORIENTED_EDGE ( 'NONE', *, *, #21761, .T. ) ;
#14447=CARTESIAN_POINT ( 'NONE',  ( 1.080000014128428498, 0.7606467978644730898, 9.943883492372853183 ) ) ;
#14476=CARTESIAN_POINT ( 'NONE',  ( -2.948105490345101387, -9.555557232197246620, 9.282506307616472441 ) ) ;
#14479=CARTESIAN_POINT ( 'NONE',  ( -24.47767542868268364, 23.18653802921800278, 8.807470649214879543 ) ) ;
#14492=CARTESIAN_POINT ( 'NONE',  ( 37.50000000000000000, 4.592425496802574367E-15, 10.00000000000000000 ) ) ;
#14497=VECTOR ( 'NONE', #6275, 1000.000000000000000 ) ;
#14500=CARTESIAN_POINT ( 'NONE',  ( 0.3862712429686894766, -1.188820645368940276, -10.00000000000000000 ) ) ;
#14511=EDGE_LOOP ( 'NONE', ( #4180, #27960, #16867 ) ) ;
#14512=CARTESIAN_POINT ( 'NONE',  ( -12.35406723005387875, 11.51001571518090039, 9.178419661560148768 ) ) ;
#14515=ORIENTED_EDGE ( 'NONE', *, *, #37787, .F. ) ;
#14519=CARTESIAN_POINT ( 'NONE',  ( -1.437255894074058515, 3.713052624461494755, 6.606856988583542645E-16 ) ) ;
#14536=CARTESIAN_POINT ( 'NONE',  ( -1.035950918207909632, -33.23661552194049307, -2.408242355805840784 ) ) ;
#14544=CARTESIAN_POINT ( 'NONE',  ( 0.1287570809895660084, -0.3962735484563127408, -10.00000000000000000 ) ) ;
#14549=CARTESIAN_POINT ( 'NONE',  ( -0.3862712429686895876, 1.188820645368940720, 10.00000000000000000 ) ) ;
#14562=B_SPLINE_SURFACE_WITH_KNOTS ( 'NONE', 3, 3, ( 
 ( #15675, #50012, #34435, #14920 ),
 ( #46937, #27487, #26464, #11323 ),
 ( #6967, #38296, #46688, #30835 ),
 ( #43130, #11584, #23629, #3105 ) ),
 .UNSPECIFIED., .F., .F., .F.,
 ( 4, 4 ),
 ( 4, 4 ),
 ( 0.000000000000000000, 1.000000000000000000 ),
 ( 0.000000000000000000, 1.000000000000000000 ),
 .UNSPECIFIED. ) ;
#14579=CARTESIAN_POINT ( 'NONE',  ( 22.69295089195473025, 45.31600496604705341, 7.455576670931136185 ) ) ;
#14584=CARTESIAN_POINT ( 'NONE',  ( 1.335416683881728739, -0.4035165624854742394, 9.955131761384823363 ) ) ;
#14587=ORIENTED_EDGE ( 'NONE', *, *, #20828, .F. ) ;
#14590=FACE_OUTER_BOUND ( 'NONE', #9476, .T. ) ;
#14602=CARTESIAN_POINT ( 'NONE',  ( 1.011271242968688311, -0.7347315653655855927, -3.333333333333333481 ) ) ;
#14607=B_SPLINE_CURVE_WITH_KNOTS ( 'NONE', 3,
 ( #24316, #8664, #28409, #7907 ),
 .UNSPECIFIED., .F., .F.,
 ( 4, 4 ),
 ( 0.000000000000000000, 0.001246897409371994052 ),
 .UNSPECIFIED. ) ;
#14609=CARTESIAN_POINT ( 'NONE',  ( -2.816440797479544234, 7.430518950465684114, 9.432811472610049819 ) ) ;
#14611=CARTESIAN_POINT ( 'NONE',  ( -23.31729631074215092, -24.19776167542410406, -8.016098858316199838 ) ) ;
#14615=CARTESIAN_POINT ( 'NONE',  ( -1.133908876584336367, -0.5183204401656656968, 9.981352469109934233 ) ) ;
#14621=ORIENTED_EDGE ( 'NONE', *, *, #38576, .F. ) ;
#14623=EDGE_CURVE ( 'NONE', #31155, #28209, #5531, .T. ) ;
#14634=EDGE_CURVE ( 'NONE', #20782, #29885, #3714, .T. ) ;
#14638=CARTESIAN_POINT ( 'NONE',  ( -34.38425513258695077, 36.82177522737848108, 8.807470649214879543 ) ) ;
#14639=CARTESIAN_POINT ( 'NONE',  ( 4.190615033700592740, 4.237471995405366343, 6.606856988583542645E-16 ) ) ;
#14644=CARTESIAN_POINT ( 'NONE',  ( -34.08355720199904226, 2.371364769369340042, 7.455576670931136185 ) ) ;
#14645=ADVANCED_FACE ( 'NONE', ( #24543 ), #40352, .T. ) ;
#14653=EDGE_LOOP ( 'NONE', ( #10666, #44479, #9725, #38091, #18046 ) ) ;
#14656=CARTESIAN_POINT ( 'NONE',  ( 25.61277432017878297, -22.36370378792834757, 7.906207997025717304 ) ) ;
#14671=CARTESIAN_POINT ( 'NONE',  ( 2.051144455471369810, 1.664205274803712831, 9.847478953136990398 ) ) ;
#14673=CARTESIAN_POINT ( 'NONE',  ( 0.3896797354184660667, -1.262193838292004155, 9.943883492372872723 ) ) ;
#14676=CARTESIAN_POINT ( 'NONE',  ( 1.011271242968683648, 0.7347315653655930312, 10.00000000000000000 ) ) ;
#14679=CARTESIAN_POINT ( 'NONE',  ( -0.3862712429686895876, 1.188820645368940720, 10.00000000000000000 ) ) ;
#14695=CARTESIAN_POINT ( 'NONE',  ( 14.86945752723346637, 7.944783388879009145, 2.590526750877053086 ) ) ;
#14701=ADVANCED_FACE ( 'NONE', ( #29904 ), #44421, .T. ) ;
#14714=CARTESIAN_POINT ( 'NONE',  ( 1.275927284277173834, -0.1224368140627448004, 9.976582533991679824 ) ) ;
#14717=B_SPLINE_CURVE_WITH_KNOTS ( 'NONE', 3,
 ( #37785, #36784, #41366, #17999 ),
 .UNSPECIFIED., .F., .F.,
 ( 4, 4 ),
 ( 5.938563236642406840E-16, 0.009782300387714819301 ),
 .UNSPECIFIED. ) ;
#14720=ORIENTED_EDGE ( 'NONE', *, *, #40067, .T. ) ;
#14724=CARTESIAN_POINT ( 'NONE',  ( -45.64490844644706868, -21.32281559348764333, 8.807470649214879543 ) ) ;
#14725=VERTEX_POINT ( 'NONE', #9896 ) ;
#14733=CARTESIAN_POINT ( 'NONE',  ( -25.61277432017861955, 22.36370378792854297, 7.906207997025717304 ) ) ;
#14735=CARTESIAN_POINT ( 'NONE',  ( 13.35436367797824353, 31.26996044524050333, 7.906207997025717304 ) ) ;
#14742=ADVANCED_FACE ( 'NONE', ( #25551 ), #36698, .T. ) ;
#14743=CARTESIAN_POINT ( 'NONE',  ( 0.5113015165352333691, 1.175527691268683395, 9.948547179989619238 ) ) ;
#14754=CARTESIAN_POINT ( 'NONE',  ( 26.18032376592674737, -21.95228666728361233, 7.455576670931136185 ) ) ;
#14755=CARTESIAN_POINT ( 'NONE',  ( -13.92102703536724384, -30.85732372859812500, 8.356839323120299312 ) ) ;
#14756=CARTESIAN_POINT ( 'NONE',  ( 17.51065725283126895, -28.41934970907778890, -9.367992836599954742 ) ) ;
#14761=CARTESIAN_POINT ( 'NONE',  ( -0.3862712429686809279, -1.188820645368943163, 10.00000000000000000 ) ) ;
#14762=CARTESIAN_POINT ( 'NONE',  ( 2.538055338523177440, 33.28424297489108596, -9.367992836599954742 ) ) ;
#14765=B_SPLINE_CURVE_WITH_KNOTS ( 'NONE', 3,
 ( #7699, #35422, #35165, #22828 ),
 .UNSPECIFIED., .F., .F.,
 ( 4, 4 ),
 ( 0.01010185847678718787, 0.01012833122192013588 ),
 .UNSPECIFIED. ) ;
#14770=CARTESIAN_POINT ( 'NONE',  ( -3.996390545799824334, 16.57371371864897469, 8.953103998512858652 ) ) ;
#14771=EDGE_LOOP ( 'NONE', ( #34337, #20149, #33278 ) ) ;
#14777=CARTESIAN_POINT ( 'NONE',  ( 0.5113015165352333691, 1.175527691268683395, 9.948547179989619238 ) ) ;
#14795=CARTESIAN_POINT ( 'NONE',  ( -4.641001526964560142, -50.00000000000000711, -8.016098858316199838 ) ) ;
#14806=CARTESIAN_POINT ( 'NONE',  ( 26.18032376592674737, -21.95228666728361233, 7.455576670931136185 ) ) ;
#14807=CARTESIAN_POINT ( 'NONE',  ( -37.09740935455761246, 5.526036232978498219, 8.506357886886741326 ) ) ;
#14809=B_SPLINE_CURVE_WITH_KNOTS ( 'NONE', 3,
 ( #31151, #6776, #26532, #30388 ),
 .UNSPECIFIED., .F., .F.,
 ( 4, 4 ),
 ( 8.940560153363745023E-19, 0.0003137973356796201589 ),
 .UNSPECIFIED. ) ;
#14816=FACE_OUTER_BOUND ( 'NONE', #4443, .T. ) ;
#14817=CARTESIAN_POINT ( 'NONE',  ( -0.2996946835593986558, -1.197003681518488794, 9.969907203203803192 ) ) ;
#14820=CARTESIAN_POINT ( 'NONE',  ( -1.011271242968688533, 0.7347315653655859258, 10.00000000000000000 ) ) ;
#14821=B_SPLINE_CURVE_WITH_KNOTS ( 'NONE', 3,
 ( #21602, #48762, #15372, #7673 ),
 .UNSPECIFIED., .F., .F.,
 ( 4, 4 ),
 ( 0.000000000000000000, 0.001249001129225746874 ),
 .UNSPECIFIED. ) ;
#14828=CARTESIAN_POINT ( 'NONE',  ( 0.3440687301471855308, 1.609937937016769460, 9.936700280135880803 ) ) ;
#14859=CARTESIAN_POINT ( 'NONE',  ( 21.58778298521313843, -25.34222074689757065, 3.199614146704519602 ) ) ;
#14865=B_SPLINE_CURVE_WITH_KNOTS ( 'NONE', 3,
 ( #33482, #45490, #6515, #22174 ),
 .UNSPECIFIED., .F., .F.,
 ( 4, 4 ),
 ( 0.000000000000000000, 2.804146970186931250E-05 ),
 .UNSPECIFIED. ) ;
#14873=CARTESIAN_POINT ( 'NONE',  ( -12.16428377685542017, -11.73151505502925929, -9.008049429158100807 ) ) ;
#14877=CARTESIAN_POINT ( 'NONE',  ( 48.99656738986517723, -11.00747004110342431, 1.847720168420772691 ) ) ;
#14878=CARTESIAN_POINT ( 'NONE',  ( -6.875132362119187768, 50.00000000000000711, 8.356839323120299312 ) ) ;
#14883=CARTESIAN_POINT ( 'NONE',  ( 34.08355720199905647, -2.371364769369109116, 7.455576670931136185 ) ) ;
#14887=ORIENTED_EDGE ( 'NONE', *, *, #21786, .F. ) ;
#14891=ADVANCED_FACE ( 'NONE', ( #39900 ), #25195, .T. ) ;
#14895=EDGE_LOOP ( 'NONE', ( #20552, #17447, #3783, #43235, #21957, #19647, #26719, #4216, #32220, #47821, #20117, #44388, #2891, #3316 ) ) ;
#14899=VERTEX_POINT ( 'NONE', #16283 ) ;
#14900=ORIENTED_EDGE ( 'NONE', *, *, #49125, .F. ) ;
#14901=CARTESIAN_POINT ( 'NONE',  ( -49.67735855322972327, 8.912210285362091255, 8.356839323120299312 ) ) ;
#14904=ORIENTED_EDGE ( 'NONE', *, *, #6986, .T. ) ;
#14914=CARTESIAN_POINT ( 'NONE',  ( 1.011271242968677653, 0.7347315653656002477, 10.00000000000000000 ) ) ;
#14915=CARTESIAN_POINT ( 'NONE',  ( 2.948105490344985480, 9.555557232197198658, 9.282506307616484875 ) ) ;
#14920=CARTESIAN_POINT ( 'NONE',  ( -1.011271242968688533, 0.7347315653655859258, 10.00000000000000000 ) ) ;
#14928=CARTESIAN_POINT ( 'NONE',  ( 24.39427009665984869, 44.07992421011656603, 8.807470649214879543 ) ) ;
#14932=CARTESIAN_POINT ( 'NONE',  ( 22.69295089195473736, 45.31600496604706052, 7.455576670931136185 ) ) ;
#14935=CARTESIAN_POINT ( 'NONE',  ( 48.34672127938079456, -13.00749071703866555, 3.199614146704519602 ) ) ;
#14938=ADVANCED_FACE ( 'NONE', ( #41645 ), #13301, .T. ) ;
#14939=CARTESIAN_POINT ( 'NONE',  ( 1.164014690938906416, -0.7287989552214911848, 9.946805383069625250 ) ) ;
#14940=CARTESIAN_POINT ( 'NONE',  ( -0.06526599240255732959, 1.373921316405938065, 9.972175347158398040 ) ) ;
#14941=ADVANCED_FACE ( 'NONE', ( #21635 ), #12569, .T. ) ;
#14945=ORIENTED_EDGE ( 'NONE', *, *, #999, .F. ) ;
#14953=B_SPLINE_CURVE_WITH_KNOTS ( 'NONE', 3,
 ( #13450, #17302, #45218, #33967 ),
 .UNSPECIFIED., .F., .F.,
 ( 4, 4 ),
 ( 0.000000000000000000, 0.2637263876330692147 ),
 .UNSPECIFIED. ) ;
#14958=CARTESIAN_POINT ( 'NONE',  ( -1.780619886013952602, -1.041246721325602920, 9.886433018048069954 ) ) ;
#14966=VERTEX_POINT ( 'NONE', #9340 ) ;
#14975=CARTESIAN_POINT ( 'NONE',  ( 1.249999999999999778, 0.000000000000000000, 3.333333333333333481 ) ) ;
#14994=ADVANCED_FACE ( 'NONE', ( #29095 ), #17288, .F. ) ;
#15001=B_SPLINE_SURFACE_WITH_KNOTS ( 'NONE', 3, 3, ( 
 ( #49956, #10750, #11009, #15376 ),
 ( #22551, #46115, #38487, #6398 ),
 ( #18945, #14859, #49710, #42309 ),
 ( #14349, #30510, #34127, #22807 ) ),
 .UNSPECIFIED., .F., .F., .F.,
 ( 4, 4 ),
 ( 4, 4 ),
 ( 0.000000000000000000, 1.000000000000000000 ),
 ( 0.000000000000000000, 1.000000000000000000 ),
 .UNSPECIFIED. ) ;
#15003=CARTESIAN_POINT ( 'NONE',  ( -32.36066692128246558, 7.813306791043033606, 3.199614146704519602 ) ) ;
#15006=CARTESIAN_POINT ( 'NONE',  ( -17.23491422248386584, 0.5912720620001978844, 8.727788335465566760 ) ) ;
#15012=CARTESIAN_POINT ( 'NONE',  ( 20.40054609052976531, -26.26366202847973597, -3.760136334089591248 ) ) ;
#15015=CARTESIAN_POINT ( 'NONE',  ( -0.9015506157965548217, 0.9804419706251666922, 9.951893257059996500 ) ) ;
#15018=ORIENTED_EDGE ( 'NONE', *, *, #37508, .T. ) ;
#15021=FACE_OUTER_BOUND ( 'NONE', #27255, .T. ) ;
#15024=ORIENTED_EDGE ( 'NONE', *, *, #26936, .T. ) ;
#15025=CARTESIAN_POINT ( 'NONE',  ( 45.64490844644691236, 21.32281559348795952, 8.807470649214879543 ) ) ;
#15026=CARTESIAN_POINT ( 'NONE',  ( 0.000000000000000000, 0.000000000000000000, 0.000000000000000000 ) ) ;
#15030=VERTEX_POINT ( 'NONE', #26498 ) ;
#15046=CARTESIAN_POINT ( 'NONE',  ( 46.10908423965007330, 19.89422939639137766, 1.847720168420772691 ) ) ;
#15050=CARTESIAN_POINT ( 'NONE',  ( -1.782521105131510186, 0.3635605703594341209, 9.903764339332088440 ) ) ;
#15052=CARTESIAN_POINT ( 'NONE',  ( 11.73320209285708415, -11.96063479729170886, 9.403735324607438884 ) ) ;
#15063=CARTESIAN_POINT ( 'NONE',  ( 30.25247992116058526, -39.82368563463805344, -3.760136334089591248 ) ) ;
#15065=B_SPLINE_CURVE_WITH_KNOTS ( 'NONE', 3,
 ( #45204, #44713, #10092, #13183 ),
 .UNSPECIFIED., .F., .F.,
 ( 4, 4 ),
 ( 0.9811748202683102660, 0.9878904167554123372 ),
 .UNSPECIFIED. ) ;
#15073=CARTESIAN_POINT ( 'NONE',  ( -0.3896797354171960270, 1.262193838292709147, 9.943883492372847854 ) ) ;
#15085=CARTESIAN_POINT ( 'NONE',  ( -50.11058929355266400, 7.578863168071933387, 7.455576670931136185 ) ) ;
#15093=EDGE_CURVE ( 'NONE', #12195, #25169, #12258, .T. ) ;
#15106=CARTESIAN_POINT ( 'NONE',  ( -0.4277546898749028381, -1.184419892831247711, 9.974012008644017158 ) ) ;
#15110=FACE_OUTER_BOUND ( 'NONE', #41997, .T. ) ;
#15116=CARTESIAN_POINT ( 'NONE',  ( -5.888214538810513154, -16.20866436362413410, 8.727788335465566760 ) ) ;
#15122=CARTESIAN_POINT ( 'NONE',  ( 1.057156451998911839, -0.7920882637786250680, 9.943883492372851407 ) ) ;
#15125=CARTESIAN_POINT ( 'NONE',  ( 16.69947034530964913, -2.312583065866261389, 2.590526750877053086 ) ) ;
#15156=FACE_OUTER_BOUND ( 'NONE', #48343, .T. ) ;
#15162=CARTESIAN_POINT ( 'NONE',  ( -21.60170755165869849, 30.69732439037094807, -6.568693074176340296 ) ) ;
#15164=CARTESIAN_POINT ( 'NONE',  ( 1.211050186583219279, 0.5544523570010763125, 9.951893257060014264 ) ) ;
#15168=DIRECTION ( 'NONE',  ( -0.000000000000000000, -0.000000000000000000, -1.000000000000000000 ) ) ;
#15176=CARTESIAN_POINT ( 'NONE',  ( 1.011271242968677653, 0.7347315653656002477, 10.00000000000000000 ) ) ;
#15177=VERTEX_POINT ( 'NONE', #11869 ) ;
#15187=CARTESIAN_POINT ( 'NONE',  ( -1.721971274562257515, -0.09408549481333014497, 9.928159647716187308 ) ) ;
#15203=CARTESIAN_POINT ( 'NONE',  ( 23.82716369509147825, 44.49195112876006419, 8.356839323120299312 ) ) ;
#15213=CARTESIAN_POINT ( 'NONE',  ( 4.256388337216338691, -5.377297509087402005, 9.753789706659947711 ) ) ;
#15219=ORIENTED_EDGE ( 'NONE', *, *, #43976, .T. ) ;
#15223=VECTOR ( 'NONE', #45712, 1000.000000000000000 ) ;
#15231=B_SPLINE_CURVE_WITH_KNOTS ( 'NONE', 3,
 ( #15904, #16398, #20253, #43337 ),
 .UNSPECIFIED., .F., .F.,
 ( 4, 4 ),
 ( 0.000000000000000000, 0.0001252128669263171171 ),
 .UNSPECIFIED. ) ;
#15235=EDGE_CURVE ( 'NONE', #13105, #31434, #48663, .T. ) ;
#15242=ORIENTED_EDGE ( 'NONE', *, *, #11243, .F. ) ;
#15244=ORIENTED_EDGE ( 'NONE', *, *, #10175, .F. ) ;
#15245=CARTESIAN_POINT ( 'NONE',  ( 1.011271242968683648, 0.7347315653655930312, 9.972675548442463622 ) ) ;
#15256=CARTESIAN_POINT ( 'NONE',  ( -48.99656738986512039, 11.00747004110376182, 1.847720168420772691 ) ) ;
#15262=CARTESIAN_POINT ( 'NONE',  ( -31.44259251615275019, -38.95901822126145220, -9.367992836599951190 ) ) ;
#15266=B_SPLINE_CURVE_WITH_KNOTS ( 'NONE', 3,
 ( #49740, #22592, #14639, #38274 ),
 .UNSPECIFIED., .F., .F.,
 ( 4, 4 ),
 ( 0.002800684175189303935, 0.008939195511151335274 ),
 .UNSPECIFIED. ) ;
#15279=CARTESIAN_POINT ( 'NONE',  ( -8.831420117243776957, -14.12636088103186260, -3.546734833711462365 ) ) ;
#15282=B_SPLINE_CURVE_WITH_KNOTS ( 'NONE', 3,
 ( #9745, #45377, #2302, #30268 ),
 .UNSPECIFIED., .F., .F.,
 ( 4, 4 ),
 ( 0.000000000000000000, 0.0002520763768916076618 ),
 .UNSPECIFIED. ) ;
#15286=CARTESIAN_POINT ( 'NONE',  ( 6.875132362119187768, -50.00000000000000711, 8.356839323120299312 ) ) ;
#15291=CARTESIAN_POINT ( 'NONE',  ( 29.39982726364966581, 16.78152490921169360, 8.356839323120299312 ) ) ;
#15293=CARTESIAN_POINT ( 'NONE',  ( 0.4166666666666669072, 0.000000000000000000, 10.00000000000000000 ) ) ;
#15300=EDGE_CURVE ( 'NONE', #9732, #29784, #20368, .T. ) ;
#15302=ORIENTED_EDGE ( 'NONE', *, *, #47892, .T. ) ;
#15316=CARTESIAN_POINT ( 'NONE',  ( 28.96803024440893992, 18.11533787072037072, 7.455576670931136185 ) ) ;
#15317=( LENGTH_UNIT ( ) NAMED_UNIT ( * ) SI_UNIT ( .MILLI., .METRE. ) );
#15324=CARTESIAN_POINT ( 'NONE',  ( 2.097937730060976946, -0.2450639578954889597, 9.884520316594379352 ) ) ;
#15328=CARTESIAN_POINT ( 'NONE',  ( 48.55374341718673747, 12.37034209168268006, -8.917361510505369182 ) ) ;
#15329=ORIENTED_EDGE ( 'NONE', *, *, #5278, .F. ) ;
#15341=CARTESIAN_POINT ( 'NONE',  ( -0.9602803029231570253, 0.8490247040095960651, 9.976582533991679824 ) ) ;
#15359=ORIENTED_EDGE ( 'NONE', *, *, #33357, .T. ) ;
#15360=FACE_OUTER_BOUND ( 'NONE', #44646, .T. ) ;
#15369=DIRECTION ( 'NONE',  ( 0.2599384441937727663, -0.8000082703740916124, 0.5407575913134972101 ) ) ;
#15372=CARTESIAN_POINT ( 'NONE',  ( 0.7769635690559215657, 0.3027738231833606020, 9.985671796968913938 ) ) ;
#15374=CARTESIAN_POINT ( 'NONE',  ( 9.999999999999998224, 1.843143693225357538E-15, 8.340239149798797769 ) ) ;
#15376=CARTESIAN_POINT ( 'NONE',  ( -1.011271242968677875, -0.7347315653656004697, -10.00000000000000000 ) ) ;
#15389=CARTESIAN_POINT ( 'NONE',  ( -0.1287570809895632329, 0.3962735484563137400, 10.00000000000000000 ) ) ;
#15391=CARTESIAN_POINT ( 'NONE',  ( 32.43949840348898306, 7.871562655726499713, -9.367992836599954742 ) ) ;
#15420=B_SPLINE_SURFACE_WITH_KNOTS ( 'NONE', 3, 3, ( 
 ( #40439, #47833, #12721, #4769 ),
 ( #28885, #44010, #17331, #39691 ),
 ( #16328, #20416, #31991, #6793 ),
 ( #25283, #25792, #26046, #9880 ) ),
 .UNSPECIFIED., .F., .F., .F.,
 ( 4, 4 ),
 ( 4, 4 ),
 ( 0.000000000000000000, 1.000000000000000000 ),
 ( 0.000000000000000000, 1.000000000000000000 ),
 .UNSPECIFIED. ) ;
#15422=CYLINDRICAL_SURFACE ( 'NONE', #16104, 37.50000000000000000 ) ;
#15427=CARTESIAN_POINT ( 'NONE',  ( 15.62858259096121216, -5.755205073598614440, -9.683996418299976483 ) ) ;
#15440=CARTESIAN_POINT ( 'NONE',  ( 50.11058929355269953, -7.578863168071589662, 7.455576670931136185 ) ) ;
#15448=CARTESIAN_POINT ( 'NONE',  ( -6.508636631827791064, -15.75743548351446854, 8.953103998512858652 ) ) ;
#15458=B_SPLINE_CURVE_WITH_KNOTS ( 'NONE', 3,
 ( #14156, #26232, #45942, #14673 ),
 .UNSPECIFIED., .F., .F.,
 ( 4, 4 ),
 ( 1.093182292142470417E-15, 0.0004154657329505190787 ),
 .UNSPECIFIED. ) ;
#15467=ORIENTED_EDGE ( 'NONE', *, *, #44632, .F. ) ;
#15474=ORIENTED_EDGE ( 'NONE', *, *, #25946, .F. ) ;
#15475=CARTESIAN_POINT ( 'NONE',  ( -16.02661358026017879, -4.530191650547607196, -9.683996418299976483 ) ) ;
#15486=CARTESIAN_POINT ( 'NONE',  ( -40.86389006639098653, -8.513139889764316237, -8.080361901872240793 ) ) ;
#15489=CARTESIAN_POINT ( 'NONE',  ( -1.468446590252919348, -0.3226319952343834063, 9.953784399990620813 ) ) ;
#15491=CYLINDRICAL_SURFACE ( 'NONE', #21752, 10.00000000000000000 ) ;
#15501=CARTESIAN_POINT ( 'NONE',  ( -33.08717642956897009, -5.870837526464928402, -8.016098858316199838 ) ) ;
#15505=EDGE_CURVE ( 'NONE', #21893, #13072, #5094, .T. ) ;
#15512=CIRCLE ( 'NONE', #36866, 37.50000000000000000 ) ;
#15527=CARTESIAN_POINT ( 'NONE',  ( 2.462075149652696027, -16.57295996686994499, 9.403735324607438884 ) ) ;
#15535=ORIENTED_EDGE ( 'NONE', *, *, #22070, .F. ) ;
#15541=CARTESIAN_POINT ( 'NONE',  ( -16.52264463346130796, 2.779753662172870232, 9.403735324607438884 ) ) ;
#15544=EDGE_LOOP ( 'NONE', ( #31972, #30060, #50586, #7176, #43121 ) ) ;
#15546=CARTESIAN_POINT ( 'NONE',  ( 6.174150299305392053, -33.14591993373988998, 8.807470649214879543 ) ) ;
#15552=EDGE_CURVE ( 'NONE', #19482, #6876, #48443, .T. ) ;
#15558=VERTEX_POINT ( 'NONE', #39965 ) ;
#15574=CARTESIAN_POINT ( 'NONE',  ( -0.3862712429686809279, -1.188820645368943163, 10.00000000000000000 ) ) ;
#15581=AXIS2_PLACEMENT_3D ( 'NONE', #33007, #17839, #10142 ) ;
#15595=EDGE_LOOP ( 'NONE', ( #26883, #1599, #15244 ) ) ;
#15599=CARTESIAN_POINT ( 'NONE',  ( 0.000000000000000000, 0.000000000000000000, 0.000000000000000000 ) ) ;
#15611=ORIENTED_EDGE ( 'NONE', *, *, #15854, .F. ) ;
#15613=CARTESIAN_POINT ( 'NONE',  ( -2.961022939495062900, 16.59676755884084187, 2.590526750877053086 ) ) ;
#15615=CARTESIAN_POINT ( 'NONE',  ( -0.3862712429686895876, 1.188820645368940720, 10.00000000000000000 ) ) ;
#15619=CARTESIAN_POINT ( 'NONE',  ( 1.862232582514315338, 0.9302239440314843399, 9.888808121373909188 ) ) ;
#15648=ORIENTED_EDGE ( 'NONE', *, *, #35405, .T. ) ;
#15658=CIRCLE ( 'NONE', #23004, 10.00000000000000000 ) ;
#15662=CARTESIAN_POINT ( 'NONE',  ( -1.250000000000000222, 0.000000000000000000, -10.00000000000000000 ) ) ;
#15665=DIRECTION ( 'NONE',  ( -0.4374820812098839107, 0.3178493372392718896, -0.8411784753765542133 ) ) ;
#15675=CARTESIAN_POINT ( 'NONE',  ( -24.39427009666018265, -44.07992421011638129, 8.807470649214879543 ) ) ;
#15676=CARTESIAN_POINT ( 'NONE',  ( 45.42829307628542779, 21.98948915213303579, 8.356839323120299312 ) ) ;
#15678=CARTESIAN_POINT ( 'NONE',  ( -34.95136153415531766, 36.40974830873496870, 8.356839323120299312 ) ) ;
#15684=CARTESIAN_POINT ( 'NONE',  ( -1.211301556933465751, -0.1727733738854601298, 9.993783931180535873 ) ) ;
#15686=CARTESIAN_POINT ( 'NONE',  ( 1.057156451998911839, -0.7920882637786250680, 9.943883492372851407 ) ) ;
#15691=CARTESIAN_POINT ( 'NONE',  ( -34.08355720199904226, 2.371364769369340042, 7.455576670931136185 ) ) ;
#15693=CARTESIAN_POINT ( 'NONE',  ( 2.097926912204255867, -0.2448757052703989245, 9.890170120223999106 ) ) ;
#15704=B_SPLINE_CURVE_WITH_KNOTS ( 'NONE', 3,
 ( #35974, #27506, #20558, #818 ),
 .UNSPECIFIED., .F., .F.,
 ( 4, 4 ),
 ( 0.01012863361515566052, 0.01015667504234235748 ),
 .UNSPECIFIED. ) ;
#15711=CARTESIAN_POINT ( 'NONE',  ( -0.8285222815141961572, -1.889008401827320771, 9.886433018048073507 ) ) ;
#15717=B_SPLINE_CURVE_WITH_KNOTS ( 'NONE', 3,
 ( #3375, #25992, #41630, #6476 ),
 .UNSPECIFIED., .F., .F.,
 ( 4, 4 ),
 ( 0.002354859187796704348, 0.002825807655362034231 ),
 .UNSPECIFIED. ) ;
#15722=CARTESIAN_POINT ( 'NONE',  ( 1.019713130072856355, 3.848720492505100843, 4.370690007832189750E-16 ) ) ;
#15726=CARTESIAN_POINT ( 'NONE',  ( -5.888214538810513154, -16.20866436362413410, 8.727788335465566760 ) ) ;
#15731=DIRECTION ( 'NONE',  ( -0.000000000000000000, -0.000000000000000000, -1.000000000000000000 ) ) ;
#15736=B_SPLINE_CURVE_WITH_KNOTS ( 'NONE', 3,
 ( #25335, #5573, #1985, #1491 ),
 .UNSPECIFIED., .F., .F.,
 ( 4, 4 ),
 ( 0.0002936521407522070222, 0.0006663369986142620403 ),
 .UNSPECIFIED. ) ;
#15746=CARTESIAN_POINT ( 'NONE',  ( 23.82716369509147825, 44.49195112876006419, 8.356839323120299312 ) ) ;
#15748=CARTESIAN_POINT ( 'NONE',  ( 1.249999999999999778, -0.000000000000000000, -10.00000000000000000 ) ) ;
#15749=CARTESIAN_POINT ( 'NONE',  ( -26.25702031264333058, 26.77347351953860155, 8.914903342594559632 ) ) ;
#15757=CARTESIAN_POINT ( 'NONE',  ( -34.08355720199904226, 2.371364769369340042, 7.455576670931136185 ) ) ;
#15766=CARTESIAN_POINT ( 'NONE',  ( -21.61731705588949737, -25.43568671410585935, -9.367992836599954742 ) ) ;
#15767=CARTESIAN_POINT ( 'NONE',  ( 9.696760411815720460, 2.443938934556958653, 0.000000000000000000 ) ) ;
#15768=EDGE_CURVE ( 'NONE', #9775, #22165, #44258, .T. ) ;
#15773=CARTESIAN_POINT ( 'NONE',  ( 1.080000014128428498, 0.7606467978644730898, 9.943883492372853183 ) ) ;
#15774=FACE_OUTER_BOUND ( 'NONE', #10674, .T. ) ;
#15794=EDGE_CURVE ( 'NONE', #30045, #26155, #44204, .T. ) ;
#15795=CARTESIAN_POINT ( 'NONE',  ( 1.337801958641917199, 1.088266084286984015, 9.928159647716135794 ) ) ;
#15813=CARTESIAN_POINT ( 'NONE',  ( -1.011271242968683426, -0.7347315653655928092, 10.00000000000000000 ) ) ;
#15826=CARTESIAN_POINT ( 'NONE',  ( -0.1287570809895602630, -0.3962735484563142396, 10.00000000000000000 ) ) ;
#15827=CARTESIAN_POINT ( 'NONE',  ( 8.294258456918035094, 5.607426633512224257, 6.185594734181536936 ) ) ;
#15829=ADVANCED_FACE ( 'NONE', ( #15774 ), #27312, .T. ) ;
#15841=B_SPLINE_SURFACE_WITH_KNOTS ( 'NONE', 3, 3, ( 
 ( #40497, #1746, #5581, #21236 ),
 ( #43822, #993, #36926, #47891 ),
 ( #9691, #736, #5336, #48640 ),
 ( #13531, #16380, #32049, #28192 ) ),
 .UNSPECIFIED., .F., .F., .F.,
 ( 4, 4 ),
 ( 4, 4 ),
 ( 0.000000000000000000, 1.000000000000000000 ),
 ( 0.000000000000000000, 1.000000000000000000 ),
 .UNSPECIFIED. ) ;
#15843=VERTEX_POINT ( 'NONE', #34530 ) ;
#15847=DIRECTION ( 'NONE',  ( -0.6805276818820436002, 0.4944323023722021482, 0.5407575913134970991 ) ) ;
#15848=CARTESIAN_POINT ( 'NONE',  ( -45.35314062630780541, 8.244242869019066333, 8.807470649214881320 ) ) ;
#15850=CARTESIAN_POINT ( 'NONE',  ( 0.5349929392774247505, 3.214704144639360717, 9.799351690761062272 ) ) ;
#15853=CARTESIAN_POINT ( 'NONE',  ( 9.999999999999994671, -1.084202172485504187E-16, 9.303249460322209785 ) ) ;
#15854=EDGE_CURVE ( 'NONE', #8731, #14966, #30136, .T. ) ;
#15861=ORIENTED_EDGE ( 'NONE', *, *, #7758, .T. ) ;
#15870=ADVANCED_FACE ( 'NONE', ( #15021 ), #694, .T. ) ;
#15873=CARTESIAN_POINT ( 'NONE',  ( -45.64490844644706868, -21.32281559348764333, 8.807470649214879543 ) ) ;
#15876=CARTESIAN_POINT ( 'NONE',  ( 8.277096487746778308, -50.00000000000000711, 7.455576670931136185 ) ) ;
#15877=CARTESIAN_POINT ( 'NONE',  ( -1.151763129092706617, 0.4096856258255360261, 9.987567862361069970 ) ) ;
#15879=CARTESIAN_POINT ( 'NONE',  ( -0.08756411783990718234, 1.703854692066548937, 9.912102921405034905 ) ) ;
#15891=CARTESIAN_POINT ( 'NONE',  ( -0.9494396179258391966, 9.954826186926261755, 9.646707543097345905 ) ) ;
#15894=B_SPLINE_CURVE_WITH_KNOTS ( 'NONE', 3,
 ( #46663, #11562, #32075, #27465 ),
 .UNSPECIFIED., .F., .F.,
 ( 4, 4 ),
 ( 0.000000000000000000, 0.0002520763768916294543 ),
 .UNSPECIFIED. ) ;
#15897=EDGE_LOOP ( 'NONE', ( #13847, #3473, #48075 ) ) ;
#15899=CARTESIAN_POINT ( 'NONE',  ( 16.76006782980217125, -2.050259795448531541, 9.178419661560148768 ) ) ;
#15904=CARTESIAN_POINT ( 'NONE',  ( -1.249999999999999778, 0.000000000000000000, 9.972675548442463622 ) ) ;
#15906=ORIENTED_EDGE ( 'NONE', *, *, #37617, .T. ) ;
#15914=CARTESIAN_POINT ( 'NONE',  ( 0.9342145181057528447, 1.950058884269514126, 9.882709995651168811 ) ) ;
#15917=ORIENTED_EDGE ( 'NONE', *, *, #42536, .T. ) ;
#15932=CARTESIAN_POINT ( 'NONE',  ( 34.08406891383362591, -15.63733501198463038, -8.192531242611266862 ) ) ;
#15936=ADVANCED_FACE ( 'NONE', ( #642 ), #4783, .T. ) ;
#15941=CARTESIAN_POINT ( 'NONE',  ( 44.99506233596247995, 23.32283626942318833, 7.455576670931136185 ) ) ;
#15943=ADVANCED_FACE ( 'NONE', ( #39647 ), #35111, .T. ) ;
#15952=CARTESIAN_POINT ( 'NONE',  ( 1.104609456715839766, 0.6504863887005235545, 9.948547179989622791 ) ) ;
#15955=CARTESIAN_POINT ( 'NONE',  ( 6.010192544690008631, -37.05120237258827132, 4.835783797351798974 ) ) ;
#15962=B_SPLINE_CURVE_WITH_KNOTS ( 'NONE', 3,
 ( #7619, #24031, #39940, #3760 ),
 .UNSPECIFIED., .F., .F.,
 ( 4, 4 ),
 ( 5.776111876705087994E-18, 0.0004301978946275169255 ),
 .UNSPECIFIED. ) ;
#15964=CARTESIAN_POINT ( 'NONE',  ( -1.011271242968688533, 0.7347315653655859258, 10.00000000000000000 ) ) ;
#15988=CARTESIAN_POINT ( 'NONE',  ( 0.1425549192113746144, -1.238581250503543618, 9.981352469109934233 ) ) ;
#16008=EDGE_LOOP ( 'NONE', ( #22004, #11307, #32065, #12636 ) ) ;
#16009=CARTESIAN_POINT ( 'NONE',  ( 9.386495789655688426, 3.489743738556303487, 6.429802539306412434 ) ) ;
#16018=CARTESIAN_POINT ( 'NONE',  ( 1.158497635116737312, -16.61944452314319420, -3.546734833711462365 ) ) ;
#16031=ADVANCED_FACE ( 'NONE', ( #21646 ), #47347, .T. ) ;
#16032=VERTEX_POINT ( 'NONE', #1654 ) ;
#16034=CARTESIAN_POINT ( 'NONE',  ( 4.672045878990125800, -33.19353511768168374, 1.847720168420772691 ) ) ;
#16039=EDGE_LOOP ( 'NONE', ( #3029, #1541, #38943, #21564 ) ) ;
#16040=EDGE_LOOP ( 'NONE', ( #42923, #23853, #38692 ) ) ;
#16042=CARTESIAN_POINT ( 'NONE',  ( 6.508636631827673824, 15.75743548351451295, 8.953103998512858652 ) ) ;
#16047=CARTESIAN_POINT ( 'NONE',  ( 12.35406723005396046, -11.51001571518080624, 9.178419661560148768 ) ) ;
#16060=ORIENTED_EDGE ( 'NONE', *, *, #3608, .F. ) ;
#16062=EDGE_CURVE ( 'NONE', #30045, #3402, #22204, .T. ) ;
#16067=CARTESIAN_POINT ( 'NONE',  ( -0.1287570809895576818, -0.3962735484563154609, 10.00000000000000000 ) ) ;
#16082=CARTESIAN_POINT ( 'NONE',  ( -6.174150299305392053, 50.00000000000000711, 8.807470649214879543 ) ) ;
#16097=CARTESIAN_POINT ( 'NONE',  ( 47.87295225382209907, 14.46560184742433641, -2.408242355805840784 ) ) ;
#16098=B_SPLINE_CURVE_WITH_KNOTS ( 'NONE', 3,
 ( #20924, #13216, #39934, #12460 ),
 .UNSPECIFIED., .F., .F.,
 ( 4, 4 ),
 ( 0.001937412222931639196, 0.003978261222106111578 ),
 .UNSPECIFIED. ) ;
#16104=AXIS2_PLACEMENT_3D ( 'NONE', #6703, #15168, #18240 ) ;
#16106=CARTESIAN_POINT ( 'NONE',  ( 1.780432407520001536, 1.041450996408479046, 9.894754715216729224 ) ) ;
#16123=ORIENTED_EDGE ( 'NONE', *, *, #15505, .F. ) ;
#16128=CARTESIAN_POINT ( 'NONE',  ( -0.1287570809895632329, 0.3962735484563137400, 10.00000000000000000 ) ) ;
#16140=B_SPLINE_CURVE_WITH_KNOTS ( 'NONE', 3,
 ( #3346, #33910, #14398, #45668 ),
 .UNSPECIFIED., .F., .F.,
 ( 4, 4 ),
 ( 0.9688112071879405596, 0.9724175925769215079 ),
 .UNSPECIFIED. ) ;
#16147=EDGE_CURVE ( 'NONE', #11134, #11547, #32567, .T. ) ;
#16149=CARTESIAN_POINT ( 'NONE',  ( -49.89397392339119364, 8.245536726717011433, 7.906207997025717304 ) ) ;
#16151=EDGE_LOOP ( 'NONE', ( #34822, #50305, #38321, #15302 ) ) ;
#16152=CARTESIAN_POINT ( 'NONE',  ( -0.7601424845489993531, 1.297311920617006065, 9.927319414211224213 ) ) ;
#16159=CARTESIAN_POINT ( 'NONE',  ( 0.7601424845489945792, -1.297311920616997627, 9.927319414211225990 ) ) ;
#16161=EDGE_CURVE ( 'NONE', #34526, #16183, #41721, .T. ) ;
#16164=ORIENTED_EDGE ( 'NONE', *, *, #12224, .T. ) ;
#16173=PLANE ( 'NONE',  #46171 ) ;
#16175=EDGE_CURVE ( 'NONE', #31056, #12217, #20916, .T. ) ;
#16181=CARTESIAN_POINT ( 'NONE',  ( -0.3862712429686895876, 1.188820645368940720, 10.00000000000000000 ) ) ;
#16183=VERTEX_POINT ( 'NONE', #31127 ) ;
#16189=FACE_OUTER_BOUND ( 'NONE', #18757, .T. ) ;
#16193=CARTESIAN_POINT ( 'NONE',  ( 15.00099850811936264, 7.462898891544210933, 9.403735324607438884 ) ) ;
#16194=EDGE_CURVE ( 'NONE', #566, #44892, #1737, .T. ) ;
#16200=CARTESIAN_POINT ( 'NONE',  ( -9.260964247899874380, 13.84230907185616744, -9.683996418299976483 ) ) ;
#16202=CARTESIAN_POINT ( 'NONE',  ( 28.52604530808654815, 41.07801380285680892, -3.760136334089591248 ) ) ;
#16205=B_SPLINE_CURVE_WITH_KNOTS ( 'NONE', 3,
 ( #43818, #19461, #27678, #38189 ),
 .UNSPECIFIED., .F., .F.,
 ( 4, 4 ),
 ( 1.734723475976807094E-18, 2.647279941188286807E-05 ),
 .UNSPECIFIED. ) ;
#16220=ORIENTED_EDGE ( 'NONE', *, *, #3976, .T. ) ;
#16229=CARTESIAN_POINT ( 'NONE',  ( 16.99749102614301677, -1.320765928724307425, 8.953103998512858652 ) ) ;
#16237=CARTESIAN_POINT ( 'NONE',  ( 0.000000000000000000, 0.000000000000000000, 0.000000000000000000 ) ) ;
#16256=CARTESIAN_POINT ( 'NONE',  ( 0.3862712429686894766, -1.188820645368940276, 3.333333333333333481 ) ) ;
#16267=B_SPLINE_SURFACE_WITH_KNOTS ( 'NONE', 3, 3, ( 
 ( #12947, #28604, #8858, #36080 ),
 ( #12704, #16563, #28365, #35578 ),
 ( #32222, #47315, #31729, #43995 ),
 ( #414, #27867, #20912, #36334 ) ),
 .UNSPECIFIED., .F., .F., .F.,
 ( 4, 4 ),
 ( 4, 4 ),
 ( 0.000000000000000000, 1.000000000000000000 ),
 ( 0.000000000000000000, 1.000000000000000000 ),
 .UNSPECIFIED. ) ;
#16274=VERTEX_POINT ( 'NONE', #15245 ) ;
#16275=CARTESIAN_POINT ( 'NONE',  ( -0.3440687301471724857, -1.609937937016752585, 9.936700280135882579 ) ) ;
#16280=EDGE_LOOP ( 'NONE', ( #9364, #28253 ) ) ;
#16283=CARTESIAN_POINT ( 'NONE',  ( 36.97942854200454832, -6.226705766838405154, 8.914903342594563185 ) ) ;
#16284=CARTESIAN_POINT ( 'NONE',  ( 1.011271242968688311, -0.7347315653655855927, -3.333333333333333481 ) ) ;
#16294=VERTEX_POINT ( 'NONE', #102 ) ;
#16296=CARTESIAN_POINT ( 'NONE',  ( -0.3910393408547386818, -3.877122853643371947, 9.741991644047244492 ) ) ;
#16297=CARTESIAN_POINT ( 'NONE',  ( 25.61277432017878297, -22.36370378792834757, 7.906207997025717304 ) ) ;
#16310=CARTESIAN_POINT ( 'NONE',  ( -8.831420117243776957, -14.12636088103186260, -3.546734833711462365 ) ) ;
#16322=FACE_OUTER_BOUND ( 'NONE', #44001, .T. ) ;
#16328=CARTESIAN_POINT ( 'NONE',  ( -31.46770792452106846, 38.94077080897363885, 3.199614146704519602 ) ) ;
#16336=VERTEX_POINT ( 'NONE', #8558 ) ;
#16354=B_SPLINE_CURVE_WITH_KNOTS ( 'NONE', 3,
 ( #45191, #37556, #50284, #22376 ),
 .UNSPECIFIED., .F., .F.,
 ( 4, 4 ),
 ( 0.000000000000000000, 0.0004072981213154963339 ),
 .UNSPECIFIED. ) ;
#16359=CARTESIAN_POINT ( 'NONE',  ( -10.30302290646040575, -13.08520913973572419, -9.683996418299976483 ) ) ;
#16362=CARTESIAN_POINT ( 'NONE',  ( 25.04522487443081502, -22.77512090857307925, 8.356839323120299312 ) ) ;
#16375=CARTESIAN_POINT ( 'NONE',  ( 6.174150299305392053, -33.14591993373988998, 8.807470649214879543 ) ) ;
#16377=CARTESIAN_POINT ( 'NONE',  ( 0.000000000000000000, 0.000000000000000000, 10.00000000000000000 ) ) ;
#16380=CARTESIAN_POINT ( 'NONE',  ( 29.61572577327002520, 16.11461842845735859, 8.807470649214879543 ) ) ;
#16384=CARTESIAN_POINT ( 'NONE',  ( -0.8808108730257375729, -0.8497440890243460609, 9.966990753365125855 ) ) ;
#16390=FACE_OUTER_BOUND ( 'NONE', #10603, .T. ) ;
#16394=CARTESIAN_POINT ( 'NONE',  ( -1.468624871022813583, -0.3222420739259539979, 9.936141075690077429 ) ) ;
#16396=CARTESIAN_POINT ( 'NONE',  ( -21.61731705588949382, -25.43568671410586290, -9.367992836599951190 ) ) ;
#16398=CARTESIAN_POINT ( 'NONE',  ( -1.258633725701695294, 0.04081300982073285399, 9.974012008644017158 ) ) ;
#16402=EDGE_LOOP ( 'NONE', ( #36508, #40788, #38687, #46151 ) ) ;
#16412=EDGE_CURVE ( 'NONE', #12217, #15843, #3832, .T. ) ;
#16413=DIRECTION ( 'NONE',  ( -1.000000000000000000, 0.000000000000000000, -0.000000000000000000 ) ) ;
#16414=EDGE_CURVE ( 'NONE', #48161, #2701, #22196, .T. ) ;
#16425=VERTEX_POINT ( 'NONE', #29059 ) ;
#16429=CARTESIAN_POINT ( 'NONE',  ( 27.73884755486784570, -25.23502201956245017, 7.697694107796188234 ) ) ;
#16434=B_SPLINE_CURVE_WITH_KNOTS ( 'NONE', 3,
 ( #17699, #21805, #33368, #5135 ),
 .UNSPECIFIED., .F., .F.,
 ( 4, 4 ),
 ( 7.273049277091620462E-19, 0.0002708531562905798062 ),
 .UNSPECIFIED. ) ;
#16435=CARTESIAN_POINT ( 'NONE',  ( 23.79193388295309219, 28.98609808355011452, -9.422646554964176246 ) ) ;
#16439=ADVANCED_FACE ( 'NONE', ( #860 ), #1864, .F. ) ;
#16444=CARTESIAN_POINT ( 'NONE',  ( -2.052560157877107994, 0.2040521727611285530, 9.891980816076527461 ) ) ;
#16447=CARTESIAN_POINT ( 'NONE',  ( -25.04522487443065160, 22.77512090857326754, 8.356839323120299312 ) ) ;
#16455=CARTESIAN_POINT ( 'NONE',  ( 18.67411147745603373, 27.51799019669827473, -3.760136334089591248 ) ) ;
#16463=ORIENTED_EDGE ( 'NONE', *, *, #10197, .T. ) ;
#16466=FACE_OUTER_BOUND ( 'NONE', #18904, .T. ) ;
#16468=EDGE_CURVE ( 'NONE', #12217, #4426, #14821, .T. ) ;
#16469=CARTESIAN_POINT ( 'NONE',  ( -0.3370904143228927730, -0.2449105217885335917, 10.00000000000000000 ) ) ;
#16482=CARTESIAN_POINT ( 'NONE',  ( 9.998889670239195837, 0.1490146381531976816, 9.282506307616472441 ) ) ;
#16496=CARTESIAN_POINT ( 'NONE',  ( -0.3862712429686809279, -1.188820645368943163, 10.00000000000000000 ) ) ;
#16499=CARTESIAN_POINT ( 'NONE',  ( -1.158497635116737312, 16.61944452314319420, -3.546734833711462365 ) ) ;
#16510=EDGE_CURVE ( 'NONE', #2282, #36948, #12366, .T. ) ;
#16531=ORIENTED_EDGE ( 'NONE', *, *, #3975, .F. ) ;
#16538=CARTESIAN_POINT ( 'NONE',  ( -0.4166666666666664631, 0.000000000000000000, -10.00000000000000000 ) ) ;
#16539=CARTESIAN_POINT ( 'NONE',  ( -33.08717642956897009, -5.870837526464928402, -8.016098858316199838 ) ) ;
#16540=FACE_OUTER_BOUND ( 'NONE', #21084, .T. ) ;
#16542=VERTEX_POINT ( 'NONE', #4073 ) ;
#16546=CARTESIAN_POINT ( 'NONE',  ( -0.3862712429686729343, -1.188820645368946050, -10.00000000000000000 ) ) ;
#16559=CARTESIAN_POINT ( 'NONE',  ( -28.55116071645519327, 41.05976639056880373, -2.408242355805840784 ) ) ;
#16563=CARTESIAN_POINT ( 'NONE',  ( -1.035950918207909632, -33.23661552194049307, -2.408242355805840784 ) ) ;
#16575=CARTESIAN_POINT ( 'NONE',  ( -1.760168014277137649, -0.8403809255486067720, 9.896382706792437034 ) ) ;
#16580=EDGE_CURVE ( 'NONE', #12217, #5524, #35655, .T. ) ;
#16588=CARTESIAN_POINT ( 'NONE',  ( 0.9983599181300923942, 1.124146016603553733, 9.953784399990620813 ) ) ;
#16591=CARTESIAN_POINT ( 'NONE',  ( -36.28567981536816234, -9.465698090293395595, -9.422646554964174470 ) ) ;
#16600=CARTESIAN_POINT ( 'NONE',  ( -0.8051714816310078238, 0.2116216362810395268, 9.985686052694763504 ) ) ;
#16613=ORIENTED_EDGE ( 'NONE', *, *, #13057, .T. ) ;
#16634=B_SPLINE_CURVE_WITH_KNOTS ( 'NONE', 3,
 ( #13224, #8385, #36616, #44259 ),
 .UNSPECIFIED., .F., .F.,
 ( 4, 4 ),
 ( 0.000000000000000000, 0.002368422649471283847 ),
 .UNSPECIFIED. ) ;
#16639=PLANE ( 'NONE',  #13841 ) ;
#16640=CARTESIAN_POINT ( 'NONE',  ( 0.3862712429686894766, -1.188820645368940276, 10.00000000000000000 ) ) ;
#16645=CARTESIAN_POINT ( 'NONE',  ( -1.468535767197700181, -0.3224370614408916813, 9.944962737616616977 ) ) ;
#16648=CARTESIAN_POINT ( 'NONE',  ( 20.72411365307712572, -36.23316402738139885, -8.080361901872242569 ) ) ;
#16674=B_SPLINE_SURFACE_WITH_KNOTS ( 'NONE', 3, 3, ( 
 ( #487, #46111, #34618, #11006 ),
 ( #23572, #7425, #39234, #233 ),
 ( #31540, #42306, #30770, #50197 ),
 ( #38483, #18942, #4072, #46381 ) ),
 .UNSPECIFIED., .F., .F., .F.,
 ( 4, 4 ),
 ( 4, 4 ),
 ( 0.000000000000000000, 1.000000000000000000 ),
 ( 0.000000000000000000, 1.000000000000000000 ),
 .UNSPECIFIED. ) ;
#16676=CARTESIAN_POINT ( 'NONE',  ( -16.16402646813540755, 4.033894069732547827, -3.546734833711462365 ) ) ;
#16679=CARTESIAN_POINT ( 'NONE',  ( -2.188678504086925880, 0.3267089737526900350, 9.881002359080270026 ) ) ;
#16683=CARTESIAN_POINT ( 'NONE',  ( 45.21167770612395742, 22.65616271077811206, 7.906207997025717304 ) ) ;
#16684=EDGE_CURVE ( 'NONE', #37965, #1676, #132, .T. ) ;
#16687=ORIENTED_EDGE ( 'NONE', *, *, #27535, .T. ) ;
#16697=EDGE_CURVE ( 'NONE', #1440, #7897, #8025, .T. ) ;
#16711=EDGE_CURVE ( 'NONE', #12321, #36910, #43531, .T. ) ;
#16713=CARTESIAN_POINT ( 'NONE',  ( 1.347864860736642800, 0.3239901621378048491, 9.960033073700785167 ) ) ;
#16718=EDGE_CURVE ( 'NONE', #20200, #11140, #30644, .T. ) ;
#16733=VECTOR ( 'NONE', #29793, 1000.000000000000000 ) ;
#16735=DIRECTION ( 'NONE',  ( -1.000000000000000000, 0.000000000000000000, -0.000000000000000000 ) ) ;
#16742=AXIS2_PLACEMENT_3D ( 'NONE', #24648, #9733, #20533 ) ;
#16743=CARTESIAN_POINT ( 'NONE',  ( 5.990542248694086247, 8.025558178072422777, 3.215106848023467911 ) ) ;
#16750=ORIENTED_EDGE ( 'NONE', *, *, #18236, .F. ) ;
#16755=CARTESIAN_POINT ( 'NONE',  ( 3.808200756227633654, 0.8261963378076531139, 9.741991644047248045 ) ) ;
#16759=VERTEX_POINT ( 'NONE', #6085 ) ;
#16768=CARTESIAN_POINT ( 'NONE',  ( -0.6440276692615888310, -16.64212148744554298, -9.683996418299976483 ) ) ;
#16773=CARTESIAN_POINT ( 'NONE',  ( 16.52264463346132572, -2.779753662172757878, 9.403735324607438884 ) ) ;
#16787=CARTESIAN_POINT ( 'NONE',  ( 4.763548243873389154, -16.57409059453848599, 8.727788335465566760 ) ) ;
#16789=CARTESIAN_POINT ( 'NONE',  ( -16.73672383626882976, -2.341008440547994063, -9.008049429158100807 ) ) ;
#16793=EDGE_LOOP ( 'NONE', ( #9001, #40340, #29278, #30387, #41038 ) ) ;
#16796=CARTESIAN_POINT ( 'NONE',  ( 15.98719783915691650, -4.501063718205879916, 3.266473740018926541 ) ) ;
#16806=EDGE_LOOP ( 'NONE', ( #31195, #30333, #32811, #24778 ) ) ;
#16842=CARTESIAN_POINT ( 'NONE',  ( 48.98697415750968531, 11.03699497439252752, -8.016098858316199838 ) ) ;
#16852=CARTESIAN_POINT ( 'NONE',  ( -19.61585174098950546, 31.96834229807166139, -9.011255500499645521 ) ) ;
#16859=CIRCLE ( 'NONE', #23416, 10.00000000000000000 ) ;
#16860=CARTESIAN_POINT ( 'NONE',  ( 1.250000000000000222, 0.000000000000000000, -10.00000000000000000 ) ) ;
#16867=ORIENTED_EDGE ( 'NONE', *, *, #2395, .T. ) ;
#16870=EDGE_LOOP ( 'NONE', ( #39604, #46153, #22023 ) ) ;
#16875=ORIENTED_EDGE ( 'NONE', *, *, #31809, .T. ) ;
#16877=CARTESIAN_POINT ( 'NONE',  ( 13.35436367797824353, 31.26996044524050333, 7.906207997025717304 ) ) ;
#16881=ORIENTED_EDGE ( 'NONE', *, *, #18086, .F. ) ;
#16886=CARTESIAN_POINT ( 'NONE',  ( -17.51065725283106289, 28.41934970907792746, -9.367992836599954742 ) ) ;
#16903=FACE_OUTER_BOUND ( 'NONE', #29136, .T. ) ;
#16918=CARTESIAN_POINT ( 'NONE',  ( 0.3862712429686727678, 1.188820645368945605, -3.333333333333333481 ) ) ;
#16936=CARTESIAN_POINT ( 'NONE',  ( -26.20171990995768141, 42.76673505352046334, -8.466730184410787174 ) ) ;
#16950=CARTESIAN_POINT ( 'NONE',  ( 18.67411147745603373, 27.51799019669827473, -3.760136334089591248 ) ) ;
#16954=CARTESIAN_POINT ( 'NONE',  ( 1.011271242968688311, -0.7347315653655855927, 10.00000000000000000 ) ) ;
#16958=VERTEX_POINT ( 'NONE', #19408 ) ;
#16962=VERTEX_POINT ( 'NONE', #35089 ) ;
#16966=CARTESIAN_POINT ( 'NONE',  ( 33.57695195286775913, 16.69845195084893064, 8.914903342594561408 ) ) ;
#16969=CARTESIAN_POINT ( 'NONE',  ( 3.345242017215822372, -2.159124855890657724, -4.878909776184769953E-16 ) ) ;
#16976=B_SPLINE_CURVE_WITH_KNOTS ( 'NONE', 3,
 ( #4314, #44532, #20712, #40217 ),
 .UNSPECIFIED., .F., .F.,
 ( 4, 4 ),
 ( 1.093600287244414006E-15, 0.0004154657329504815111 ),
 .UNSPECIFIED. ) ;
#16977=B_SPLINE_CURVE_WITH_KNOTS ( 'NONE', 3,
 ( #7260, #37331, #18542, #17799 ),
 .UNSPECIFIED., .F., .F.,
 ( 4, 4 ),
 ( 0.0009679537044783742029, 0.001281751046851238845 ),
 .UNSPECIFIED. ) ;
#16978=CARTESIAN_POINT ( 'NONE',  ( 20.21530556545302559, -31.58467066308217497, -9.422646554964174470 ) ) ;
#16979=VERTEX_POINT ( 'NONE', #50659 ) ;
#16986=ORIENTED_EDGE ( 'NONE', *, *, #9534, .T. ) ;
#16994=CARTESIAN_POINT ( 'NONE',  ( -0.1475726264153620626, -1.496347932843211215, 9.927319414211227766 ) ) ;
#16996=CARTESIAN_POINT ( 'NONE',  ( 1.256322718835040542, 0.9753643601100148164, 9.933322880749875239 ) ) ;
#16997=CARTESIAN_POINT ( 'NONE',  ( -32.36066692128246558, 7.813306791043033606, 3.199614146704519602 ) ) ;
#17002=ORIENTED_EDGE ( 'NONE', *, *, #7054, .T. ) ;
#17023=CARTESIAN_POINT ( 'NONE',  ( -3.566525152643847285, 1.569997364305458776, 9.741991644046965604 ) ) ;
#17024=EDGE_LOOP ( 'NONE', ( #20037, #15917, #27588, #16687, #9601, #16220, #47932, #25547, #37089, #19342, #24428, #50016 ) ) ;
#17027=CARTESIAN_POINT ( 'NONE',  ( -5.325039556154594678, 2.676059031921508513, 6.606856988583542645E-16 ) ) ;
#17033=CARTESIAN_POINT ( 'NONE',  ( 0.3370904143228981575, -0.2449105217885261532, 10.00000000000000000 ) ) ;
#17034=CARTESIAN_POINT ( 'NONE',  ( 12.16428377685533135, 11.73151505502934988, -9.008049429158100807 ) ) ;
#17035=B_SPLINE_CURVE_WITH_KNOTS ( 'NONE', 3,
 ( #47973, #21067, #36753, #48965 ),
 .UNSPECIFIED., .F., .F.,
 ( 4, 4 ),
 ( 0.000000000000000000, 0.002368422649471300760 ),
 .UNSPECIFIED. ) ;
#17040=ORIENTED_EDGE ( 'NONE', *, *, #27535, .F. ) ;
#17042=CARTESIAN_POINT ( 'NONE',  ( -1.250000000000000222, 0.000000000000000000, -10.00000000000000000 ) ) ;
#17048=CARTESIAN_POINT ( 'NONE',  ( -1.019713130072858798, -3.848720492505054658, 6.098637220230962441E-17 ) ) ;
#17055=EDGE_CURVE ( 'NONE', #48113, #5629, #49573, .T. ) ;
#17063=EDGE_CURVE ( 'NONE', #2158, #7144, #7374, .T. ) ;
#17065=ORIENTED_EDGE ( 'NONE', *, *, #25589, .T. ) ;
#17067=CARTESIAN_POINT ( 'NONE',  ( -46.33529284216709243, 19.19803090445757121, -8.466730184410787174 ) ) ;
#17081=CARTESIAN_POINT ( 'NONE',  ( 21.60170755165891521, -30.69732439037074911, -6.568693074176334967 ) ) ;
#17084=CARTESIAN_POINT ( 'NONE',  ( 6.875132362119187768, -33.14667368551891258, 8.356839323120299312 ) ) ;
#17086=CARTESIAN_POINT ( 'NONE',  ( -1.655785408455817675, -0.7536129375911022610, 9.903764339332079558 ) ) ;
#17116=ORIENTED_EDGE ( 'NONE', *, *, #16161, .T. ) ;
#17124=CARTESIAN_POINT ( 'NONE',  ( 14.48769039275578407, 30.44468701195595983, 8.807470649214879543 ) ) ;
#17130=CARTESIAN_POINT ( 'NONE',  ( -9.260964247899874380, 13.84230907185616744, -9.683996418299976483 ) ) ;
#17131=CARTESIAN_POINT ( 'NONE',  ( -34.76907794179056310, 14.14424844080176236, -5.338708898921615820 ) ) ;
#17137=CARTESIAN_POINT ( 'NONE',  ( 28.55116071645549525, -41.05976639056858346, -2.408242355805840784 ) ) ;
#17140=CARTESIAN_POINT ( 'NONE',  ( 0.9985466430067150290, 1.124040728742683903, 9.944962737436837230 ) ) ;
#17144=CARTESIAN_POINT ( 'NONE',  ( -33.14391172085785797, -37.72293746533094350, -8.016098858316205167 ) ) ;
#17145=CARTESIAN_POINT ( 'NONE',  ( -15.80799809827351154, 29.65358618225718956, -8.016098858316199838 ) ) ;
#17154=B_SPLINE_CURVE_WITH_KNOTS ( 'NONE', 3,
 ( #45448, #40637, #18266, #1883 ),
 .UNSPECIFIED., .F., .F.,
 ( 4, 4 ),
 ( 0.0003760194760206989387, 0.0006307719036365364972 ),
 .UNSPECIFIED. ) ;
#17166=VECTOR ( 'NONE', #28146, 1000.000000000000114 ) ;
#17174=B_SPLINE_CURVE_WITH_KNOTS ( 'NONE', 3,
 ( #26790, #22929, #42418, #15489 ),
 .UNSPECIFIED., .F., .F.,
 ( 4, 4 ),
 ( 0.0002936521407534355859, 0.0006663369986142269122 ),
 .UNSPECIFIED. ) ;
#17175=CARTESIAN_POINT ( 'NONE',  ( -16.37555114979269888, 29.24217402453077597, -8.466730184410787174 ) ) ;
#17191=CARTESIAN_POINT ( 'NONE',  ( -12.35406723005387875, 11.51001571518090039, 9.178419661560148768 ) ) ;
#17193=CARTESIAN_POINT ( 'NONE',  ( 12.78770032058947237, 31.68259716188277864, 7.455576670931136185 ) ) ;
#17210=CARTESIAN_POINT ( 'NONE',  ( 1.468446590252912465, 0.3226319952343980058, 9.953784399990622589 ) ) ;
#17212=CARTESIAN_POINT ( 'NONE',  ( -49.46074318306826001, 9.578883844007169301, 8.807470649214879543 ) ) ;
#17252=CARTESIAN_POINT ( 'NONE',  ( 0.3862712429686810944, 1.188820645368943607, -10.00000000000000000 ) ) ;
#17262=ORIENTED_EDGE ( 'NONE', *, *, #18699, .F. ) ;
#17279=CARTESIAN_POINT ( 'NONE',  ( -15.00099850811941948, -7.462898891544107016, 9.403735324607438884 ) ) ;
#17280=B_SPLINE_CURVE_WITH_KNOTS ( 'NONE', 3,
 ( #29246, #21042, #48691, #9995 ),
 .UNSPECIFIED., .F., .F.,
 ( 4, 4 ),
 ( 0.009557256062580683775, 0.01933991692386597544 ),
 .UNSPECIFIED. ) ;
#17288=PLANE ( 'NONE',  #45856 ) ;
#17289=CARTESIAN_POINT ( 'NONE',  ( 17.43089236541784359, 28.36237856644539690, 3.199614146704519602 ) ) ;
#17290=CARTESIAN_POINT ( 'NONE',  ( -29.61572577327014955, -16.11461842845715253, 8.807470649214879543 ) ) ;
#17291=CARTESIAN_POINT ( 'NONE',  ( 0.3862712429686727678, 1.188820645368945605, 10.00000000000000000 ) ) ;
#17292=ORIENTED_EDGE ( 'NONE', *, *, #45237, .T. ) ;
#17293=VERTEX_POINT ( 'NONE', #49827 ) ;
#17294=CARTESIAN_POINT ( 'NONE',  ( -0.3656201545664206076, 2.182515578491385000, 9.881002359080270026 ) ) ;
#17302=CARTESIAN_POINT ( 'NONE',  ( -20.08067494016849608, -41.72051557472617134, 7.455576670931136185 ) ) ;
#17304=ORIENTED_EDGE ( 'NONE', *, *, #40896, .F. ) ;
#17307=VECTOR ( 'NONE', #27585, 1000.000000000000114 ) ;
#17315=ORIENTED_EDGE ( 'NONE', *, *, #19752, .T. ) ;
#17331=CARTESIAN_POINT ( 'NONE',  ( -8.843309649387274263, 14.11631751497152720, -2.870787844569587133 ) ) ;
#17343=CARTESIAN_POINT ( 'NONE',  ( -0.3862712429686895876, 1.188820645368940720, -3.333333333333333481 ) ) ;
#17352=FACE_OUTER_BOUND ( 'NONE', #40126, .T. ) ;
#17359=VERTEX_POINT ( 'NONE', #31681 ) ;
#17372=ORIENTED_EDGE ( 'NONE', *, *, #41861, .T. ) ;
#17384=CARTESIAN_POINT ( 'NONE',  ( 7.398363427652525637, -15.19415887381133246, -9.008049429158100807 ) ) ;
#17391=CARTESIAN_POINT ( 'NONE',  ( 48.99656738986517723, -11.00747004110342431, 1.847720168420772691 ) ) ;
#17405=EDGE_CURVE ( 'NONE', #17745, #5629, #31417, .T. ) ;
#17407=CARTESIAN_POINT ( 'NONE',  ( 34.08355720199905647, -2.371364769369109116, 7.455576670931136185 ) ) ;
#17419=CARTESIAN_POINT ( 'NONE',  ( -5.888214538810513154, -16.20866436362413410, 8.727788335465566760 ) ) ;
#17442=CARTESIAN_POINT ( 'NONE',  ( -1.150625731496824011, 0.4126014017553036872, 9.969517326150318937 ) ) ;
#17443=CARTESIAN_POINT ( 'NONE',  ( -2.569099690548740877, 33.19126772784019153, 3.199614146704519602 ) ) ;
#17447=ORIENTED_EDGE ( 'NONE', *, *, #47446, .T. ) ;
#17467=CARTESIAN_POINT ( 'NONE',  ( 11.73320209285708415, -11.96063479729170886, 9.403735324607438884 ) ) ;
#17468=ORIENTED_EDGE ( 'NONE', *, *, #22040, .F. ) ;
#17482=CARTESIAN_POINT ( 'NONE',  ( -1.540526284687967706, 1.371707213411501147, 9.886433018048069954 ) ) ;
#17483=CARTESIAN_POINT ( 'NONE',  ( 32.43949840348898306, 7.871562655726499713, -9.367992836599954742 ) ) ;
#17493=CARTESIAN_POINT ( 'NONE',  ( 44.99506233596246574, 23.32283626942318477, 7.455576670931136185 ) ) ;
#17499=CARTESIAN_POINT ( 'NONE',  ( -7.216980890441389462, 6.922079660550276792, 0.000000000000000000 ) ) ;
#17500=CARTESIAN_POINT ( 'NONE',  ( -15.45175104485246820, 6.222373774239106758, -2.870787844569587133 ) ) ;
#17502=ORIENTED_EDGE ( 'NONE', *, *, #12886, .F. ) ;
#17511=ORIENTED_EDGE ( 'NONE', *, *, #41392, .F. ) ;
#17524=B_SPLINE_SURFACE_WITH_KNOTS ( 'NONE', 3, 3, ( 
 ( #41500, #17145, #1504, #28944 ),
 ( #33561, #21745, #37178, #21240 ),
 ( #10203, #32560, #33314, #29444 ),
 ( #29204, #44555, #5339, #44820 ) ),
 .UNSPECIFIED., .F., .F., .F.,
 ( 4, 4 ),
 ( 4, 4 ),
 ( 0.000000000000000000, 1.000000000000000000 ),
 ( 0.000000000000000000, 1.000000000000000000 ),
 .UNSPECIFIED. ) ;
#17529=CARTESIAN_POINT ( 'NONE',  ( 33.64889274059390090, -3.704246042440748621, 8.356839323120299312 ) ) ;
#17531=CARTESIAN_POINT ( 'NONE',  ( -23.31729631074215092, -24.19776167542410406, -8.016098858316199838 ) ) ;
#17535=B_SPLINE_CURVE_WITH_KNOTS ( 'NONE', 3,
 ( #40188, #5024, #20684, #1201 ),
 .UNSPECIFIED., .F., .F.,
 ( 4, 4 ),
 ( 0.0009679537044783566389, 0.001281751046851271805 ),
 .UNSPECIFIED. ) ;
#17536=CARTESIAN_POINT ( 'NONE',  ( 0.3370904143228924954, 0.2449105217885333141, -10.00000000000000000 ) ) ;
#17540=CARTESIAN_POINT ( 'NONE',  ( 12.78770032058947237, 31.68259716188277864, 7.455576670931136185 ) ) ;
#17541=VECTOR ( 'NONE', #36184, 1000.000000000000000 ) ;
#17549=CARTESIAN_POINT ( 'NONE',  ( 1.249999999999999778, -0.000000000000000000, -10.00000000000000000 ) ) ;
#17573=PLANE ( 'NONE',  #36543 ) ;
#17575=CARTESIAN_POINT ( 'NONE',  ( 47.55282581475750447, 15.45084971874791080, 0.000000000000000000 ) ) ;
#17582=CARTESIAN_POINT ( 'NONE',  ( 48.99656738986517723, -11.00747004110342431, 1.847720168420772691 ) ) ;
#17583=LINE ( 'NONE', #33257, #24491 ) ;
#17598=CARTESIAN_POINT ( 'NONE',  ( 1.377636575563020438, -0.6021164824561170414, 9.953784399990622589 ) ) ;
#17603=CARTESIAN_POINT ( 'NONE',  ( 0.3862712429686810944, 1.188820645368943607, 10.00000000000000000 ) ) ;
#17604=CARTESIAN_POINT ( 'NONE',  ( -4.030066147382709296, 6.879218662320311317, 9.147955830346443662E-16 ) ) ;
#17605=B_SPLINE_CURVE_WITH_KNOTS ( 'NONE', 3,
 ( #30617, #26764, #6750, #2644 ),
 .UNSPECIFIED., .F., .F.,
 ( 4, 4 ),
 ( 0.002911903035958271057, 0.009050416366962861503 ),
 .UNSPECIFIED. ) ;
#17613=CARTESIAN_POINT ( 'NONE',  ( -0.5349938414998356428, -3.214699992961246977, 9.799352050262458036 ) ) ;
#17637=FACE_OUTER_BOUND ( 'NONE', #33736, .T. ) ;
#17642=CARTESIAN_POINT ( 'NONE',  ( -23.29043492822808759, 24.10797434788186067, 1.847720168420772691 ) ) ;
#17644=DIRECTION ( 'NONE',  ( 0.000000000000000000, 0.000000000000000000, -1.000000000000000000 ) ) ;
#17648=FACE_OUTER_BOUND ( 'NONE', #36293, .T. ) ;
#17656=CARTESIAN_POINT ( 'NONE',  ( 1.270883027773819229, 0.2878889193223041487, 9.961922210043287151 ) ) ;
#17682=VERTEX_POINT ( 'NONE', #14928 ) ;
#17699=CARTESIAN_POINT ( 'NONE',  ( -0.8433491450857070193, 0.9182416014173486740, 9.981352469109932457 ) ) ;
#17700=CARTESIAN_POINT ( 'NONE',  ( -32.43949840348904701, -7.871562655726274116, -9.367992836599954742 ) ) ;
#17705=CARTESIAN_POINT ( 'NONE',  ( 21.58778298521313843, -25.34222074689757065, 3.199614146704519602 ) ) ;
#17709=CARTESIAN_POINT ( 'NONE',  ( -15.00099850811941948, -7.462898891544107016, 9.403735324607438884 ) ) ;
#17716=ADVANCED_FACE ( 'NONE', ( #49013 ), #50167, .T. ) ;
#17733=EDGE_CURVE ( 'NONE', #25169, #16336, #23, .T. ) ;
#17741=CARTESIAN_POINT ( 'NONE',  ( 48.33712804702526000, 13.03701565032775456, -9.367992836599954742 ) ) ;
#17745=VERTEX_POINT ( 'NONE', #19786 ) ;
#17751=CARTESIAN_POINT ( 'NONE',  ( -0.9983599181300891745, -1.124146016603549070, 9.953784399990620813 ) ) ;
#17752=EDGE_CURVE ( 'NONE', #50186, #31279, #5452, .T. ) ;
#17755=CARTESIAN_POINT ( 'NONE',  ( 1.193089574352119264, 0.2545860991493882342, 9.963925895596188909 ) ) ;
#17756=CARTESIAN_POINT ( 'NONE',  ( -30.21887974406478250, 14.69854701517550666, -8.016098858316199838 ) ) ;
#17758=CARTESIAN_POINT ( 'NONE',  ( -1.211050186583223720, -0.5544523570010669866, 9.951893257060014264 ) ) ;
#17762=CARTESIAN_POINT ( 'NONE',  ( -1.320835335343009787, 0.01943189458965158267, 9.943883492372876276 ) ) ;
#17766=VERTEX_POINT ( 'NONE', #20044 ) ;
#17785=CARTESIAN_POINT ( 'NONE',  ( -17.43089236541806031, -28.36237856644526900, 3.199614146704519602 ) ) ;
#17788=CARTESIAN_POINT ( 'NONE',  ( 1.011271242968688311, -0.7347315653655855927, 10.00000000000000000 ) ) ;
#17791=CARTESIAN_POINT ( 'NONE',  ( 25.63461350838963071, -43.17876197216377676, -8.016098858316205167 ) ) ;
#17792=B_SPLINE_CURVE_WITH_KNOTS ( 'NONE', 3,
 ( #29892, #25286, #37866, #45005 ),
 .UNSPECIFIED., .F., .F.,
 ( 4, 4 ),
 ( 9.129125108812345642E-16, 0.0004154657329515903247 ),
 .UNSPECIFIED. ) ;
#17796=CARTESIAN_POINT ( 'NONE',  ( 10.00000000000000000, 1.224646799147353256E-15, 10.00000000000000000 ) ) ;
#17799=CARTESIAN_POINT ( 'NONE',  ( -0.8282505383454070724, -1.889063466747028297, 9.894754715216727448 ) ) ;
#17800=CARTESIAN_POINT ( 'NONE',  ( 0.000000000000000000, 0.000000000000000000, 0.000000000000000000 ) ) ;
#17804=CARTESIAN_POINT ( 'NONE',  ( -0.2778388845795317086, 1.251314014313103851, 9.976582533991678048 ) ) ;
#17806=CARTESIAN_POINT ( 'NONE',  ( -0.6215990105957072132, 1.608617984725374983, 9.928159647716134018 ) ) ;
#17812=VERTEX_POINT ( 'NONE', #47202 ) ;
#17818=CARTESIAN_POINT ( 'NONE',  ( -30.43621780902774532, 14.03210827430580210, -8.466730184410787174 ) ) ;
#17830=EDGE_CURVE ( 'NONE', #43927, #11996, #50108, .T. ) ;
#17831=CARTESIAN_POINT ( 'NONE',  ( -8.277096487746778308, 50.00000000000000000, 7.455576670931136185 ) ) ;
#17838=CARTESIAN_POINT ( 'NONE',  ( 6.174150299305392053, -33.14591993373988998, 8.807470649214879543 ) ) ;
#17839=DIRECTION ( 'NONE',  ( -0.000000000000000000, -0.000000000000000000, -1.000000000000000000 ) ) ;
#17853=CARTESIAN_POINT ( 'NONE',  ( -34.95136153415531766, 36.40974830873496870, 8.356839323120299312 ) ) ;
#17862=CARTESIAN_POINT ( 'NONE',  ( 12.78770032058947237, 31.68259716188277864, 7.455576670931136185 ) ) ;
#17874=CARTESIAN_POINT ( 'NONE',  ( -0.8155877869437639927, -0.9072449372115535260, 9.963925895596188909 ) ) ;
#17876=CARTESIAN_POINT ( 'NONE',  ( 2.538055338523173443, 50.00000000000000000, -9.367992836599951190 ) ) ;
#17879=CARTESIAN_POINT ( 'NONE',  ( 0.9460392030551082465, 0.7922402054952416561, 9.969907203203607793 ) ) ;
#17886=CARTESIAN_POINT ( 'NONE',  ( -14.76429217231967428, -8.192625680377590314, 9.178419661560148768 ) ) ;
#17887=CARTESIAN_POINT ( 'NONE',  ( 0.2774838294623813151, -1.251476322270253405, 9.957892297621013356 ) ) ;
#17888=B_SPLINE_CURVE_WITH_KNOTS ( 'NONE', 3,
 ( #25470, #48265, #29566, #21109 ),
 .UNSPECIFIED., .F., .F.,
 ( 4, 4 ),
 ( 0.0004299334430849316652, 0.0007706806524479852200 ),
 .UNSPECIFIED. ) ;
#17906=VERTEX_POINT ( 'NONE', #806 ) ;
#17924=B_SPLINE_SURFACE_WITH_KNOTS ( 'NONE', 3, 3, ( 
 ( #49207, #6154, #21545, #36983 ),
 ( #1805, #33121, #2056, #25662 ),
 ( #21806, #44868, #9740, #25405 ),
 ( #41053, #17700, #33370, #37479 ) ),
 .UNSPECIFIED., .F., .F., .F.,
 ( 4, 4 ),
 ( 4, 4 ),
 ( 0.000000000000000000, 1.000000000000000000 ),
 ( 0.000000000000000000, 1.000000000000000000 ),
 .UNSPECIFIED. ) ;
#17938=CARTESIAN_POINT ( 'NONE',  ( -29.39982726364978660, -16.78152490921149109, 8.356839323120299312 ) ) ;
#17939=CARTESIAN_POINT ( 'NONE',  ( -16.52264463346130796, 2.779753662172870232, 9.403735324607438884 ) ) ;
#17946=CARTESIAN_POINT ( 'NONE',  ( 13.35436367797824353, 31.26996044524050333, 7.906207997025717304 ) ) ;
#17947=CARTESIAN_POINT ( 'NONE',  ( -0.3862712429686809279, -1.188820645368943163, 10.00000000000000000 ) ) ;
#17948=CARTESIAN_POINT ( 'NONE',  ( -6.174150299305392053, 33.14591993373988998, 8.807470649214879543 ) ) ;
#17956=CARTESIAN_POINT ( 'NONE',  ( -8.277096487746778308, 50.00000000000000711, 7.455576670931136185 ) ) ;
#17965=CARTESIAN_POINT ( 'NONE',  ( -19.81499429539154278, 31.87968861126203635, -5.338708898921614043 ) ) ;
#17966=ORIENTED_EDGE ( 'NONE', *, *, #48331, .F. ) ;
#17970=CARTESIAN_POINT ( 'NONE',  ( 44.99506233596247995, 23.32283626942318833, 7.455576670931136185 ) ) ;
#17974=CARTESIAN_POINT ( 'NONE',  ( -0.1425549192113998442, 1.238581250503548059, 9.981352469109934233 ) ) ;
#17975=EDGE_CURVE ( 'NONE', #29885, #44630, #26901, .T. ) ;
#17986=EDGE_CURVE ( 'NONE', #1823, #9976, #15282, .T. ) ;
#17992=CARTESIAN_POINT ( 'NONE',  ( -7.398363427652414614, 15.19415887381139108, -9.008049429158100807 ) ) ;
#17999=CARTESIAN_POINT ( 'NONE',  ( 9.760995290733820440, -2.173239732351728293, 9.646707543097347681 ) ) ;
#18001=EDGE_CURVE ( 'NONE', #10758, #6007, #21994, .T. ) ;
#18004=CARTESIAN_POINT ( 'NONE',  ( -1.249999999999999778, 0.000000000000000000, 10.00000000000000000 ) ) ;
#18006=CARTESIAN_POINT ( 'NONE',  ( -13.35436367797847801, -31.26996044524040741, 7.906207997025717304 ) ) ;
#18009=CARTESIAN_POINT ( 'NONE',  ( -1.164014690938856456, 0.7287989552215266009, 9.946805383069621698 ) ) ;
#18027=DIRECTION ( 'NONE',  ( -0.3090169943749515591, 0.9510565162951523099, 0.000000000000000000 ) ) ;
#18032=B_SPLINE_CURVE_WITH_KNOTS ( 'NONE', 3,
 ( #48746, #13636, #25447, #21585, #10542, #19244 ),
 .UNSPECIFIED., .F., .F.,
 ( 4, 2, 4 ),
 ( 9.965227682168975268E-18, 0.009877169331704831884, 0.01975433866340965683 ),
 .UNSPECIFIED. ) ;
#18033=CARTESIAN_POINT ( 'NONE',  ( 6.508636631827673824, 15.75743548351451295, 8.953103998512858652 ) ) ;
#18037=CARTESIAN_POINT ( 'NONE',  ( 0.3862712429686894211, -1.188820645368940276, 9.972675548442463622 ) ) ;
#18042=ADVANCED_FACE ( 'NONE', ( #41056 ), #19504, .T. ) ;
#18043=B_SPLINE_CURVE_WITH_KNOTS ( 'NONE', 3,
 ( #6507, #22917, #26774, #2890 ),
 .UNSPECIFIED., .F., .F.,
 ( 4, 4 ),
 ( 0.0004299334430849581197, 0.0007706806524480063619 ),
 .UNSPECIFIED. ) ;
#18046=ORIENTED_EDGE ( 'NONE', *, *, #16175, .F. ) ;
#18078=CARTESIAN_POINT ( 'NONE',  ( 36.08557433729230013, -35.58569447144767395, 7.455576670931136185 ) ) ;
#18086=EDGE_CURVE ( 'NONE', #42215, #35501, #33545, .T. ) ;
#18098=VERTEX_POINT ( 'NONE', #7171 ) ;
#18116=CARTESIAN_POINT ( 'NONE',  ( 10.30302290646030627, 13.08520913973580058, -9.683996418299976483 ) ) ;
#18124=DIRECTION ( 'NONE',  ( 0.2599384441937558354, 0.8000082703740967194, -0.5407575913134976542 ) ) ;
#18132=ORIENTED_EDGE ( 'NONE', *, *, #23160, .T. ) ;
#18134=CARTESIAN_POINT ( 'NONE',  ( 30.22736451279166658, 39.84193304692632154, -2.408242355805840784 ) ) ;
#18138=CARTESIAN_POINT ( 'NONE',  ( 17.23491422248386584, -0.5912720620000816441, 8.727788335465566760 ) ) ;
#18139=B_SPLINE_CURVE_WITH_KNOTS ( 'NONE', 3,
 ( #39470, #24818, #40470, #16106 ),
 .UNSPECIFIED., .F., .F.,
 ( 4, 4 ),
 ( 0.0003309173790299507799, 0.0006447147193715880220 ),
 .UNSPECIFIED. ) ;
#18150=EDGE_LOOP ( 'NONE', ( #33835, #32380, #22089 ) ) ;
#18164=CARTESIAN_POINT ( 'NONE',  ( -16.16402646813540755, 4.033894069732547827, -3.546734833711462365 ) ) ;
#18169=CARTESIAN_POINT ( 'NONE',  ( 34.38425513258721367, -36.82177522737821107, 8.807470649214879543 ) ) ;
#18182=CARTESIAN_POINT ( 'NONE',  ( -1.011271242968693862, 0.7347315653655780432, -3.333333333333333481 ) ) ;
#18185=CARTESIAN_POINT ( 'NONE',  ( -6.174150299305392053, 50.00000000000000711, 8.807470649214879543 ) ) ;
#18191=CARTESIAN_POINT ( 'NONE',  ( 1.011271242968688311, -0.7347315653655855927, 10.00000000000000000 ) ) ;
#18192=EDGE_LOOP ( 'NONE', ( #48822, #35842, #7582 ) ) ;
#18194=CARTESIAN_POINT ( 'NONE',  ( 24.47767542868285062, -23.18653802921781448, 8.807470649214879543 ) ) ;
#18196=CARTESIAN_POINT ( 'NONE',  ( -1.011271242968683426, -0.7347315653655928092, 3.333333333333333481 ) ) ;
#18198=VERTEX_POINT ( 'NONE', #9881 ) ;
#18200=CARTESIAN_POINT ( 'NONE',  ( 7.129058724844953510, 15.30620660340485095, 9.178419661560148768 ) ) ;
#18202=CARTESIAN_POINT ( 'NONE',  ( 0.8283411193307036458, 1.889045124114310026, 9.891980816043068003 ) ) ;
#18204=EDGE_CURVE ( 'NONE', #13812, #8942, #27454, .T. ) ;
#18209=CARTESIAN_POINT ( 'NONE',  ( 0.4166666666666669072, 0.000000000000000000, 10.00000000000000000 ) ) ;
#18218=VERTEX_POINT ( 'NONE', #13731 ) ;
#18219=CARTESIAN_POINT ( 'NONE',  ( -45.64490844644706158, -21.32281559348763977, 8.807470649214879543 ) ) ;
#18222=CARTESIAN_POINT ( 'NONE',  ( -12.35406723005387875, 11.51001571518090039, 9.178419661560148768 ) ) ;
#18228=CARTESIAN_POINT ( 'NONE',  ( -16.52264463346130796, 2.779753662172870232, 9.403735324607438884 ) ) ;
#18230=ORIENTED_EDGE ( 'NONE', *, *, #42205, .F. ) ;
#18236=EDGE_CURVE ( 'NONE', #9153, #23786, #46406, .T. ) ;
#18238=B_SPLINE_SURFACE_WITH_KNOTS ( 'NONE', 3, 3, ( 
 ( #42361, #46435, #38790, #19776 ),
 ( #22615, #42609, #7224, #23379 ),
 ( #34953, #39049, #26970, #298 ),
 ( #31347, #35457, #15427, #39292 ) ),
 .UNSPECIFIED., .F., .F., .F.,
 ( 4, 4 ),
 ( 4, 4 ),
 ( 0.000000000000000000, 1.000000000000000000 ),
 ( 0.000000000000000000, 1.000000000000000000 ),
 .UNSPECIFIED. ) ;
#18240=DIRECTION ( 'NONE',  ( -1.000000000000000000, 0.000000000000000000, 0.000000000000000000 ) ) ;
#18242=CARTESIAN_POINT ( 'NONE',  ( -24.47767542868268364, 23.18653802921800278, 8.807470649214879543 ) ) ;
#18244=EDGE_LOOP ( 'NONE', ( #20347, #521, #48370, #857 ) ) ;
#18245=ORIENTED_EDGE ( 'NONE', *, *, #22024, .T. ) ;
#18251=SHAPE_REPRESENTATION_RELATIONSHIP ( 'NONE' , 'NONE' ,  #39915, #21546 ) ;
#18266=CARTESIAN_POINT ( 'NONE',  ( -0.7248414106044189786, 1.181973560820994917, 9.960027343378008879 ) ) ;
#18280=EDGE_LOOP ( 'NONE', ( #23476, #24501, #24783 ) ) ;
#18288=CARTESIAN_POINT ( 'NONE',  ( 1.019713130072856355, 3.848720492505100843, 4.370690007832189750E-16 ) ) ;
#18294=EDGE_CURVE ( 'NONE', #37965, #27105, #44260, .T. ) ;
#18296=ORIENTED_EDGE ( 'NONE', *, *, #29276, .F. ) ;
#18305=FACE_OUTER_BOUND ( 'NONE', #14653, .T. ) ;
#18314=CARTESIAN_POINT ( 'NONE',  ( 9.998889670239195837, 0.1490146381531976816, 9.282506307616472441 ) ) ;
#18319=CARTESIAN_POINT ( 'NONE',  ( -2.052581215100349521, 0.2042358160481012597, 9.886433018048073507 ) ) ;
#18321=CARTESIAN_POINT ( 'NONE',  ( 0.3862712429686810944, 1.188820645368943607, 10.00000000000000000 ) ) ;
#18336=CARTESIAN_POINT ( 'NONE',  ( -16.73672383626882976, -2.341008440547994063, -9.008049429158100807 ) ) ;
#18337=CARTESIAN_POINT ( 'NONE',  ( -5.888214538810513154, -16.20866436362413410, 8.727788335465566760 ) ) ;
#18338=CARTESIAN_POINT ( 'NONE',  ( 1.011271242968677653, 0.7347315653656002477, -10.00000000000000000 ) ) ;
#18349=ORIENTED_EDGE ( 'NONE', *, *, #37885, .T. ) ;
#18355=VERTEX_POINT ( 'NONE', #42186 ) ;
#18360=CARTESIAN_POINT ( 'NONE',  ( 15.73090589902275482, 29.60029367929053024, 1.847720168420772691 ) ) ;
#18373=CARTESIAN_POINT ( 'NONE',  ( 0.3910393408562611861, 3.877122853646846945, 9.741991644046958498 ) ) ;
#18381=CARTESIAN_POINT ( 'NONE',  ( 2.569099690548740877, -33.19126772784019153, 3.199614146704519602 ) ) ;
#18387=CARTESIAN_POINT ( 'NONE',  ( -17.51065725283106289, 28.41934970907792746, -9.367992836599954742 ) ) ;
#18388=ADVANCED_FACE ( 'NONE', ( #14227 ), #38364, .T. ) ;
#18393=ORIENTED_EDGE ( 'NONE', *, *, #3975, .T. ) ;
#18398=EDGE_CURVE ( 'NONE', #36524, #21893, #6627, .T. ) ;
#18402=CARTESIAN_POINT ( 'NONE',  ( -4.339432828817248122, -37.24807810779213213, -8.192531242611266862 ) ) ;
#18405=CARTESIAN_POINT ( 'NONE',  ( -0.6215990105957072132, 1.608617984725374983, 9.928159647716134018 ) ) ;
#18407=CARTESIAN_POINT ( 'NONE',  ( 7.203307948779654524, -6.979912421814508328, 9.516222621873129839 ) ) ;
#18427=CARTESIAN_POINT ( 'NONE',  ( 1.365263087672787590, -0.5437404457008400138, 9.958264684458717042 ) ) ;
#18433=CARTESIAN_POINT ( 'NONE',  ( -1.231028901681122445, -0.08486789822041165832, 9.969907203203806745 ) ) ;
#18434=CARTESIAN_POINT ( 'NONE',  ( 33.47329838550567160, -31.99020508012700148, 7.455576670931137073 ) ) ;
#18447=CARTESIAN_POINT ( 'NONE',  ( -42.07173315646050327, 18.54977254542426124, -8.016098858316205167 ) ) ;
#18458=CARTESIAN_POINT ( 'NONE',  ( -33.14391172085785797, -37.72293746533095060, -8.016098858316199838 ) ) ;
#18460=CARTESIAN_POINT ( 'NONE',  ( 0.3862712429686727678, 1.188820645368945605, 3.333333333333333481 ) ) ;
#18461=CARTESIAN_POINT ( 'NONE',  ( -3.229232847726260403, 16.57333684275945629, 9.178419661560148768 ) ) ;
#18487=CARTESIAN_POINT ( 'NONE',  ( 4.339432828817248122, 37.24807810779213213, -8.192531242611266862 ) ) ;
#18490=VECTOR ( 'NONE', #5276, 1000.000000000000000 ) ;
#18495=CARTESIAN_POINT ( 'NONE',  ( 0.3139796262078408673, -1.230474926876621078, 9.975314328424616406 ) ) ;
#18500=CARTESIAN_POINT ( 'NONE',  ( -1.448406091252275818, 0.9360325558308429938, 9.928159647716187308 ) ) ;
#18501=CARTESIAN_POINT ( 'NONE',  ( -0.3370904143228927730, -0.2449105217885335917, 10.00000000000000000 ) ) ;
#18508=CARTESIAN_POINT ( 'NONE',  ( -34.38425513258695077, 36.82177522737848108, 8.807470649214879543 ) ) ;
#18528=ADVANCED_FACE ( 'NONE', ( #32180 ), #30566, .T. ) ;
#18534=CARTESIAN_POINT ( 'NONE',  ( -1.153670525509249423, -0.4304314044324315525, 9.975326647350897247 ) ) ;
#18535=VERTEX_POINT ( 'NONE', #5468 ) ;
#18538=CARTESIAN_POINT ( 'NONE',  ( -1.468713901642213493, -0.3220470327672489419, 9.927319414211227766 ) ) ;
#18542=CARTESIAN_POINT ( 'NONE',  ( -0.8510287611193614321, -1.787020300838985110, 9.897807938190497978 ) ) ;
#18543=B_SPLINE_CURVE_WITH_KNOTS ( 'NONE', 3,
 ( #5309, #25073, #20968, #36653 ),
 .UNSPECIFIED., .F., .F.,
 ( 4, 4 ),
 ( 0.000000000000000000, 0.0002610106747150240823 ),
 .UNSPECIFIED. ) ;
#18553=CARTESIAN_POINT ( 'NONE',  ( -1.011271242968688533, 0.7347315653655859258, 10.00000000000000000 ) ) ;
#18557=CARTESIAN_POINT ( 'NONE',  ( 1.158497635116737312, -16.61944452314319420, -3.546734833711462365 ) ) ;
#18569=CARTESIAN_POINT ( 'NONE',  ( -34.95136153415531766, 36.40974830873496870, 8.356839323120299312 ) ) ;
#18571=CARTESIAN_POINT ( 'NONE',  ( 23.26005729352310425, 44.90397804740356236, 7.906207997025717304 ) ) ;
#18576=DIRECTION ( 'NONE',  ( 0.000000000000000000, 0.000000000000000000, -1.000000000000000000 ) ) ;
#18581=CARTESIAN_POINT ( 'NONE',  ( 0.1287570809895604018, 0.3962735484563146282, 10.00000000000000000 ) ) ;
#18585=CARTESIAN_POINT ( 'NONE',  ( 0.6126904405382156416, 1.085824959725723016, 9.981352469109932457 ) ) ;
#18590=CARTESIAN_POINT ( 'NONE',  ( 13.59579750444771307, -10.60877755095900632, 8.727788335465566760 ) ) ;
#18593=EDGE_CURVE ( 'NONE', #13052, #48164, #18885, .T. ) ;
#18595=ORIENTED_EDGE ( 'NONE', *, *, #20982, .F. ) ;
#18597=CARTESIAN_POINT ( 'NONE',  ( -2.961022939495062900, 16.59676755884084187, 2.590526750877053086 ) ) ;
#18604=ORIENTED_EDGE ( 'NONE', *, *, #12924, .T. ) ;
#18618=ORIENTED_EDGE ( 'NONE', *, *, #50617, .F. ) ;
#18619=ORIENTED_EDGE ( 'NONE', *, *, #10266, .T. ) ;
#18643=CARTESIAN_POINT ( 'NONE',  ( 12.15085308559846844, -11.68662139125803989, 2.590526750877053086 ) ) ;
#18644=CARTESIAN_POINT ( 'NONE',  ( -37.27397286063865778, 4.111076158911805223, 7.697694107796192675 ) ) ;
#18654=CARTESIAN_POINT ( 'NONE',  ( -0.3862712429686809279, -1.188820645368942941, 9.972675548442463622 ) ) ;
#18666=EDGE_CURVE ( 'NONE', #25205, #28949, #45764, .T. ) ;
#18683=ORIENTED_EDGE ( 'NONE', *, *, #4497, .T. ) ;
#18687=CARTESIAN_POINT ( 'NONE',  ( -1.011271242968693862, 0.7347315653655780432, 3.333333333333333481 ) ) ;
#18692=DIRECTION ( 'NONE',  ( -1.000000000000000000, 0.000000000000000000, 0.000000000000000000 ) ) ;
#18693=FACE_OUTER_BOUND ( 'NONE', #12754, .T. ) ;
#18694=CARTESIAN_POINT ( 'NONE',  ( 1.011271242968688311, -0.7347315653655855927, 10.00000000000000000 ) ) ;
#18695=FACE_OUTER_BOUND ( 'NONE', #25645, .T. ) ;
#18699=EDGE_CURVE ( 'NONE', #17766, #46997, #16354, .T. ) ;
#18704=CARTESIAN_POINT ( 'NONE',  ( 1.769963848780946369, -9.842115015280432644, 0.000000000000000000 ) ) ;
#18705=CARTESIAN_POINT ( 'NONE',  ( 0.4166666666666669072, 0.000000000000000000, 10.00000000000000000 ) ) ;
#18706=ORIENTED_EDGE ( 'NONE', *, *, #31217, .F. ) ;
#18724=B_SPLINE_CURVE_WITH_KNOTS ( 'NONE', 3,
 ( #20721, #33040, #47879, #44057 ),
 .UNSPECIFIED., .F., .F.,
 ( 4, 4 ),
 ( 0.9688112071879397824, 0.9724175925769218409 ),
 .UNSPECIFIED. ) ;
#18734=CARTESIAN_POINT ( 'NONE',  ( -9.386495789655715072, -3.489743738556220443, 6.429802539306306741 ) ) ;
#18736=CARTESIAN_POINT ( 'NONE',  ( 0.3862712429686894211, -1.188820645368940276, 9.972675548442463622 ) ) ;
#18737=EDGE_CURVE ( 'NONE', #49396, #19482, #15717, .T. ) ;
#18740=FACE_BOUND ( 'NONE', #25421, .T. ) ;
#18752=CARTESIAN_POINT ( 'NONE',  ( -26.18032376592659105, 21.95228666728381128, 7.455576670931136185 ) ) ;
#18754=CARTESIAN_POINT ( 'NONE',  ( 1.011271242968677653, 0.7347315653656002477, -10.00000000000000000 ) ) ;
#18757=EDGE_LOOP ( 'NONE', ( #43717, #33894, #24806 ) ) ;
#18768=CARTESIAN_POINT ( 'NONE',  ( 30.21887974406487487, -14.69854701517530060, -8.016098858316199838 ) ) ;
#18769=B_SPLINE_SURFACE_WITH_KNOTS ( 'NONE', 3, 3, ( 
 ( #23016, #34585, #3259, #30739 ),
 ( #46346, #30999, #11240, #42513 ),
 ( #34090, #49916, #3011, #7391 ),
 ( #2758, #11486, #7133, #14820 ) ),
 .UNSPECIFIED., .F., .F., .F.,
 ( 4, 4 ),
 ( 4, 4 ),
 ( 0.000000000000000000, 1.000000000000000000 ),
 ( 0.000000000000000000, 1.000000000000000000 ),
 .UNSPECIFIED. ) ;
#18770=CARTESIAN_POINT ( 'NONE',  ( -48.99656738986512039, 11.00747004110376182, 1.847720168420772691 ) ) ;
#18781=VECTOR ( 'NONE', #10578, 1000.000000000000114 ) ;
#18784=CARTESIAN_POINT ( 'NONE',  ( -0.3862712429686977478, 1.188820645368937390, -10.00000000000000000 ) ) ;
#18787=CARTESIAN_POINT ( 'NONE',  ( -10.00000000000000000, 0.000000000000000000, 10.00000000000000000 ) ) ;
#18791=CARTESIAN_POINT ( 'NONE',  ( 0.04754753503591857555, -0.8311582663284580175, 9.985686052694763504 ) ) ;
#18801=CARTESIAN_POINT ( 'NONE',  ( -14.29087950072019098, -9.652079258044555132, 8.727788335465566760 ) ) ;
#18808=EDGE_CURVE ( 'NONE', #20022, #42350, #12094, .T. ) ;
#18819=CARTESIAN_POINT ( 'NONE',  ( -13.59579750444763668, 10.60877755095910935, 8.727788335465566760 ) ) ;
#18821=CARTESIAN_POINT ( 'NONE',  ( -0.3862712429686809279, -1.188820645368943163, 3.333333333333333481 ) ) ;
#18838=CARTESIAN_POINT ( 'NONE',  ( 23.29043492822826167, -24.10797434788167948, 1.847720168420772691 ) ) ;
#18845=CARTESIAN_POINT ( 'NONE',  ( 2.538055338523177440, 50.00000000000000711, -9.367992836599954742 ) ) ;
#18851=FACE_OUTER_BOUND ( 'NONE', #18150, .T. ) ;
#18856=VECTOR ( 'NONE', #45858, 1000.000000000000227 ) ;
#18860=CARTESIAN_POINT ( 'NONE',  ( 1.370084944437007568, 0.09457992852872378065, 9.946805383069623474 ) ) ;
#18864=CARTESIAN_POINT ( 'NONE',  ( -3.808200756227646089, -0.8261963378076270237, 9.741991644047246268 ) ) ;
#18868=EDGE_CURVE ( 'NONE', #715, #48113, #32271, .T. ) ;
#18870=B_SPLINE_CURVE_WITH_KNOTS ( 'NONE', 3,
 ( #24440, #48230, #47981, #13120 ),
 .UNSPECIFIED., .F., .F.,
 ( 4, 4 ),
 ( 5.641302087653063738E-05, 0.0003272669002613203459 ),
 .UNSPECIFIED. ) ;
#18874=CARTESIAN_POINT ( 'NONE',  ( 30.12518629743562926, 14.70074613238908157, 1.847720168420772691 ) ) ;
#18885=B_SPLINE_CURVE_WITH_KNOTS ( 'NONE', 3,
 ( #44446, #33447, #33198, #8828 ),
 .UNSPECIFIED., .F., .F.,
 ( 4, 4 ),
 ( 0.000000000000000000, 2.647279941188469089E-05 ),
 .UNSPECIFIED. ) ;
#18886=CARTESIAN_POINT ( 'NONE',  ( -4.353119224255007857, -9.002796955359011477, 0.000000000000000000 ) ) ;
#18887=EDGE_CURVE ( 'NONE', #1058, #42210, #29802, .T. ) ;
#18889=CARTESIAN_POINT ( 'NONE',  ( 0.3862712429686727678, 1.188820645368945605, -3.333333333333333481 ) ) ;
#18894=CARTESIAN_POINT ( 'NONE',  ( 4.641001526964560142, 33.28196331604080171, -8.016098858316199838 ) ) ;
#18904=EDGE_LOOP ( 'NONE', ( #34791, #32999, #4315, #28176 ) ) ;
#18906=CARTESIAN_POINT ( 'NONE',  ( 0.4166666666666669072, 0.000000000000000000, -10.00000000000000000 ) ) ;
#18908=CARTESIAN_POINT ( 'NONE',  ( 0.6108107228405675881, -1.056024183042613140, 9.963925895596188909 ) ) ;
#18929=CARTESIAN_POINT ( 'NONE',  ( -3.566525152643847285, 1.569997364305458776, 9.741991644046965604 ) ) ;
#18932=ORIENTED_EDGE ( 'NONE', *, *, #46186, .T. ) ;
#18933=CARTESIAN_POINT ( 'NONE',  ( 17.43089236541784359, 28.36237856644539690, 3.199614146704519602 ) ) ;
#18941=CARTESIAN_POINT ( 'NONE',  ( 2.052549611693792464, -0.2039603569406628347, 9.894754715216725671 ) ) ;
#18942=CARTESIAN_POINT ( 'NONE',  ( -8.277096487746778308, 33.14818118907697198, 7.455576670931136185 ) ) ;
#18945=CARTESIAN_POINT ( 'NONE',  ( 31.46770792452135268, -38.94077080897339727, 3.199614146704519602 ) ) ;
#18953=CARTESIAN_POINT ( 'NONE',  ( 2.707743684961791075, 37.43817128298309882, -5.338708898921614043 ) ) ;
#18959=VECTOR ( 'NONE', #45636, 1000.000000000000114 ) ;
#18960=CARTESIAN_POINT ( 'NONE',  ( -1.424818880981866931, 0.8247269902860274726, 9.936700280135957186 ) ) ;
#18964=EDGE_CURVE ( 'NONE', #37517, #28949, #35378, .T. ) ;
#18968=VERTEX_POINT ( 'NONE', #41064 ) ;
#18983=CARTESIAN_POINT ( 'NONE',  ( -9.260964247899874380, 13.84230907185616744, -9.683996418299976483 ) ) ;
#18992=PLANE ( 'NONE',  #36609 ) ;
#18993=CARTESIAN_POINT ( 'NONE',  ( -27.73884755486766096, 25.23502201956265978, 7.697694107796191787 ) ) ;
#18994=ORIENTED_EDGE ( 'NONE', *, *, #41864, .F. ) ;
#18995=CARTESIAN_POINT ( 'NONE',  ( -22.69295089195507131, -45.31600496604688999, 7.455576670931136185 ) ) ;
#19008=CARTESIAN_POINT ( 'NONE',  ( 45.64490844644691236, 21.32281559348795952, 8.807470649214879543 ) ) ;
#19012=CARTESIAN_POINT ( 'NONE',  ( 1.780619886013945052, 1.041246721325614466, 9.886433018048068178 ) ) ;
#19013=CARTESIAN_POINT ( 'NONE',  ( -5.880994916442842779, -0.9650022442184716942, 5.692061405548898279E-16 ) ) ;
#19019=CARTESIAN_POINT ( 'NONE',  ( 14.91630425054810161, -7.943683830272122215, -9.008049429158100807 ) ) ;
#19021=CARTESIAN_POINT ( 'NONE',  ( -30.87089393895367095, 12.69923079256638587, -9.367992836599954742 ) ) ;
#19023=ADVANCED_FACE ( 'NONE', ( #29013 ), #11737, .T. ) ;
#19025=EDGE_CURVE ( 'NONE', #16759, #40675, #46309, .T. ) ;
#19027=CARTESIAN_POINT ( 'NONE',  ( -9.999626982420839028, -0.09954095390202467863, 8.968381510274571866 ) ) ;
#19030=B_SPLINE_CURVE_WITH_KNOTS ( 'NONE', 3,
 ( #18319, #46258, #10635, #34003 ),
 .UNSPECIFIED., .F., .F.,
 ( 4, 4 ),
 ( 0.001403500796105015694, 0.001586656765098967562 ),
 .UNSPECIFIED. ) ;
#19037=EDGE_LOOP ( 'NONE', ( #49117, #3508, #10419 ) ) ;
#19040=EDGE_CURVE ( 'NONE', #25169, #12217, #31648, .T. ) ;
#19042=AXIS2_PLACEMENT_3D ( 'NONE', #26710, #29106, #44726 ) ;
#19053=VERTEX_POINT ( 'NONE', #45885 ) ;
#19063=CARTESIAN_POINT ( 'NONE',  ( -25.63461350838931097, 43.17876197216396150, -8.016098858316205167 ) ) ;
#19085=B_SPLINE_SURFACE_WITH_KNOTS ( 'NONE', 3, 3, ( 
 ( #25416, #40563, #44384, #48953 ),
 ( #25675, #41317, #6167, #33630 ),
 ( #49217, #1567, #9260, #24916 ),
 ( #5401, #32880, #29012, #44626 ) ),
 .UNSPECIFIED., .F., .F., .F.,
 ( 4, 4 ),
 ( 4, 4 ),
 ( 0.000000000000000000, 1.000000000000000000 ),
 ( 0.000000000000000000, 1.000000000000000000 ),
 .UNSPECIFIED. ) ;
#19089=CARTESIAN_POINT ( 'NONE',  ( -49.89397392339119364, 8.245536726717011433, 7.906207997025717304 ) ) ;
#19092=ORIENTED_EDGE ( 'NONE', *, *, #11882, .F. ) ;
#19099=VECTOR ( 'NONE', #955, 999.9999999999998863 ) ;
#19105=ORIENTED_EDGE ( 'NONE', *, *, #46186, .F. ) ;
#19108=CARTESIAN_POINT ( 'NONE',  ( -1.249999999999999778, 0.000000000000000000, 3.333333333333333481 ) ) ;
#19113=CARTESIAN_POINT ( 'NONE',  ( 13.59579750444771307, -10.60877755095900632, 8.727788335465566760 ) ) ;
#19115=VERTEX_POINT ( 'NONE', #15891 ) ;
#19121=B_SPLINE_CURVE_WITH_KNOTS ( 'NONE', 3,
 ( #39552, #16444, #12839, #46938 ),
 .UNSPECIFIED., .F., .F.,
 ( 4, 4 ),
 ( 1.735570302229820823E-18, 8.326314924661348653E-06 ),
 .UNSPECIFIED. ) ;
#19124=CARTESIAN_POINT ( 'NONE',  ( -2.538055338523177440, -33.28424297489108596, -9.367992836599954742 ) ) ;
#19134=EDGE_CURVE ( 'NONE', #14725, #44231, #10799, .T. ) ;
#19144=CARTESIAN_POINT ( 'NONE',  ( -6.646097924775362209, 4.355953743238499598, 9.432811472610049819 ) ) ;
#19149=CARTESIAN_POINT ( 'NONE',  ( 0.3862712429686727678, 1.188820645368945605, -10.00000000000000000 ) ) ;
#19152=CARTESIAN_POINT ( 'NONE',  ( 1.035950918207909632, 50.00000000000000711, -2.408242355805840784 ) ) ;
#19153=CARTESIAN_POINT ( 'NONE',  ( 0.000000000000000000, 0.000000000000000000, 0.000000000000000000 ) ) ;
#19164=CARTESIAN_POINT ( 'NONE',  ( -1.377509002708424468, 0.6027468487255034368, 9.927319414211229542 ) ) ;
#19165=ORIENTED_EDGE ( 'NONE', *, *, #17752, .T. ) ;
#19169=CARTESIAN_POINT ( 'NONE',  ( 3.231548175622897645, -9.463461120997347820, 9.282506307616472441 ) ) ;
#19179=CARTESIAN_POINT ( 'NONE',  ( -50.11058929355264979, 7.578863168071929834, 7.455576670931136185 ) ) ;
#19183=CARTESIAN_POINT ( 'NONE',  ( 1.275994128725544741, -0.1230186051320594776, 9.948547179989619238 ) ) ;
#19187=ORIENTED_EDGE ( 'NONE', *, *, #18593, .F. ) ;
#19194=CARTESIAN_POINT ( 'NONE',  ( 0.4266413953668419246, 1.250184266969606162, 9.943883492372851407 ) ) ;
#19198=CARTESIAN_POINT ( 'NONE',  ( -1.133908876584336367, -0.5183204401656656968, 9.981352469109934233 ) ) ;
#19210=CARTESIAN_POINT ( 'NONE',  ( -17.43089236541806031, -28.36237856644526900, 3.199614146704519602 ) ) ;
#19215=CARTESIAN_POINT ( 'NONE',  ( 47.22310614333766665, 16.46562252335956344, -3.760136334089591248 ) ) ;
#19220=CARTESIAN_POINT ( 'NONE',  ( 33.43156050989131955, -4.370686678976570150, 8.807470649214879543 ) ) ;
#19236=CARTESIAN_POINT ( 'NONE',  ( -1.011271242968683426, -0.7347315653655928092, 10.00000000000000000 ) ) ;
#19241=CARTESIAN_POINT ( 'NONE',  ( -32.57170742938676256, -18.58316106410400437, 7.697694107796192675 ) ) ;
#19244=CARTESIAN_POINT ( 'NONE',  ( -17.34922095635781147, -33.24536858281880569, 8.914903342594564961 ) ) ;
#19255=CARTESIAN_POINT ( 'NONE',  ( -48.98697415750977768, -11.03699497439218291, -8.016098858316205167 ) ) ;
#19267=CARTESIAN_POINT ( 'NONE',  ( 14.76429217231961566, 8.192625680377691566, 9.178419661560148768 ) ) ;
#19277=ORIENTED_EDGE ( 'NONE', *, *, #35989, .T. ) ;
#19297=VECTOR ( 'NONE', #12465, 1000.000000000000000 ) ;
#19313=VERTEX_POINT ( 'NONE', #1509 ) ;
#19320=CARTESIAN_POINT ( 'NONE',  ( 1.011271242968688311, -0.7347315653655855927, -10.00000000000000000 ) ) ;
#19327=EDGE_CURVE ( 'NONE', #18968, #16979, #24904, .T. ) ;
#19334=CARTESIAN_POINT ( 'NONE',  ( -23.79193388295331602, -28.98609808354994044, -9.422646554964178023 ) ) ;
#19342=ORIENTED_EDGE ( 'NONE', *, *, #49413, .F. ) ;
#19347=CARTESIAN_POINT ( 'NONE',  ( 4.672045878990125800, -33.19353511768168374, 1.847720168420772691 ) ) ;
#19366=CARTESIAN_POINT ( 'NONE',  ( 27.33593271309472073, -41.94268121623323964, -9.367992836599954742 ) ) ;
#19368=CARTESIAN_POINT ( 'NONE',  ( 1.011271242968688311, -0.7347315653655855927, 3.333333333333333481 ) ) ;
#19370=EDGE_LOOP ( 'NONE', ( #34303, #29542, #10365, #8979, #37329 ) ) ;
#19374=CARTESIAN_POINT ( 'NONE',  ( 8.277096487746778308, -33.14818118907697198, 7.455576670931136185 ) ) ;
#19378=CARTESIAN_POINT ( 'NONE',  ( -3.996390545799824334, 16.57371371864897469, 8.953103998512858652 ) ) ;
#19380=VERTEX_POINT ( 'NONE', #12794 ) ;
#19400=ORIENTED_EDGE ( 'NONE', *, *, #34934, .F. ) ;
#19405=EDGE_CURVE ( 'NONE', #8523, #9153, #13877, .T. ) ;
#19408=CARTESIAN_POINT ( 'NONE',  ( 0.2050626648100478400, -1.807624707196173519, 9.903764339332001398 ) ) ;
#19415=B_SPLINE_CURVE_WITH_KNOTS ( 'NONE', 3,
 ( #19645, #12200, #46800, #657 ),
 .UNSPECIFIED., .F., .F.,
 ( 4, 4 ),
 ( 0.000000000000000000, 0.0004154657329505417928 ),
 .UNSPECIFIED. ) ;
#19421=CARTESIAN_POINT ( 'NONE',  ( -49.89397392339119364, 8.245536726717011433, 7.906207997025717304 ) ) ;
#19428=CARTESIAN_POINT ( 'NONE',  ( 2.538055338523173443, 50.00000000000000711, -9.367992836599951190 ) ) ;
#19435=EDGE_LOOP ( 'NONE', ( #49311, #19935, #19092, #17315 ) ) ;
#19436=ADVANCED_FACE ( 'NONE', ( #17648 ), #47771, .T. ) ;
#19442=EDGE_LOOP ( 'NONE', ( #46230, #30645, #35717, #43100 ) ) ;
#19454=CARTESIAN_POINT ( 'NONE',  ( -0.3862712429686809279, -1.188820645368942941, 9.972675548442463622 ) ) ;
#19461=CARTESIAN_POINT ( 'NONE',  ( -1.377594142017869450, 0.6023266041008150662, 9.944962737616616977 ) ) ;
#19474=CARTESIAN_POINT ( 'NONE',  ( -0.3862712429686809279, -1.188820645368943163, 10.00000000000000000 ) ) ;
#19482=VERTEX_POINT ( 'NONE', #25858 ) ;
#19491=CARTESIAN_POINT ( 'NONE',  ( -30.25247992116029394, 39.82368563463828792, -3.760136334089591248 ) ) ;
#19494=EDGE_LOOP ( 'NONE', ( #12019, #47500, #7905, #11897, #12626, #33085, #33772, #29099, #3654, #34225, #28119, #44884, #26920, #33231 ) ) ;
#19498=CARTESIAN_POINT ( 'NONE',  ( -1.035950918207909632, -50.00000000000000711, -2.408242355805840784 ) ) ;
#19503=CARTESIAN_POINT ( 'NONE',  ( 32.57170742938662755, 18.58316106410423174, 7.697694107796188234 ) ) ;
#19504=B_SPLINE_SURFACE_WITH_KNOTS ( 'NONE', 3, 3, ( 
 ( #3055, #42058, #33374, #5901 ),
 ( #30024, #21550, #37238, #6916 ),
 ( #22559, #17705, #10505, #41559 ),
 ( #38240, #18194, #10005, #25667 ) ),
 .UNSPECIFIED., .F., .F., .F.,
 ( 4, 4 ),
 ( 4, 4 ),
 ( 0.000000000000000000, 1.000000000000000000 ),
 ( 0.000000000000000000, 1.000000000000000000 ),
 .UNSPECIFIED. ) ;
#19507=CARTESIAN_POINT ( 'NONE',  ( -48.33712804702535948, -13.03701565032741883, -9.367992836599951190 ) ) ;
#19514=CARTESIAN_POINT ( 'NONE',  ( 13.59579750444771307, -10.60877755095900632, 8.727788335465566760 ) ) ;
#19524=CARTESIAN_POINT ( 'NONE',  ( 10.30302290646030627, 13.08520913973580058, -9.683996418299976483 ) ) ;
#19526=CARTESIAN_POINT ( 'NONE',  ( 33.43156050989131955, -4.370686678976570150, 8.807470649214879543 ) ) ;
#19541=CARTESIAN_POINT ( 'NONE',  ( 32.00969891772083287, 38.54699130261819562, -8.917361510505369182 ) ) ;
#19546=ADVANCED_FACE ( 'NONE', ( #23003 ), #22773, .T. ) ;
#19550=CARTESIAN_POINT ( 'NONE',  ( -0.1475726264153620626, -1.496347932843211215, 9.927319414211227766 ) ) ;
#19569=CARTESIAN_POINT ( 'NONE',  ( -15.44803555374685189, -6.237487519713257100, -3.546734833711462365 ) ) ;
#19571=ADVANCED_FACE ( 'NONE', ( #438 ), #46081, .T. ) ;
#19574=CARTESIAN_POINT ( 'NONE',  ( 0.6440276692615888310, 16.64212148744554298, -9.683996418299976483 ) ) ;
#19578=EDGE_LOOP ( 'NONE', ( #43998, #50420, #26854, #28007 ) ) ;
#19581=B_SPLINE_CURVE_WITH_KNOTS ( 'NONE', 3,
 ( #48705, #1813, #41059, #41561 ),
 .UNSPECIFIED., .F., .F.,
 ( 4, 4 ),
 ( 1.735570302229820823E-18, 8.326314924663078294E-06 ),
 .UNSPECIFIED. ) ;
#19584=CARTESIAN_POINT ( 'NONE',  ( -22.51959565330812296, -30.03043964857251780, -6.568693074176339408 ) ) ;
#19597=ORIENTED_EDGE ( 'NONE', *, *, #30625, .T. ) ;
#19601=B_SPLINE_CURVE_WITH_KNOTS ( 'NONE', 3,
 ( #40777, #32332, #44585, #9468 ),
 .UNSPECIFIED., .F., .F.,
 ( 4, 4 ),
 ( 0.01012863361515542113, 0.01015667504234211982 ),
 .UNSPECIFIED. ) ;
#19606=CARTESIAN_POINT ( 'NONE',  ( 33.57695195286775913, 16.69845195084893064, 8.914903342594561408 ) ) ;
#19618=EDGE_CURVE ( 'NONE', #12550, #7144, #50471, .T. ) ;
#19620=EDGE_CURVE ( 'NONE', #12768, #18535, #10167, .T. ) ;
#19621=ORIENTED_EDGE ( 'NONE', *, *, #46014, .F. ) ;
#19626=CARTESIAN_POINT ( 'NONE',  ( -6.196515397221703303, -4.974751005920792224, 9.432811472610147518 ) ) ;
#19630=CARTESIAN_POINT ( 'NONE',  ( -8.277096487746778308, 50.00000000000000711, 7.455576670931136185 ) ) ;
#19636=VECTOR ( 'NONE', #42078, 999.9999999999998863 ) ;
#19642=CARTESIAN_POINT ( 'NONE',  ( 1.066995270233474624, -33.23888904628638841, -3.760136334089591248 ) ) ;
#19645=CARTESIAN_POINT ( 'NONE',  ( -1.448406091252275818, 0.9360325558308429938, 9.928159647716187308 ) ) ;
#19647=ORIENTED_EDGE ( 'NONE', *, *, #50041, .F. ) ;
#19654=CARTESIAN_POINT ( 'NONE',  ( -0.3862712429686977478, 1.188820645368937390, 10.00000000000000000 ) ) ;
#19667=CARTESIAN_POINT ( 'NONE',  ( 16.50002041759926286, 3.070736177214647977, -9.233365092205394475 ) ) ;
#19669=CARTESIAN_POINT ( 'NONE',  ( 1.011271242968677653, 0.7347315653656002477, 10.00000000000000000 ) ) ;
#19670=CARTESIAN_POINT ( 'NONE',  ( -17.23491422248386584, 0.5912720620001978844, 8.727788335465566760 ) ) ;
#19687=ORIENTED_EDGE ( 'NONE', *, *, #37885, .F. ) ;
#19689=ORIENTED_EDGE ( 'NONE', *, *, #9385, .T. ) ;
#19691=CARTESIAN_POINT ( 'NONE',  ( 29.61572577327002520, 16.11461842845735859, 8.807470649214879543 ) ) ;
#19699=EDGE_CURVE ( 'NONE', #25517, #43044, #17535, .T. ) ;
#19711=CARTESIAN_POINT ( 'NONE',  ( 23.31729631074197329, 24.19776167542427814, -8.016098858316199838 ) ) ;
#19715=CARTESIAN_POINT ( 'NONE',  ( -23.29043492822808759, 24.10797434788186067, 1.847720168420772691 ) ) ;
#19716=CARTESIAN_POINT ( 'NONE',  ( 9.999999999999994671, -1.084202172485504187E-16, 9.303249460322209785 ) ) ;
#19734=CARTESIAN_POINT ( 'NONE',  ( -23.79193388295331602, -28.98609808354994044, -9.422646554964178023 ) ) ;
#19738=CARTESIAN_POINT ( 'NONE',  ( -16.99749102614300966, 1.320765928724422222, 8.953103998512858652 ) ) ;
#19752=EDGE_CURVE ( 'NONE', #39413, #45145, #23620, .T. ) ;
#19757=DIRECTION ( 'NONE',  ( 0.000000000000000000, 0.000000000000000000, -1.000000000000000000 ) ) ;
#19771=CARTESIAN_POINT ( 'NONE',  ( -1.073226156958101862, -0.6788500330460245369, 9.975314328424618182 ) ) ;
#19772=CARTESIAN_POINT ( 'NONE',  ( -0.3862712429686895876, 1.188820645368940720, -10.00000000000000000 ) ) ;
#19776=CARTESIAN_POINT ( 'NONE',  ( 0.3862712429686727678, 1.188820645368945605, 10.00000000000000000 ) ) ;
#19782=VECTOR ( 'NONE', #36147, 1000.000000000000000 ) ;
#19786=CARTESIAN_POINT ( 'NONE',  ( -4.641001526964561030, -50.00000000000000000, -8.016098858316205167 ) ) ;
#19788=CARTESIAN_POINT ( 'NONE',  ( 2.538055338523173443, 50.00000000000000000, -9.367992836599951190 ) ) ;
#19798=DIRECTION ( 'NONE',  ( 1.000000000000000000, 0.000000000000000000, -0.000000000000000000 ) ) ;
#19807=ORIENTED_EDGE ( 'NONE', *, *, #15552, .T. ) ;
#19812=LINE ( 'NONE', #27274, #37372 ) ;
#19827=B_SPLINE_CURVE_WITH_KNOTS ( 'NONE', 3,
 ( #50312, #38589, #30889, #31392, #27541, #344 ),
 .UNSPECIFIED., .F., .F.,
 ( 4, 2, 4 ),
 ( 4.906538933386797396E-18, 0.009877169331704833619, 0.01975433866340966030 ),
 .UNSPECIFIED. ) ;
#19828=CARTESIAN_POINT ( 'NONE',  ( -1.011271242968688533, 0.7347315653655859258, 10.00000000000000000 ) ) ;
#19829=CARTESIAN_POINT ( 'NONE',  ( -8.277096487746778308, 33.14818118907697198, 7.455576670931136185 ) ) ;
#19853=CARTESIAN_POINT ( 'NONE',  ( -3.441214337941710610, 1.549069628443896285, 9.865049507598756762 ) ) ;
#19877=ORIENTED_EDGE ( 'NONE', *, *, #31485, .T. ) ;
#19883=ORIENTED_EDGE ( 'NONE', *, *, #18868, .F. ) ;
#19884=ORIENTED_EDGE ( 'NONE', *, *, #25759, .F. ) ;
#19885=EDGE_LOOP ( 'NONE', ( #26726, #40920, #41818, #39206, #45979 ) ) ;
#19889=CARTESIAN_POINT ( 'NONE',  ( 4.672045878990125800, -33.19353511768168374, 1.847720168420772691 ) ) ;
#19891=CARTESIAN_POINT ( 'NONE',  ( 16.91580242619102137, 33.50775492265647415, 4.835783797351798974 ) ) ;
#19902=EDGE_LOOP ( 'NONE', ( #22783, #8631, #34930 ) ) ;
#19907=EDGE_CURVE ( 'NONE', #3402, #26155, #32815, .T. ) ;
#19911=ADVANCED_FACE ( 'NONE', ( #49376 ), #43701, .T. ) ;
#19918=CARTESIAN_POINT ( 'NONE',  ( 1.250000000000000222, 0.000000000000000000, -3.333333333333333481 ) ) ;
#19919=EDGE_CURVE ( 'NONE', #3733, #1058, #13783, .T. ) ;
#19928=CARTESIAN_POINT ( 'NONE',  ( 49.46074318306830975, -9.578883844006831794, 8.807470649214879543 ) ) ;
#19933=B_SPLINE_SURFACE_WITH_KNOTS ( 'NONE', 3, 3, ( 
 ( #12804, #17407, #48654, #28709 ),
 ( #4609, #33075, #39767, #8720 ),
 ( #21256, #25116, #44084, #16918 ),
 ( #32825, #28210, #8956, #28465 ) ),
 .UNSPECIFIED., .F., .F., .F.,
 ( 4, 4 ),
 ( 4, 4 ),
 ( 0.000000000000000000, 1.000000000000000000 ),
 ( 0.000000000000000000, 1.000000000000000000 ),
 .UNSPECIFIED. ) ;
#19935=ORIENTED_EDGE ( 'NONE', *, *, #10247, .F. ) ;
#19949=CARTESIAN_POINT ( 'NONE',  ( -0.3862712429686809279, -1.188820645368943163, 10.00000000000000000 ) ) ;
#19960=CARTESIAN_POINT ( 'NONE',  ( -0.5107275442771143092, -1.175643901748072873, 9.976582533991681601 ) ) ;
#19968=CARTESIAN_POINT ( 'NONE',  ( -0.1083801931742817276, -1.382014125000175397, 9.960033073700733652 ) ) ;
#19969=CARTESIAN_POINT ( 'NONE',  ( -1.081517186030697797, 0.5722085955955610315, 9.993783931180535873 ) ) ;
#19978=CARTESIAN_POINT ( 'NONE',  ( -0.9390173899430289683, -1.130417317737636651, 9.958264684458541183 ) ) ;
#19987=CARTESIAN_POINT ( 'NONE',  ( 0.1287570809895604018, 0.3962735484563146282, 10.00000000000000000 ) ) ;
#19992=CARTESIAN_POINT ( 'NONE',  ( 16.99749102614301677, -1.320765928724307425, 8.953103998512858652 ) ) ;
#20000=CARTESIAN_POINT ( 'NONE',  ( 32.57170742938662755, 18.58316106410423174, 7.697694107796188234 ) ) ;
#20006=EDGE_LOOP ( 'NONE', ( #22544, #21166, #146, #43994, #42768 ) ) ;
#20022=VERTEX_POINT ( 'NONE', #154 ) ;
#20036=CARTESIAN_POINT ( 'NONE',  ( -11.73320209285699889, 11.96063479729179768, 9.403735324607438884 ) ) ;
#20037=ORIENTED_EDGE ( 'NONE', *, *, #38254, .F. ) ;
#20044=CARTESIAN_POINT ( 'NONE',  ( -1.578643388466005160, 1.550786058692512182, 9.881002359080275355 ) ) ;
#20045=CARTESIAN_POINT ( 'NONE',  ( -17.51065725283106289, 28.41934970907792746, -9.367992836599954742 ) ) ;
#20046=CARTESIAN_POINT ( 'NONE',  ( 21.61731705588930907, 25.43568671410602278, -9.367992836599954742 ) ) ;
#20048=ADVANCED_FACE ( 'NONE', ( #27089 ), #11316, .T. ) ;
#20057=CARTESIAN_POINT ( 'NONE',  ( -9.999999999999994671, 2.168404344971008375E-16, 8.340239149799208107 ) ) ;
#20064=CARTESIAN_POINT ( 'NONE',  ( 0.3965304326644019106, -0.1288405477284165490, 9.992737347336296594 ) ) ;
#20074=EDGE_LOOP ( 'NONE', ( #24263, #49383, #32703, #48856 ) ) ;
#20081=ORIENTED_EDGE ( 'NONE', *, *, #2658, .T. ) ;
#20098=CARTESIAN_POINT ( 'NONE',  ( -28.96803024440907137, -18.11533787072017176, 7.455576670931136185 ) ) ;
#20105=CARTESIAN_POINT ( 'NONE',  ( 1.066995270233474624, -50.00000000000000711, -3.760136334089591248 ) ) ;
#20111=CARTESIAN_POINT ( 'NONE',  ( -9.483938762529191990, 3.217310375392813615, 3.215106848023462138 ) ) ;
#20117=ORIENTED_EDGE ( 'NONE', *, *, #23029, .T. ) ;
#20130=CARTESIAN_POINT ( 'NONE',  ( 47.23269937569327226, -16.43609759007049931, -2.408242355805840784 ) ) ;
#20135=CARTESIAN_POINT ( 'NONE',  ( 6.408332700304398166, 7.676800896350598258, 0.000000000000000000 ) ) ;
#20136=CARTESIAN_POINT ( 'NONE',  ( 34.95136153415558056, -36.40974830873469870, 8.356839323120299312 ) ) ;
#20142=ORIENTED_EDGE ( 'NONE', *, *, #11749, .T. ) ;
#20149=ORIENTED_EDGE ( 'NONE', *, *, #3088, .F. ) ;
#20151=CARTESIAN_POINT ( 'NONE',  ( -18.67411147745623978, -27.51799019669813973, -3.760136334089591248 ) ) ;
#20156=FACE_OUTER_BOUND ( 'NONE', #34154, .T. ) ;
#20163=VECTOR ( 'NONE', #18124, 1000.000000000000114 ) ;
#20170=CARTESIAN_POINT ( 'NONE',  ( 0.3862712429686978033, -1.188820645368937834, -10.00000000000000000 ) ) ;
#20178=CARTESIAN_POINT ( 'NONE',  ( -1.593403307199984020, -0.6097984806593539364, 9.912102921405034905 ) ) ;
#20184=CARTESIAN_POINT ( 'NONE',  ( 0.3147652639080171233, -1.255102005797306575, 9.947020512645400103 ) ) ;
#20188=DIRECTION ( 'NONE',  ( 0.5877852522924743583, -0.8090169943749466741, 0.000000000000000000 ) ) ;
#20193=VERTEX_POINT ( 'NONE', #47308 ) ;
#20200=VERTEX_POINT ( 'NONE', #6004 ) ;
#20211=CARTESIAN_POINT ( 'NONE',  ( 1.011271242968688311, -0.7347315653655855927, -3.333333333333333481 ) ) ;
#20213=CARTESIAN_POINT ( 'NONE',  ( 11.73320209285708415, -11.96063479729170886, 9.403735324607438884 ) ) ;
#20232=DIRECTION ( 'NONE',  ( -0.6805276818820470419, 0.4944323023721968191, -0.5407575913134976542 ) ) ;
#20244=CARTESIAN_POINT ( 'NONE',  ( 31.28234235046230793, 11.28615439405779064, -3.760136334089591248 ) ) ;
#20246=ORIENTED_EDGE ( 'NONE', *, *, #50617, .T. ) ;
#20248=B_SPLINE_CURVE_WITH_KNOTS ( 'NONE', 3,
 ( #34781, #30927, #7565, #17023 ),
 .UNSPECIFIED., .F., .F.,
 ( 4, 4 ),
 ( 0.001937412222931638979, 0.003978261222109142140 ),
 .UNSPECIFIED. ) ;
#20253=CARTESIAN_POINT ( 'NONE',  ( -1.267276237729528798, 0.08162529406826846134, 9.975314328424614629 ) ) ;
#20254=CARTESIAN_POINT ( 'NONE',  ( -36.28567981536816234, -9.465698090293395595, -9.422646554964174470 ) ) ;
#20264=ORIENTED_EDGE ( 'NONE', *, *, #44586, .F. ) ;
#20266=CARTESIAN_POINT ( 'NONE',  ( 46.76852358249013264, -17.86468378716708827, -9.367992836599951190 ) ) ;
#20278=EDGE_LOOP ( 'NONE', ( #35823, #696, #5495 ) ) ;
#20282=CARTESIAN_POINT ( 'NONE',  ( -0.1287570809895632329, 0.3962735484563137400, -10.00000000000000000 ) ) ;
#20289=CARTESIAN_POINT ( 'NONE',  ( -24.47767542868268364, 23.18653802921800278, 8.807470649214879543 ) ) ;
#20302=CARTESIAN_POINT ( 'NONE',  ( 2.143303251558809297, -0.2857918750720293000, 9.885585981620947038 ) ) ;
#20307=CARTESIAN_POINT ( 'NONE',  ( 34.95136153415558056, -36.40974830873469870, 8.356839323120299312 ) ) ;
#20316=CARTESIAN_POINT ( 'NONE',  ( 27.33593271309472073, -41.94268121623323253, -9.367992836599951190 ) ) ;
#20322=CARTESIAN_POINT ( 'NONE',  ( -36.97942854200451990, 6.226705766838657397, 8.914903342594564961 ) ) ;
#20332=CARTESIAN_POINT ( 'NONE',  ( 0.5953091702432292687, 3.900377598923890243, 6.494306381704024744 ) ) ;
#20344=DIRECTION ( 'NONE',  ( 0.000000000000000000, -0.000000000000000000, -1.000000000000000000 ) ) ;
#20347=ORIENTED_EDGE ( 'NONE', *, *, #26070, .F. ) ;
#20352=CARTESIAN_POINT ( 'NONE',  ( 3.231548175622897645, -9.463461120997347820, 9.282506307616472441 ) ) ;
#20353=CARTESIAN_POINT ( 'NONE',  ( 1.647520908219943792, -0.4432416309287623979, 9.912102921405036682 ) ) ;
#20360=B_SPLINE_SURFACE_WITH_KNOTS ( 'NONE', 3, 3, ( 
 ( #115, #42935, #7553, #45997 ),
 ( #15746, #39124, #38614, #31161 ),
 ( #18571, #14735, #11150, #35028 ),
 ( #31416, #50599, #30652, #34247 ) ),
 .UNSPECIFIED., .F., .F., .F.,
 ( 4, 4 ),
 ( 4, 4 ),
 ( 0.000000000000000000, 1.000000000000000000 ),
 ( 0.000000000000000000, 1.000000000000000000 ),
 .UNSPECIFIED. ) ;
#20366=ORIENTED_EDGE ( 'NONE', *, *, #33425, .F. ) ;
#20368=B_SPLINE_CURVE_WITH_KNOTS ( 'NONE', 3,
 ( #34332, #25625, #30222, #37197 ),
 .UNSPECIFIED., .F., .F.,
 ( 4, 4 ),
 ( 0.003717746584991899611, 0.009855832532552960198 ),
 .UNSPECIFIED. ) ;
#20393=CARTESIAN_POINT ( 'NONE',  ( 1.011271242968683648, 0.7347315653655930312, 3.333333333333333481 ) ) ;
#20397=FACE_OUTER_BOUND ( 'NONE', #48626, .T. ) ;
#20398=CARTESIAN_POINT ( 'NONE',  ( 14.76429217231961566, 8.192625680377691566, 9.178419661560148768 ) ) ;
#20401=LINE ( 'NONE', #24781, #28251 ) ;
#20414=CARTESIAN_POINT ( 'NONE',  ( -31.94178169330213279, 9.256608784834037706, -3.760136334089591248 ) ) ;
#20416=CARTESIAN_POINT ( 'NONE',  ( -21.58778298521296080, 25.34222074689773407, 3.199614146704519602 ) ) ;
#20430=ORIENTED_EDGE ( 'NONE', *, *, #50402, .F. ) ;
#20452=CARTESIAN_POINT ( 'NONE',  ( -7.929028342769414373, 0.8360401409709390386, 1.626303258728256651E-16 ) ) ;
#20456=ORIENTED_EDGE ( 'NONE', *, *, #47464, .F. ) ;
#20458=B_SPLINE_CURVE_WITH_KNOTS ( 'NONE', 3,
 ( #11901, #38605, #50590, #34759 ),
 .UNSPECIFIED., .F., .F.,
 ( 4, 4 ),
 ( 0.0003760194760206631058, 0.0006307719036365294499 ),
 .UNSPECIFIED. ) ;
#20465=EDGE_CURVE ( 'NONE', #21273, #16032, #5161, .T. ) ;
#20485=CARTESIAN_POINT ( 'NONE',  ( 33.14391172085757375, 37.72293746533118508, -8.016098858316205167 ) ) ;
#20497=CARTESIAN_POINT ( 'NONE',  ( -1.337801958641930300, -1.088266084286974689, 9.928159647716134018 ) ) ;
#20504=ORIENTED_EDGE ( 'NONE', *, *, #39172, .T. ) ;
#20506=B_SPLINE_CURVE_WITH_KNOTS ( 'NONE', 3,
 ( #14134, #10797, #11057, #17751 ),
 .UNSPECIFIED., .F., .F.,
 ( 4, 4 ),
 ( 0.0002936521407533901036, 0.0006663369986142128176 ),
 .UNSPECIFIED. ) ;
#20516=CARTESIAN_POINT ( 'NONE',  ( -34.38425513258694366, 36.82177522737846687, 8.807470649214879543 ) ) ;
#20523=FACE_OUTER_BOUND ( 'NONE', #26457, .T. ) ;
#20526=CARTESIAN_POINT ( 'NONE',  ( -1.080000014127418639, -0.7606467978654640749, 9.943883492372872723 ) ) ;
#20532=FACE_OUTER_BOUND ( 'NONE', #15544, .T. ) ;
#20533=DIRECTION ( 'NONE',  ( 1.000000000000000000, 0.000000000000000000, 0.000000000000000000 ) ) ;
#20540=CARTESIAN_POINT ( 'NONE',  ( -34.38425513258695077, 36.82177522737848108, 8.807470649214879543 ) ) ;
#20548=EDGE_CURVE ( 'NONE', #49029, #5524, #12524, .T. ) ;
#20552=ORIENTED_EDGE ( 'NONE', *, *, #12224, .F. ) ;
#20553=EDGE_CURVE ( 'NONE', #38616, #17359, #32711, .T. ) ;
#20558=CARTESIAN_POINT ( 'NONE',  ( 0.5109188679997901383, 1.175605252300628623, 9.967237415621765351 ) ) ;
#20561=CARTESIAN_POINT ( 'NONE',  ( -0.4266413953668892756, -1.250184266969579294, 9.943883492372849631 ) ) ;
#20566=AXIS2_PLACEMENT_3D ( 'NONE', #50672, #35099, #27129 ) ;
#20575=CARTESIAN_POINT ( 'NONE',  ( 33.86622497129647513, -3.037805405904928868, 7.906207997025717304 ) ) ;
#20595=ORIENTED_EDGE ( 'NONE', *, *, #42830, .F. ) ;
#20606=CARTESIAN_POINT ( 'NONE',  ( 3.345242017215822372, -2.159124855890657724, -4.878909776184769953E-16 ) ) ;
#20613=CARTESIAN_POINT ( 'NONE',  ( -2.538055338523177440, -50.00000000000000711, -9.367992836599954742 ) ) ;
#20616=ADVANCED_FACE ( 'NONE', ( #5692 ), #1133, .T. ) ;
#20622=CARTESIAN_POINT ( 'NONE',  ( 33.43156050989131955, -4.370686678976570150, 8.807470649214879543 ) ) ;
#20636=CARTESIAN_POINT ( 'NONE',  ( 7.787882027935128626, 1.707024178319727969, -2.642742795433417058E-16 ) ) ;
#20638=ORIENTED_EDGE ( 'NONE', *, *, #6276, .T. ) ;
#20640=CARTESIAN_POINT ( 'NONE',  ( -0.4402948852767746279, 2.015117899693936732, 9.894754715216722118 ) ) ;
#20646=CARTESIAN_POINT ( 'NONE',  ( 45.64490844644691236, 21.32281559348795952, 8.807470649214879543 ) ) ;
#20651=EDGE_CURVE ( 'NONE', #41040, #30921, #3338, .T. ) ;
#20658=CARTESIAN_POINT ( 'NONE',  ( 45.64490844644691236, 21.32281559348795952, 8.807470649214879543 ) ) ;
#20672=B_SPLINE_CURVE_WITH_KNOTS ( 'NONE', 3,
 ( #28639, #24803, #37126, #17598 ),
 .UNSPECIFIED., .F., .F.,
 ( 4, 4 ),
 ( 0.9811748202683100439, 0.9878904167554126703 ),
 .UNSPECIFIED. ) ;
#20674=FACE_OUTER_BOUND ( 'NONE', #47258, .T. ) ;
#20676=B_SPLINE_SURFACE_WITH_KNOTS ( 'NONE', 3, 3, ( 
 ( #30033, #44877, #10760, #48952 ),
 ( #49216, #49472, #18200, #26414 ),
 ( #2806, #17946, #41565, #22061 ),
 ( #33629, #25673, #45638, #33881 ) ),
 .UNSPECIFIED., .F., .F., .F.,
 ( 4, 4 ),
 ( 4, 4 ),
 ( 0.000000000000000000, 1.000000000000000000 ),
 ( 0.000000000000000000, 1.000000000000000000 ),
 .UNSPECIFIED. ) ;
#20679=CARTESIAN_POINT ( 'NONE',  ( -28.96803024440907137, -18.11533787072017176, 7.455576670931136185 ) ) ;
#20681=EDGE_CURVE ( 'NONE', #44030, #25517, #5802, .T. ) ;
#20682=CARTESIAN_POINT ( 'NONE',  ( -0.9000089392641369423, -1.054368634403656690, 9.960033073700792272 ) ) ;
#20683=AXIS2_PLACEMENT_3D ( 'NONE', #6626, #37953, #7853 ) ;
#20684=CARTESIAN_POINT ( 'NONE',  ( -1.962539651752354564, 0.2571568065648870971, 9.897807938190499755 ) ) ;
#20685=CARTESIAN_POINT ( 'NONE',  ( 15.42815683172628738, 34.17926237904582365, 7.697694107796191787 ) ) ;
#20692=CARTESIAN_POINT ( 'NONE',  ( 5.930385588435886923, -41.38048276556310157, 8.846626183609801686 ) ) ;
#20698=CARTESIAN_POINT ( 'NONE',  ( -33.43156050989129824, 4.370686678976795747, 8.807470649214879543 ) ) ;
#20709=ADVANCED_FACE ( 'NONE', ( #6448, #34946, #18740, #22104, #2840, #42357 ), #15422, .T. ) ;
#20710=CARTESIAN_POINT ( 'NONE',  ( -1.249999999999999778, 0.000000000000000000, -10.00000000000000000 ) ) ;
#20711=CARTESIAN_POINT ( 'NONE',  ( -19.52505477809972945, -36.96330698207071919, 8.846626183609801686 ) ) ;
#20712=CARTESIAN_POINT ( 'NONE',  ( -1.170692300221099824, -0.8653481604899971869, 9.938560165450807560 ) ) ;
#20715=CARTESIAN_POINT ( 'NONE',  ( -0.3370904143228978245, 0.2449105217885259589, 10.00000000000000000 ) ) ;
#20716=VERTEX_POINT ( 'NONE', #45419 ) ;
#20719=CARTESIAN_POINT ( 'NONE',  ( -1.468713901642213493, -0.3220470327672489419, 9.927319414211227766 ) ) ;
#20721=CARTESIAN_POINT ( 'NONE',  ( -1.962712821592842882, -1.022159834731130257, 9.881002359080275355 ) ) ;
#20727=CARTESIAN_POINT ( 'NONE',  ( -0.6126904405382037622, -1.085824959725731231, 9.981352469109934233 ) ) ;
#20748=CARTESIAN_POINT ( 'NONE',  ( 1.011271242968688311, -0.7347315653655855927, -10.00000000000000000 ) ) ;
#20753=VERTEX_POINT ( 'NONE', #18500 ) ;
#20757=CARTESIAN_POINT ( 'NONE',  ( -7.749480817862350435, -14.85497772329513211, 9.403735324607438884 ) ) ;
#20776=B_SPLINE_SURFACE_WITH_KNOTS ( 'NONE', 3, 3, ( 
 ( #50641, #15546, #11691, #31457 ),
 ( #42980, #43241, #8106, #39162 ),
 ( #3992, #39419, #37287, #25969 ),
 ( #29051, #21342, #33661, #36773 ) ),
 .UNSPECIFIED., .F., .F., .F.,
 ( 4, 4 ),
 ( 4, 4 ),
 ( 0.000000000000000000, 1.000000000000000000 ),
 ( 0.000000000000000000, 1.000000000000000000 ),
 .UNSPECIFIED. ) ;
#20779=CARTESIAN_POINT ( 'NONE',  ( -25.04522487443065160, 22.77512090857326754, 8.356839323120299312 ) ) ;
#20781=CARTESIAN_POINT ( 'NONE',  ( -1.011271242968693862, 0.7347315653655780432, 10.00000000000000000 ) ) ;
#20782=VERTEX_POINT ( 'NONE', #34429 ) ;
#20804=EDGE_LOOP ( 'NONE', ( #32977, #28766, #48811 ) ) ;
#20807=CARTESIAN_POINT ( 'NONE',  ( 12.97493236725083676, -11.05939663306990717, 8.953103998512858652 ) ) ;
#20816=CARTESIAN_POINT ( 'NONE',  ( -6.219530239386607207, 7.848697864701671634, 6.429802539306387565 ) ) ;
#20819=CARTESIAN_POINT ( 'NONE',  ( 1.769963848780946369, -9.842115015280432644, 0.000000000000000000 ) ) ;
#20822=CARTESIAN_POINT ( 'NONE',  ( 14.29087950072012170, 9.652079258044652832, 8.727788335465566760 ) ) ;
#20828=EDGE_CURVE ( 'NONE', #12798, #49396, #21068, .T. ) ;
#20837=EDGE_CURVE ( 'NONE', #22255, #290, #49195, .T. ) ;
#20842=CARTESIAN_POINT ( 'NONE',  ( 1.158497635116737312, -16.61944452314319420, -3.546734833711462365 ) ) ;
#20856=CARTESIAN_POINT ( 'NONE',  ( -3.229232847726260403, 16.57333684275945629, 9.178419661560148768 ) ) ;
#20862=CARTESIAN_POINT ( 'NONE',  ( 23.79193388295309219, 28.98609808355011452, -9.422646554964176246 ) ) ;
#20864=CARTESIAN_POINT ( 'NONE',  ( 0.5672860446885946706, 37.53182223685058716, -6.568693074176339408 ) ) ;
#20869=CARTESIAN_POINT ( 'NONE',  ( -36.28567981536816234, -9.465698090293395595, -9.422646554964174470 ) ) ;
#20870=CARTESIAN_POINT ( 'NONE',  ( -29.61572577327014955, -16.11461842845715253, 8.807470649214879543 ) ) ;
#20871=EDGE_CURVE ( 'NONE', #13001, #42210, #21697, .T. ) ;
#20885=CARTESIAN_POINT ( 'NONE',  ( -31.93002621080269421, -9.285431160462335853, -2.408242355805840784 ) ) ;
#20890=CARTESIAN_POINT ( 'NONE',  ( 13.92102703536701114, 30.85732372859822803, 8.356839323120299312 ) ) ;
#20893=EDGE_CURVE ( 'NONE', #47273, #18535, #27802, .T. ) ;
#20904=ADVANCED_FACE ( 'NONE', ( #20532 ), #289, .T. ) ;
#20906=EDGE_CURVE ( 'NONE', #28949, #13072, #10184, .T. ) ;
#20912=CARTESIAN_POINT ( 'NONE',  ( 2.462075149652696027, -16.57295996686994499, 9.403735324607438884 ) ) ;
#20916=B_SPLINE_CURVE_WITH_KNOTS ( 'NONE', 3,
 ( #38332, #18791, #50568, #23159 ),
 .UNSPECIFIED., .F., .F.,
 ( 4, 4 ),
 ( 0.000000000000000000, 0.001246897409371945480 ),
 .UNSPECIFIED. ) ;
#20924=CARTESIAN_POINT ( 'NONE',  ( -1.780619886013952602, -1.041246721325602920, 9.886433018048069954 ) ) ;
#20926=EDGE_CURVE ( 'NONE', #13001, #27141, #38160, .T. ) ;
#20927=CARTESIAN_POINT ( 'NONE',  ( 34.38425513258721367, -36.82177522737820397, 8.807470649214879543 ) ) ;
#20929=CARTESIAN_POINT ( 'NONE',  ( -48.99656738986512039, 11.00747004110376182, 1.847720168420772691 ) ) ;
#20931=CARTESIAN_POINT ( 'NONE',  ( 15.62858259096121216, -5.755205073598614440, -9.683996418299976483 ) ) ;
#20933=CARTESIAN_POINT ( 'NONE',  ( -36.02002318912981593, 10.56068015588366116, -3.721387749823083624 ) ) ;
#20943=CARTESIAN_POINT ( 'NONE',  ( -6.508636631827791064, -15.75743548351446854, 8.953103998512858652 ) ) ;
#20949=CARTESIAN_POINT ( 'NONE',  ( 25.61277432017878297, -22.36370378792834757, 7.906207997025717304 ) ) ;
#20952=CARTESIAN_POINT ( 'NONE',  ( -1.565927753002675615, 1.491090762200759423, 9.882710035074767418 ) ) ;
#20957=CARTESIAN_POINT ( 'NONE',  ( 1.224837355096363156, 1.100071488488148619, 9.927568724237747944 ) ) ;
#20968=CARTESIAN_POINT ( 'NONE',  ( 0.5359691244547075684, -1.100286284792932889, 9.966990753365129407 ) ) ;
#20979=EDGE_LOOP ( 'NONE', ( #4363, #21459, #37154, #34652 ) ) ;
#20981=CARTESIAN_POINT ( 'NONE',  ( 24.39427009665985224, 44.07992421011656603, 8.807470649214879543 ) ) ;
#20982=EDGE_CURVE ( 'NONE', #6876, #6581, #24697, .T. ) ;
#20991=CARTESIAN_POINT ( 'NONE',  ( 15.80799809827373004, -29.65358618225706522, -8.016098858316199838 ) ) ;
#21003=ORIENTED_EDGE ( 'NONE', *, *, #18964, .F. ) ;
#21009=B_SPLINE_CURVE_WITH_KNOTS ( 'NONE', 3,
 ( #20927, #28879, #21417, #9376 ),
 .UNSPECIFIED., .F., .F.,
 ( 4, 4 ),
 ( 0.000000000000000000, 0.2562577668812813236 ),
 .UNSPECIFIED. ) ;
#21010=CARTESIAN_POINT ( 'NONE',  ( -22.18397680750705092, -25.02304503454527662, -8.917361510505369182 ) ) ;
#21011=CARTESIAN_POINT ( 'NONE',  ( 27.33593271309472073, -41.94268121623323253, -9.367992836599951190 ) ) ;
#21035=ORIENTED_EDGE ( 'NONE', *, *, #21829, .T. ) ;
#21042=CARTESIAN_POINT ( 'NONE',  ( 0.1291293981302941152, 10.01396644373391887, 3.215203646305365925 ) ) ;
#21047=CARTESIAN_POINT ( 'NONE',  ( -17.34922095635781147, -33.24536858281880569, 8.914903342594564961 ) ) ;
#21053=CARTESIAN_POINT ( 'NONE',  ( -45.64490844644706868, -21.32281559348764333, 8.807470649214879543 ) ) ;
#21059=CARTESIAN_POINT ( 'NONE',  ( 0.1265591857323814795, 1.213367045380162823, 9.963925895596176474 ) ) ;
#21064=CARTESIAN_POINT ( 'NONE',  ( 24.47767542868285062, -23.18653802921781448, 8.807470649214879543 ) ) ;
#21067=CARTESIAN_POINT ( 'NONE',  ( -8.864235763825252690, -4.693841405978048442, 9.516222621873129839 ) ) ;
#21068=B_SPLINE_CURVE_WITH_KNOTS ( 'NONE', 3,
 ( #43875, #42856, #47186, #27482 ),
 .UNSPECIFIED., .F., .F.,
 ( 4, 4 ),
 ( 4.114257970988321555E-18, 0.0004072981213154478700 ),
 .UNSPECIFIED. ) ;
#21073=CARTESIAN_POINT ( 'NONE',  ( 0.7603004677395120980, -1.297166976433627550, 9.936141075690075652 ) ) ;
#21074=CARTESIAN_POINT ( 'NONE',  ( 50.11058929355270664, -7.578863168071591438, 7.455576670931136185 ) ) ;
#21081=ORIENTED_EDGE ( 'NONE', *, *, #22075, .T. ) ;
#21084=EDGE_LOOP ( 'NONE', ( #23155, #13661, #41346 ) ) ;
#21088=B_SPLINE_SURFACE_WITH_KNOTS ( 'NONE', 3, 3, ( 
 ( #21288, #48937, #37472, #13823 ),
 ( #41292, #6394, #44859, #1797 ),
 ( #37715, #17443, #33115, #40794 ),
 ( #18185, #41047, #5887, #22042 ) ),
 .UNSPECIFIED., .F., .F., .F.,
 ( 4, 4 ),
 ( 4, 4 ),
 ( 0.000000000000000000, 1.000000000000000000 ),
 ( 0.000000000000000000, 1.000000000000000000 ),
 .UNSPECIFIED. ) ;
#21098=B_SPLINE_CURVE_WITH_KNOTS ( 'NONE', 3,
 ( #28443, #32298, #1989, #45057 ),
 .UNSPECIFIED., .F., .F.,
 ( 4, 4 ),
 ( 0.000000000000000000, 0.002466147708923232748 ),
 .UNSPECIFIED. ) ;
#21103=CARTESIAN_POINT ( 'NONE',  ( -8.277096487746778308, 33.14818118907697198, 7.455576670931136185 ) ) ;
#21109=CARTESIAN_POINT ( 'NONE',  ( 1.448406091252584238, -0.9360325558322883932, 9.928159647716132241 ) ) ;
#21115=ORIENTED_EDGE ( 'NONE', *, *, #36055, .F. ) ;
#21118=CARTESIAN_POINT ( 'NONE',  ( -30.77287599203642188, -12.70002479445974686, 3.199614146704519602 ) ) ;
#21130=EDGE_CURVE ( 'NONE', #22165, #15558, #2061, .T. ) ;
#21132=VERTEX_POINT ( 'NONE', #38409 ) ;
#21133=CARTESIAN_POINT ( 'NONE',  ( 5.888214538810389698, 16.20866436362417673, 8.727788335465566760 ) ) ;
#21134=FACE_OUTER_BOUND ( 'NONE', #49456, .T. ) ;
#21141=CARTESIAN_POINT ( 'NONE',  ( 44.99506233596247995, 23.32283626942318833, 7.455576670931136185 ) ) ;
#21150=CARTESIAN_POINT ( 'NONE',  ( -1.721971274562257515, -0.09408549481333014497, 9.928159647716187308 ) ) ;
#21155=ADVANCED_FACE ( 'NONE', ( #661 ), #40045, .T. ) ;
#21165=CARTESIAN_POINT ( 'NONE',  ( -46.55190821232856280, 18.53135734581249139, -8.917361510505369182 ) ) ;
#21166=ORIENTED_EDGE ( 'NONE', *, *, #34413, .F. ) ;
#21167=CARTESIAN_POINT ( 'NONE',  ( -0.4166666666666669072, 0.000000000000000000, 10.00000000000000000 ) ) ;
#21168=CARTESIAN_POINT ( 'NONE',  ( 9.696760411815720460, 2.443938934556958653, 0.000000000000000000 ) ) ;
#21177=CARTESIAN_POINT ( 'NONE',  ( 22.93339884797969930, -29.71580813607141636, -3.721387749823079627 ) ) ;
#21179=ADVANCED_FACE ( 'NONE', ( #20397 ), #16267, .T. ) ;
#21183=CARTESIAN_POINT ( 'NONE',  ( 6.174150299305392053, -50.00000000000000711, 8.807470649214879543 ) ) ;
#21185=EDGE_CURVE ( 'NONE', #18535, #2268, #14865, .T. ) ;
#21191=CARTESIAN_POINT ( 'NONE',  ( -47.87295225382221275, -14.46560184742400423, -2.408242355805840784 ) ) ;
#21197=B_SPLINE_SURFACE_WITH_KNOTS ( 'NONE', 3, 3, ( 
 ( #19507, #39287, #549, #23882 ),
 ( #35195, #8493, #11832, #27483 ),
 ( #42602, #24148, #3869, #20282 ),
 ( #19255, #4133, #26965, #19772 ) ),
 .UNSPECIFIED., .F., .F., .F.,
 ( 4, 4 ),
 ( 4, 4 ),
 ( 0.000000000000000000, 1.000000000000000000 ),
 ( 0.000000000000000000, 1.000000000000000000 ),
 .UNSPECIFIED. ) ;
#21199=CARTESIAN_POINT ( 'NONE',  ( 1.780432407520001536, 1.041450996408479046, 9.894754715216729224 ) ) ;
#21208=CARTESIAN_POINT ( 'NONE',  ( -1.655083081098053466, 7.799304653815004151, 2.264627287779097387E-14 ) ) ;
#21231=CARTESIAN_POINT ( 'NONE',  ( 40.86389006639091548, 8.513139889764598678, -8.080361901872240793 ) ) ;
#21236=CARTESIAN_POINT ( 'NONE',  ( 0.3862712429686978033, -1.188820645368937834, -10.00000000000000000 ) ) ;
#21240=CARTESIAN_POINT ( 'NONE',  ( 1.011271242968683648, 0.7347315653655930312, -3.333333333333333481 ) ) ;
#21256=CARTESIAN_POINT ( 'NONE',  ( 47.88254548617766204, -14.43607691413525984, -3.760136334089591248 ) ) ;
#21267=CARTESIAN_POINT ( 'NONE',  ( -1.011271242968688533, 0.7347315653655859258, 10.00000000000000000 ) ) ;
#21269=CARTESIAN_POINT ( 'NONE',  ( 14.52758583651987223, 8.922352469211173087, 8.953103998512858652 ) ) ;
#21272=CARTESIAN_POINT ( 'NONE',  ( 0.3862712429686894766, -1.188820645368940276, 10.00000000000000000 ) ) ;
#21273=VERTEX_POINT ( 'NONE', #13460 ) ;
#21288=CARTESIAN_POINT ( 'NONE',  ( 4.641001526964560142, 50.00000000000000711, -8.016098858316199838 ) ) ;
#21302=CARTESIAN_POINT ( 'NONE',  ( 1.290940757014967355, -0.08848829412275825701, 9.947020512645421420 ) ) ;
#21303=CARTESIAN_POINT ( 'NONE',  ( -33.43156050989129824, 4.370686678976795747, 8.807470649214879543 ) ) ;
#21306=CARTESIAN_POINT ( 'NONE',  ( -44.99506233596264337, -23.32283626942287214, 7.455576670931136185 ) ) ;
#21314=ORIENTED_EDGE ( 'NONE', *, *, #37138, .T. ) ;
#21315=CARTESIAN_POINT ( 'NONE',  ( 1.011271242968677653, 0.7347315653656002477, 10.00000000000000000 ) ) ;
#21322=ORIENTED_EDGE ( 'NONE', *, *, #45119, .T. ) ;
#21332=CARTESIAN_POINT ( 'NONE',  ( 16.02661358026014327, 4.530191650547718218, -9.683996418299976483 ) ) ;
#21337=CARTESIAN_POINT ( 'NONE',  ( 0.1425549192113746144, -1.238581250503543618, 9.981352469109934233 ) ) ;
#21342=CARTESIAN_POINT ( 'NONE',  ( 8.277096487746778308, -33.14818118907697198, 7.455576670931136185 ) ) ;
#21344=CARTESIAN_POINT ( 'NONE',  ( -31.28977333267361871, 11.25592690310926969, -2.408242355805840784 ) ) ;
#21348=ORIENTED_EDGE ( 'NONE', *, *, #19327, .F. ) ;
#21353=CARTESIAN_POINT ( 'NONE',  ( 2.538055338523177440, 33.28424297489108596, -9.367992836599954742 ) ) ;
#21356=VERTEX_POINT ( 'NONE', #30384 ) ;
#21372=ORIENTED_EDGE ( 'NONE', *, *, #29595, .T. ) ;
#21373=EDGE_CURVE ( 'NONE', #36910, #12217, #34513, .T. ) ;
#21381=CARTESIAN_POINT ( 'NONE',  ( 10.69268279052430159, 12.77266927778462779, -2.870787844569587133 ) ) ;
#21417=CARTESIAN_POINT ( 'NONE',  ( 29.12062022658201244, -29.99172060348948321, 8.846626183609803462 ) ) ;
#21427=B_SPLINE_CURVE_WITH_KNOTS ( 'NONE', 3,
 ( #3591, #31323, #15914, #22839 ),
 .UNSPECIFIED., .F., .F.,
 ( 4, 4 ),
 ( 5.210275057513392971E-05, 0.0002352737929598119979 ),
 .UNSPECIFIED. ) ;
#21429=EDGE_CURVE ( 'NONE', #5197, #44630, #47278, .T. ) ;
#21430=CYLINDRICAL_SURFACE ( 'NONE', #15581, 10.00000000000000000 ) ;
#21434=ORIENTED_EDGE ( 'NONE', *, *, #6406, .T. ) ;
#21447=CARTESIAN_POINT ( 'NONE',  ( -13.59579750444763668, 10.60877755095910935, 8.727788335465566760 ) ) ;
#21451=ORIENTED_EDGE ( 'NONE', *, *, #20893, .T. ) ;
#21459=ORIENTED_EDGE ( 'NONE', *, *, #39950, .T. ) ;
#21485=CARTESIAN_POINT ( 'NONE',  ( 16.69947034530964913, -2.312583065866261389, 2.590526750877053086 ) ) ;
#21493=CARTESIAN_POINT ( 'NONE',  ( -29.18392875402943432, -17.44843138996582965, 7.906207997025717304 ) ) ;
#21505=B_SPLINE_SURFACE_WITH_KNOTS ( 'NONE', 3, 3, ( 
 ( #3244, #14806, #42501, #19669 ),
 ( #30202, #22758, #18643, #46574 ),
 ( #15063, #30726, #34315, #45813 ),
 ( #38185, #30461, #7889, #3494 ) ),
 .UNSPECIFIED., .F., .F., .F.,
 ( 4, 4 ),
 ( 4, 4 ),
 ( 0.000000000000000000, 1.000000000000000000 ),
 ( 0.000000000000000000, 1.000000000000000000 ),
 .UNSPECIFIED. ) ;
#21514=VERTEX_POINT ( 'NONE', #33671 ) ;
#21530=ORIENTED_EDGE ( 'NONE', *, *, #19620, .F. ) ;
#21539=CARTESIAN_POINT ( 'NONE',  ( 0.000000000000000000, 0.000000000000000000, 10.00000000000000000 ) ) ;
#21545=CARTESIAN_POINT ( 'NONE',  ( -14.29087950072019098, -9.652079258044555132, 8.727788335465566760 ) ) ;
#21546=ADVANCED_BREP_SHAPE_REPRESENTATION ( '', ( #5361, #45486 ), #38147 ) ;
#21550=CARTESIAN_POINT ( 'NONE',  ( 18.69789054174343690, -27.49790346457731616, -2.408242355805840784 ) ) ;
#21551=CARTESIAN_POINT ( 'NONE',  ( -9.260964247899874380, 13.84230907185616744, -9.683996418299976483 ) ) ;
#21552=CARTESIAN_POINT ( 'NONE',  ( -48.34672127938071640, 13.00749071703899773, 3.199614146704519602 ) ) ;
#21560=DIRECTION ( 'NONE',  ( -1.000000000000000000, 0.000000000000000000, 0.000000000000000000 ) ) ;
#21562=DIRECTION ( 'NONE',  ( 0.000000000000000000, 0.000000000000000000, -1.000000000000000000 ) ) ;
#21564=ORIENTED_EDGE ( 'NONE', *, *, #20871, .T. ) ;
#21570=ADVANCED_FACE ( 'NONE', ( #40614 ), #38782, .T. ) ;
#21578=CARTESIAN_POINT ( 'NONE',  ( 14.86945752723346637, 7.944783388879009145, 2.590526750877053086 ) ) ;
#21585=CARTESIAN_POINT ( 'NONE',  ( -20.20970188815926250, -31.63128376650800533, 3.209567239418976481 ) ) ;
#21602=CARTESIAN_POINT ( 'NONE',  ( -4.207128120815918256E-14, 3.058192377181588826E-14, 10.00000000000000000 ) ) ;
#21607=CARTESIAN_POINT ( 'NONE',  ( -4.672045878990125800, 33.19353511768168374, 1.847720168420772691 ) ) ;
#21620=DIRECTION ( 'NONE',  ( 0.5877852522924685852, 0.8090169943749507819, 0.000000000000000000 ) ) ;
#21621=B_SPLINE_SURFACE_WITH_KNOTS ( 'NONE', 3, 3, ( 
 ( #13776, #33311, #29440, #9938 ),
 ( #18134, #25595, #2240, #21736 ),
 ( #33557, #49145, #2989, #34306 ),
 ( #37664, #42493, #27633, #43260 ) ),
 .UNSPECIFIED., .F., .F., .F.,
 ( 4, 4 ),
 ( 4, 4 ),
 ( 0.000000000000000000, 1.000000000000000000 ),
 ( 0.000000000000000000, 1.000000000000000000 ),
 .UNSPECIFIED. ) ;
#21628=ORIENTED_EDGE ( 'NONE', *, *, #16510, .T. ) ;
#21631=CARTESIAN_POINT ( 'NONE',  ( 0.7849184246612691540, -1.242376769536456704, 9.958264684458541183 ) ) ;
#21632=B_SPLINE_CURVE_WITH_KNOTS ( 'NONE', 3,
 ( #6921, #26412, #46394, #15122 ),
 .UNSPECIFIED., .F., .F.,
 ( 4, 4 ),
 ( 1.105609816134553033E-15, 0.0004154657329505368596 ),
 .UNSPECIFIED. ) ;
#21633=CARTESIAN_POINT ( 'NONE',  ( 26.76882631152636094, -42.35470813487675201, -8.917361510505369182 ) ) ;
#21635=FACE_OUTER_BOUND ( 'NONE', #25302, .T. ) ;
#21640=CARTESIAN_POINT ( 'NONE',  ( -8.032723559237163968, 41.13077784380362090, 7.544061037322996377 ) ) ;
#21646=FACE_OUTER_BOUND ( 'NONE', #45195, .T. ) ;
#21661=ORIENTED_EDGE ( 'NONE', *, *, #15300, .F. ) ;
#21665=ORIENTED_EDGE ( 'NONE', *, *, #10053, .F. ) ;
#21682=CARTESIAN_POINT ( 'NONE',  ( 0.2458784654125734381, 0.3384226744270686926, 9.992713367193012175 ) ) ;
#21687=ADVANCED_FACE ( 'NONE', ( #11585 ), #42436, .T. ) ;
#21691=CARTESIAN_POINT ( 'NONE',  ( -15.57957361750255565, -5.755602074545403291, 3.266473740018926541 ) ) ;
#21692=APPLICATION_CONTEXT ( 'automotive_design' ) ;
#21697=B_SPLINE_CURVE_WITH_KNOTS ( 'NONE', 3,
 ( #4382, #27979, #37, #15932 ),
 .UNSPECIFIED., .F., .F.,
 ( 4, 4 ),
 ( 0.000000000000000000, 0.2545280377015987638 ),
 .UNSPECIFIED. ) ;
#21698=ORIENTED_EDGE ( 'NONE', *, *, #6484, .F. ) ;
#21708=ORIENTED_EDGE ( 'NONE', *, *, #24647, .T. ) ;
#21712=CARTESIAN_POINT ( 'NONE',  ( 33.43156050989131955, -4.370686678976570150, 8.807470649214879543 ) ) ;
#21717=CARTESIAN_POINT ( 'NONE',  ( 23.82716369509147825, 44.49195112876006419, 8.356839323120299312 ) ) ;
#21718=VERTEX_POINT ( 'NONE', #3359 ) ;
#21719=ORIENTED_EDGE ( 'NONE', *, *, #11882, .T. ) ;
#21723=CARTESIAN_POINT ( 'NONE',  ( 1.238491169207262432, 5.772936915101642086, 9.586754400233969520 ) ) ;
#21728=EDGE_CURVE ( 'NONE', #43044, #37083, #19121, .T. ) ;
#21736=CARTESIAN_POINT ( 'NONE',  ( 1.011271242968694084, -0.7347315653655782652, -3.333333333333333481 ) ) ;
#21742=CARTESIAN_POINT ( 'NONE',  ( -33.16902712922616558, 37.70469005304312304, 1.847720168420772691 ) ) ;
#21745=CARTESIAN_POINT ( 'NONE',  ( -18.69789054174323084, 27.49790346457746182, -2.408242355805840784 ) ) ;
#21748=CARTESIAN_POINT ( 'NONE',  ( 0.3862712429686894766, -1.188820645368940276, 10.00000000000000000 ) ) ;
#21752=AXIS2_PLACEMENT_3D ( 'NONE', #30647, #38097, #31156 ) ;
#21754=ADVANCED_FACE ( 'NONE', ( #7998 ), #24057, .T. ) ;
#21761=EDGE_CURVE ( 'NONE', #39341, #27105, #30002, .T. ) ;
#21776=CARTESIAN_POINT ( 'NONE',  ( 4.339432828817248122, 37.24807810779213213, -8.192531242611266862 ) ) ;
#21784=EDGE_CURVE ( 'NONE', #18218, #16294, #11531, .T. ) ;
#21786=EDGE_CURVE ( 'NONE', #37517, #14294, #16434, .T. ) ;
#21792=ORIENTED_EDGE ( 'NONE', *, *, #40853, .F. ) ;
#21795=CARTESIAN_POINT ( 'NONE',  ( 12.78770032058947237, 31.68259716188277864, 7.455576670931136185 ) ) ;
#21796=EDGE_LOOP ( 'NONE', ( #42577, #48095, #44096, #26816 ) ) ;
#21800=FACE_OUTER_BOUND ( 'NONE', #19442, .T. ) ;
#21802=CARTESIAN_POINT ( 'NONE',  ( -5.320787806781440921, 8.466948512633457824, -1.544988095791843818E-15 ) ) ;
#21805=CARTESIAN_POINT ( 'NONE',  ( -0.7658683902953777878, 0.9641952520609238242, 9.975326647350893694 ) ) ;
#21806=CARTESIAN_POINT ( 'NONE',  ( -47.22310614333779455, -16.46562252335923660, -3.760136334089591248 ) ) ;
#21808=ORIENTED_EDGE ( 'NONE', *, *, #46852, .F. ) ;
#21814=EDGE_CURVE ( 'NONE', #17812, #21132, #23144, .T. ) ;
#21823=CARTESIAN_POINT ( 'NONE',  ( 0.03684434657438797472, 1.221810944802236287, 9.969517326150310055 ) ) ;
#21829=EDGE_CURVE ( 'NONE', #9096, #18355, #7251, .T. ) ;
#21832=VECTOR ( 'NONE', #20232, 1000.000000000000227 ) ;
#21840=B_SPLINE_CURVE_WITH_KNOTS ( 'NONE', 3,
 ( #25334, #33801, #41737, #37657 ),
 .UNSPECIFIED., .F., .F.,
 ( 4, 4 ),
 ( 0.000000000000000000, 0.2562577668812811571 ),
 .UNSPECIFIED. ) ;
#21844=CARTESIAN_POINT ( 'NONE',  ( -1.436574951976946402, 1.361596091069438463, 9.897807938190497978 ) ) ;
#21865=CARTESIAN_POINT ( 'NONE',  ( -16.52264463346130796, 2.779753662172870232, 9.403735324607438884 ) ) ;
#21874=CARTESIAN_POINT ( 'NONE',  ( -2.961022939495062900, 16.59676755884084187, 2.590526750877053086 ) ) ;
#21881=CARTESIAN_POINT ( 'NONE',  ( -0.3370904143228963812, 0.2449105217885287067, 10.00000000000000000 ) ) ;
#21886=CARTESIAN_POINT ( 'NONE',  ( -2.491056982571220324, 9.716321351877633461, 9.390253821402618328 ) ) ;
#21890=CARTESIAN_POINT ( 'NONE',  ( 16.99749102614301677, -1.320765928724307425, 8.953103998512858652 ) ) ;
#21893=VERTEX_POINT ( 'NONE', #28993 ) ;
#21897=B_SPLINE_CURVE_WITH_KNOTS ( 'NONE', 3,
 ( #41453, #38378, #37385, #41191 ),
 .UNSPECIFIED., .F., .F.,
 ( 4, 4 ),
 ( 0.9688112071879398934, 0.9724175925769218409 ),
 .UNSPECIFIED. ) ;
#21903=ORIENTED_EDGE ( 'NONE', *, *, #2346, .T. ) ;
#21906=DIRECTION ( 'NONE',  ( 0.000000000000000000, 0.000000000000000000, -1.000000000000000000 ) ) ;
#21910=CARTESIAN_POINT ( 'NONE',  ( -33.14391172085785797, -37.72293746533094350, -8.016098858316205167 ) ) ;
#21913=ORIENTED_EDGE ( 'NONE', *, *, #14351, .F. ) ;
#21914=CARTESIAN_POINT ( 'NONE',  ( 0.8965959638259385356, 1.582931917743541028, 9.903764339332076005 ) ) ;
#21930=EDGE_CURVE ( 'NONE', #29168, #16294, #7167, .T. ) ;
#21947=CARTESIAN_POINT ( 'NONE',  ( 0.3862712429686978033, -1.188820645368937834, -3.333333333333333481 ) ) ;
#21948=ADVANCED_FACE ( 'NONE', ( #31031 ), #15001, .T. ) ;
#21951=CARTESIAN_POINT ( 'NONE',  ( 0.2778388845795309314, -1.251314014313100520, 9.976582533991681601 ) ) ;
#21952=CARTESIAN_POINT ( 'NONE',  ( -46.10908423965022251, -19.89422939639105437, 1.847720168420772691 ) ) ;
#21957=ORIENTED_EDGE ( 'NONE', *, *, #18001, .T. ) ;
#21963=CARTESIAN_POINT ( 'NONE',  ( -1.011271242968683426, -0.7347315653655928092, 10.00000000000000000 ) ) ;
#21970=CARTESIAN_POINT ( 'NONE',  ( -1.543575080196365468, 5.756315878809935782, -4.878909776184769953E-16 ) ) ;
#21972=ORIENTED_EDGE ( 'NONE', *, *, #36167, .T. ) ;
#21990=CARTESIAN_POINT ( 'NONE',  ( -47.55282581475773185, 15.45084971874723934, 0.000000000000000000 ) ) ;
#21994=B_SPLINE_CURVE_WITH_KNOTS ( 'NONE', 3,
 ( #25921, #37486, #14096, #45124 ),
 .UNSPECIFIED., .F., .F.,
 ( 4, 4 ),
 ( 0.8097120833243680593, 0.9322955464062552267 ),
 .UNSPECIFIED. ) ;
#21996=CARTESIAN_POINT ( 'NONE',  ( 34.08355720199905647, -2.371364769369109116, 7.455576670931136185 ) ) ;
#22004=ORIENTED_EDGE ( 'NONE', *, *, #49465, .F. ) ;
#22017=CARTESIAN_POINT ( 'NONE',  ( -31.94178169330213279, 9.256608784834037706, -3.760136334089591248 ) ) ;
#22023=ORIENTED_EDGE ( 'NONE', *, *, #29379, .F. ) ;
#22024=EDGE_CURVE ( 'NONE', #19380, #14899, #2337, .T. ) ;
#22037=B_SPLINE_SURFACE_WITH_KNOTS ( 'NONE', 3, 3, ( 
 ( #6782, #14479, #46249, #22428 ),
 ( #18569, #11148, #26537, #34245 ),
 ( #49824, #14733, #26794, #42176 ),
 ( #7044, #38355, #18819, #34501 ) ),
 .UNSPECIFIED., .F., .F., .F.,
 ( 4, 4 ),
 ( 4, 4 ),
 ( 0.000000000000000000, 1.000000000000000000 ),
 ( 0.000000000000000000, 1.000000000000000000 ),
 .UNSPECIFIED. ) ;
#22040=EDGE_CURVE ( 'NONE', #10853, #33462, #44730, .T. ) ;
#22042=CARTESIAN_POINT ( 'NONE',  ( 1.250000000000000222, 0.000000000000000000, 10.00000000000000000 ) ) ;
#22045=CYLINDRICAL_SURFACE ( 'NONE', #36678, 10.00000000000000000 ) ;
#22055=CARTESIAN_POINT ( 'NONE',  ( -14.29087950072019098, -9.652079258044555132, 8.727788335465566760 ) ) ;
#22061=CARTESIAN_POINT ( 'NONE',  ( -0.3370904143228978245, 0.2449105217885259589, 10.00000000000000000 ) ) ;
#22070=EDGE_CURVE ( 'NONE', #15558, #30326, #13961, .T. ) ;
#22075=EDGE_CURVE ( 'NONE', #46476, #22371, #11776, .T. ) ;
#22077=B_SPLINE_CURVE_WITH_KNOTS ( 'NONE', 3,
 ( #26467, #22618, #50015, #49516 ),
 .UNSPECIFIED., .F., .F.,
 ( 4, 4 ),
 ( 2.557173108762071179E-16, 0.0001831559689937848462 ),
 .UNSPECIFIED. ) ;
#22085=CARTESIAN_POINT ( 'NONE',  ( -25.04522487443065160, 22.77512090857326754, 8.356839323120299312 ) ) ;
#22087=CARTESIAN_POINT ( 'NONE',  ( -4.256388337216303164, 5.377297509087435756, 9.753789706659947711 ) ) ;
#22089=ORIENTED_EDGE ( 'NONE', *, *, #19134, .T. ) ;
#22094=VERTEX_POINT ( 'NONE', #239 ) ;
#22097=ORIENTED_EDGE ( 'NONE', *, *, #39950, .F. ) ;
#22104=FACE_BOUND ( 'NONE', #37640, .T. ) ;
#22105=CARTESIAN_POINT ( 'NONE',  ( 1.468713901642212161, 0.3220470327672588229, 9.927319414211225990 ) ) ;
#22106=CARTESIAN_POINT ( 'NONE',  ( -11.73320209285699889, 11.96063479729179768, 9.403735324607438884 ) ) ;
#22111=VERTEX_POINT ( 'NONE', #1497 ) ;
#22123=CARTESIAN_POINT ( 'NONE',  ( -24.39427009666018265, -44.07992421011638129, 8.807470649214879543 ) ) ;
#22137=ORIENTED_EDGE ( 'NONE', *, *, #37894, .T. ) ;
#22148=CARTESIAN_POINT ( 'NONE',  ( 15.62858259096121216, -5.755205073598612664, -9.683996418299976483 ) ) ;
#22151=CARTESIAN_POINT ( 'NONE',  ( -1.637520033018239118, -0.1700351954323520154, 9.927568724237804787 ) ) ;
#22160=CARTESIAN_POINT ( 'NONE',  ( -0.2774838294623820922, 1.251476322270256736, 9.957892297621016908 ) ) ;
#22165=VERTEX_POINT ( 'NONE', #13528 ) ;
#22171=ADVANCED_FACE ( 'NONE', ( #40494 ), #8490, .T. ) ;
#22174=CARTESIAN_POINT ( 'NONE',  ( -1.104609456715841986, -0.6504863887005195577, 9.948547179989617462 ) ) ;
#22196=B_SPLINE_CURVE_WITH_KNOTS ( 'NONE', 3,
 ( #44185, #39870, #43939, #44430 ),
 .UNSPECIFIED., .F., .F.,
 ( 4, 4 ),
 ( 0.000000000000000000, 0.2545280377015988749 ),
 .UNSPECIFIED. ) ;
#22198=CARTESIAN_POINT ( 'NONE',  ( 0.3862712429686810944, 1.188820645368943607, -3.333333333333333481 ) ) ;
#22204=CIRCLE ( 'NONE', #10728, 10.00000000000000000 ) ;
#22206=CARTESIAN_POINT ( 'NONE',  ( 0.3370904143228981575, -0.2449105217885261532, -10.00000000000000000 ) ) ;
#22208=CARTESIAN_POINT ( 'NONE',  ( -0.3862712429686895876, 1.188820645368940720, 10.00000000000000000 ) ) ;
#22209=CARTESIAN_POINT ( 'NONE',  ( -7.359817328027146388, -15.16751262232800102, 2.590526750877053086 ) ) ;
#22210=CARTESIAN_POINT ( 'NONE',  ( 1.011271242968677653, 0.7347315653656002477, 10.00000000000000000 ) ) ;
#22224=CARTESIAN_POINT ( 'NONE',  ( 34.08355720199905647, -2.371364769369109116, 7.455576670931136185 ) ) ;
#22255=VERTEX_POINT ( 'NONE', #20862 ) ;
#22276=ORIENTED_EDGE ( 'NONE', *, *, #26962, .T. ) ;
#22278=CARTESIAN_POINT ( 'NONE',  ( -16.69947034530963847, 2.312583065866374632, 2.590526750877053086 ) ) ;
#22295=CARTESIAN_POINT ( 'NONE',  ( -8.277096487746778308, 50.00000000000000711, 7.455576670931136185 ) ) ;
#22313=CARTESIAN_POINT ( 'NONE',  ( 1.437255894074055185, -3.713052624461447682, -1.301042606982605321E-15 ) ) ;
#22347=B_SPLINE_SURFACE_WITH_KNOTS ( 'NONE', 3, 3, ( 
 ( #508, #39508, #46894, #39761 ),
 ( #24109, #4349, #47390, #19987 ),
 ( #16149, #32058, #19738, #11792 ),
 ( #8713, #43081, #27442, #19474 ) ),
 .UNSPECIFIED., .F., .F., .F.,
 ( 4, 4 ),
 ( 4, 4 ),
 ( 0.000000000000000000, 1.000000000000000000 ),
 ( 0.000000000000000000, 1.000000000000000000 ),
 .UNSPECIFIED. ) ;
#22350=CARTESIAN_POINT ( 'NONE',  ( 11.73320209285708415, -11.96063479729170886, 9.403735324607438884 ) ) ;
#22361=ORIENTED_EDGE ( 'NONE', *, *, #32411, .T. ) ;
#22365=CARTESIAN_POINT ( 'NONE',  ( 2.322372356066598531, 2.286285436021770145, 9.799352050262459812 ) ) ;
#22366=CARTESIAN_POINT ( 'NONE',  ( -12.78770032058971395, -31.68259716188267916, 7.455576670931136185 ) ) ;
#22371=VERTEX_POINT ( 'NONE', #36289 ) ;
#22376=CARTESIAN_POINT ( 'NONE',  ( -1.228394325311288560, 1.341866297401936636, 9.903764339332077782 ) ) ;
#22382=EDGE_LOOP ( 'NONE', ( #2250, #15219, #6261, #31970, #46862 ) ) ;
#22386=CARTESIAN_POINT ( 'NONE',  ( 1.011271242968677653, 0.7347315653656002477, -10.00000000000000000 ) ) ;
#22400=CARTESIAN_POINT ( 'NONE',  ( -6.174150299305392053, 50.00000000000000000, 8.807470649214879543 ) ) ;
#22401=CARTESIAN_POINT ( 'NONE',  ( 0.4384698884932147211, 1.388183145050263745, 9.938560701278168708 ) ) ;
#22428=CARTESIAN_POINT ( 'NONE',  ( 1.011271242968683648, 0.7347315653655930312, 10.00000000000000000 ) ) ;
#22434=ORIENTED_EDGE ( 'NONE', *, *, #7955, .F. ) ;
#22443=EDGE_CURVE ( 'NONE', #29288, #15030, #5974, .T. ) ;
#22450=CARTESIAN_POINT ( 'NONE',  ( -0.3370904143228978245, 0.2449105217885259589, -10.00000000000000000 ) ) ;
#22455=CARTESIAN_POINT ( 'NONE',  ( 12.15085308559846844, -11.68662139125803989, 2.590526750877053086 ) ) ;
#22459=B_SPLINE_SURFACE_WITH_KNOTS ( 'NONE', 3, 3, ( 
 ( #10751, #30513, #15116, #18191 ),
 ( #33872, #14352, #6912, #49459 ),
 ( #50204, #46386, #30020, #14602 ),
 ( #34891, #26913, #7168, #42310 ) ),
 .UNSPECIFIED., .F., .F., .F.,
 ( 4, 4 ),
 ( 4, 4 ),
 ( 0.000000000000000000, 1.000000000000000000 ),
 ( 0.000000000000000000, 1.000000000000000000 ),
 .UNSPECIFIED. ) ;
#22469=CARTESIAN_POINT ( 'NONE',  ( -0.4166666666666664631, 0.000000000000000000, 10.00000000000000000 ) ) ;
#22472=EDGE_LOOP ( 'NONE', ( #44391, #21792, #12067, #48910, #16881 ) ) ;
#22475=CARTESIAN_POINT ( 'NONE',  ( 8.831420117243668599, 14.12636088103192655, -3.546734833711462365 ) ) ;
#22480=CARTESIAN_POINT ( 'NONE',  ( 1.540526284687965264, -1.371707213411490267, 9.886433018048071730 ) ) ;
#22484=CARTESIAN_POINT ( 'NONE',  ( 1.111507796622770883, 1.112188257001374581, 9.945241992664893615 ) ) ;
#22502=CARTESIAN_POINT ( 'NONE',  ( 7.576114424932982594, -33.14742743729794938, 7.906207997025717304 ) ) ;
#22505=ORIENTED_EDGE ( 'NONE', *, *, #38200, .F. ) ;
#22543=CARTESIAN_POINT ( 'NONE',  ( 30.67467450244491900, -28.55398182363552806, 7.544061037322998153 ) ) ;
#22544=ORIENTED_EDGE ( 'NONE', *, *, #4965, .F. ) ;
#22551=CARTESIAN_POINT ( 'NONE',  ( 28.55116071645549525, -41.05976639056858346, -2.408242355805840784 ) ) ;
#22552=CARTESIAN_POINT ( 'NONE',  ( 1.042245359060418375, 0.7067879234688301260, 9.974012008644017158 ) ) ;
#22555=ORIENTED_EDGE ( 'NONE', *, *, #25946, .T. ) ;
#22559=CARTESIAN_POINT ( 'NONE',  ( 31.46770792452135268, -38.94077080897339727, 3.199614146704519602 ) ) ;
#22569=EDGE_LOOP ( 'NONE', ( #4550, #9566, #32561, #32247 ) ) ;
#22573=CARTESIAN_POINT ( 'NONE',  ( -6.174150299305392053, 33.14591993373988998, 8.807470649214879543 ) ) ;
#22583=VERTEX_POINT ( 'NONE', #47699 ) ;
#22592=CARTESIAN_POINT ( 'NONE',  ( 5.297170062947166969, 5.958621178614006197, -4.472333961502705790E-16 ) ) ;
#22594=DIRECTION ( 'NONE',  ( 0.000000000000000000, 0.000000000000000000, -1.000000000000000000 ) ) ;
#22597=B_SPLINE_CURVE_WITH_KNOTS ( 'NONE', 3,
 ( #11571, #30822, #18734, #23103 ),
 .UNSPECIFIED., .F., .F.,
 ( 4, 4 ),
 ( 2.732001163471678047E-18, 0.009782300387714808892 ),
 .UNSPECIFIED. ) ;
#22604=CARTESIAN_POINT ( 'NONE',  ( -22.93339884797946127, 29.71580813607156912, -3.721387749823086732 ) ) ;
#22610=CARTESIAN_POINT ( 'NONE',  ( 36.08557433729230723, -35.58569447144768105, 7.455576670931136185 ) ) ;
#22615=CARTESIAN_POINT ( 'NONE',  ( 48.99656738986517723, -11.00747004110342431, 1.847720168420772691 ) ) ;
#22617=CARTESIAN_POINT ( 'NONE',  ( -36.08557433729205144, 35.58569447144795816, 7.455576670931136185 ) ) ;
#22618=CARTESIAN_POINT ( 'NONE',  ( -0.3904210042914396661, 2.126747006146315844, 9.882710035074776300 ) ) ;
#22622=( NAMED_UNIT ( * ) PLANE_ANGLE_UNIT ( ) SI_UNIT ( $, .RADIAN. ) );
#22633=CARTESIAN_POINT ( 'NONE',  ( -46.76852358249002606, 17.86468378716741512, -9.367992836599954742 ) ) ;
#22637=CARTESIAN_POINT ( 'NONE',  ( -24.39427009666018265, -44.07992421011638129, 8.807470649214879543 ) ) ;
#22646=CARTESIAN_POINT ( 'NONE',  ( 15.44803555374680393, 6.237487519713364570, -3.546734833711462365 ) ) ;
#22660=ORIENTED_EDGE ( 'NONE', *, *, #31789, .F. ) ;
#22664=ADVANCED_FACE ( 'NONE', ( #43631 ), #35532, .T. ) ;
#22684=CARTESIAN_POINT ( 'NONE',  ( -30.87089393895367095, 12.69923079256638587, -9.367992836599954742 ) ) ;
#22690=EDGE_CURVE ( 'NONE', #23786, #49960, #42676, .T. ) ;
#22691=CARTESIAN_POINT ( 'NONE',  ( 0.4266413953668419246, 1.250184266969606162, 9.943883492372851407 ) ) ;
#22694=B_SPLINE_CURVE_WITH_KNOTS ( 'NONE', 3,
 ( #48528, #13418, #2137, #40876 ),
 .UNSPECIFIED., .F., .F.,
 ( 4, 4 ),
 ( 0.01010185847678694501, 0.01012833122191989475 ),
 .UNSPECIFIED. ) ;
#22711=B_SPLINE_CURVE_WITH_KNOTS ( 'NONE', 3,
 ( #11464, #50417, #11715, #26607 ),
 .UNSPECIFIED., .F., .F.,
 ( 4, 4 ),
 ( 0.0006669682284780797596, 0.0007799402130920312336 ),
 .UNSPECIFIED. ) ;
#22718=CARTESIAN_POINT ( 'NONE',  ( 0.3862712429686815385, 1.188820645368943385, 9.972675548442461846 ) ) ;
#22722=B_SPLINE_CURVE_WITH_KNOTS ( 'NONE', 3,
 ( #38130, #10653, #15015, #30416 ),
 .UNSPECIFIED., .F., .F.,
 ( 4, 4 ),
 ( 3.969024117295675979E-17, 0.0004301978946275559026 ),
 .UNSPECIFIED. ) ;
#22726=CARTESIAN_POINT ( 'NONE',  ( -49.46074318306826001, 9.578883844007169301, 8.807470649214879543 ) ) ;
#22753=CARTESIAN_POINT ( 'NONE',  ( -1.019713130072858798, -3.848720492505054658, 6.098637220230962441E-17 ) ) ;
#22758=CARTESIAN_POINT ( 'NONE',  ( 23.29043492822826167, -24.10797434788167948, 1.847720168420772691 ) ) ;
#22767=CARTESIAN_POINT ( 'NONE',  ( 2.178343065408716139, 16.64136160116211727, -9.233365092205394475 ) ) ;
#22773=B_SPLINE_SURFACE_WITH_KNOTS ( 'NONE', 3, 3, ( 
 ( #188, #23258, #39444, #27377 ),
 ( #38679, #39193, #11984, #4025 ),
 ( #19421, #27638, #3771, #15826 ),
 ( #43270, #7890, #19670, #15574 ) ),
 .UNSPECIFIED., .F., .F., .F.,
 ( 4, 4 ),
 ( 4, 4 ),
 ( 0.000000000000000000, 1.000000000000000000 ),
 ( 0.000000000000000000, 1.000000000000000000 ),
 .UNSPECIFIED. ) ;
#22775=ORIENTED_EDGE ( 'NONE', *, *, #26594, .T. ) ;
#22779=CARTESIAN_POINT ( 'NONE',  ( -15.62858259096117841, 5.755205073598721910, -9.683996418299976483 ) ) ;
#22783=ORIENTED_EDGE ( 'NONE', *, *, #21784, .F. ) ;
#22789=B_SPLINE_CURVE_WITH_KNOTS ( 'NONE', 3,
 ( #43145, #39305, #43379, #19788 ),
 .UNSPECIFIED., .F., .F.,
 ( 4, 4 ),
 ( 0.7491799374948677759, 1.000000000000000000 ),
 .UNSPECIFIED. ) ;
#22794=ORIENTED_EDGE ( 'NONE', *, *, #12373, .F. ) ;
#22796=CARTESIAN_POINT ( 'NONE',  ( -1.011271242968693862, 0.7347315653655780432, 10.00000000000000000 ) ) ;
#22798=CARTESIAN_POINT ( 'NONE',  ( -1.066995270233474624, 33.23888904628638841, -3.760136334089591248 ) ) ;
#22803=CARTESIAN_POINT ( 'NONE',  ( -6.429410166934457216, -2.386389549874184279, 9.753789706659947711 ) ) ;
#22807=CARTESIAN_POINT ( 'NONE',  ( -1.011271242968677875, -0.7347315653656004697, 10.00000000000000000 ) ) ;
#22815=CARTESIAN_POINT ( 'NONE',  ( 9.174209336589868258, 3.979181203266223488, 9.646707543097347681 ) ) ;
#22816=CARTESIAN_POINT ( 'NONE',  ( -3.231548175622898089, 9.463461120997347820, 9.282506307616472441 ) ) ;
#22821=CARTESIAN_POINT ( 'NONE',  ( -0.3862712429686895876, 1.188820645368940720, 10.00000000000000000 ) ) ;
#22824=B_SPLINE_CURVE_WITH_KNOTS ( 'NONE', 3,
 ( #14169, #29843, #40881, #29586 ),
 .UNSPECIFIED., .F., .F.,
 ( 4, 4 ),
 ( 1.735570302229820823E-18, 2.647279941212161278E-05 ),
 .UNSPECIFIED. ) ;
#22828=CARTESIAN_POINT ( 'NONE',  ( 0.1469336902871260508, 1.496274467947966258, 9.953784399990622589 ) ) ;
#22830=CARTESIAN_POINT ( 'NONE',  ( 0.4266413953668419246, 1.250184266969606162, 9.943883492372851407 ) ) ;
#22834=ORIENTED_EDGE ( 'NONE', *, *, #6572, .F. ) ;
#22836=LINE ( 'NONE', #18219, #19636 ) ;
#22839=CARTESIAN_POINT ( 'NONE',  ( 0.9870575514054733546, 1.980598328282569653, 9.881002359080278907 ) ) ;
#22844=CARTESIAN_POINT ( 'NONE',  ( -2.948105490345101387, -9.555557232197246620, 9.282506307616472441 ) ) ;
#22849=CARTESIAN_POINT ( 'NONE',  ( -20.21530556545279111, 31.58467066308232063, -9.422646554964174470 ) ) ;
#22862=CARTESIAN_POINT ( 'NONE',  ( -1.377509002708424468, 0.6027468487255034368, 9.927319414211229542 ) ) ;
#22867=CARTESIAN_POINT ( 'NONE',  ( 10.70590866674922204, -12.76446523155706814, -3.546734833711462365 ) ) ;
#22873=CARTESIAN_POINT ( 'NONE',  ( 6.909265173666245374, -36.86491375218297861, 8.100132398494514163 ) ) ;
#22874=CARTESIAN_POINT ( 'NONE',  ( 2.595273106918288164, 2.906811120256387326, 9.741991644047248045 ) ) ;
#22875=CARTESIAN_POINT ( 'NONE',  ( -1.172603113866931501, -0.3455467477709202595, 9.987567862361071747 ) ) ;
#22894=VECTOR ( 'NONE', #9640, 1000.000000000000000 ) ;
#22899=CARTESIAN_POINT ( 'NONE',  ( -1.780494907546731120, -1.041382914740391019, 9.891980816076523908 ) ) ;
#22917=CARTESIAN_POINT ( 'NONE',  ( -1.111875982683548703, -1.111927553622429343, 9.927288994922816912 ) ) ;
#22923=ORIENTED_EDGE ( 'NONE', *, *, #20837, .T. ) ;
#22926=CARTESIAN_POINT ( 'NONE',  ( -0.6126904405382037622, -1.085824959725731231, 9.981352469109934233 ) ) ;
#22929=CARTESIAN_POINT ( 'NONE',  ( -1.370084944437349295, -0.09457992852950281026, 9.946805383069644790 ) ) ;
#22938=CARTESIAN_POINT ( 'NONE',  ( 1.249999999999999778, 0.000000000000000000, 3.333333333333333481 ) ) ;
#22947=CARTESIAN_POINT ( 'NONE',  ( -29.39982726364978660, -16.78152490921149109, 8.356839323120299312 ) ) ;
#22952=CARTESIAN_POINT ( 'NONE',  ( 1.011271242968677653, 0.7347315653656002477, -3.333333333333333481 ) ) ;
#22954=CARTESIAN_POINT ( 'NONE',  ( 0.9015506157962454026, -0.9804419706258503675, 9.951893257060014264 ) ) ;
#22957=CARTESIAN_POINT ( 'NONE',  ( -6.174150299305392053, 33.14591993373988998, 8.807470649214879543 ) ) ;
#22958=CARTESIAN_POINT ( 'NONE',  ( -1.066995270233474624, 33.23888904628638841, -3.760136334089591248 ) ) ;
#22963=CARTESIAN_POINT ( 'NONE',  ( 0.3862712429686978033, -1.188820645368937834, 10.00000000000000000 ) ) ;
#22964=CARTESIAN_POINT ( 'NONE',  ( -0.3370904143228927730, -0.2449105217885335917, 10.00000000000000000 ) ) ;
#22980=CARTESIAN_POINT ( 'NONE',  ( 0.9494396179258391966, -9.954826186926261755, 9.646707543097345905 ) ) ;
#22988=EDGE_CURVE ( 'NONE', #27847, #48161, #31267, .T. ) ;
#22989=CARTESIAN_POINT ( 'NONE',  ( 1.011271242968677653, 0.7347315653656002477, 3.333333333333333481 ) ) ;
#22995=EDGE_CURVE ( 'NONE', #40295, #5199, #12698, .T. ) ;
#23002=CARTESIAN_POINT ( 'NONE',  ( 6.174150299305392053, -50.00000000000000711, 8.807470649214879543 ) ) ;
#23003=FACE_OUTER_BOUND ( 'NONE', #9410, .T. ) ;
#23004=AXIS2_PLACEMENT_3D ( 'NONE', #19153, #9642, #44510 ) ;
#23005=CARTESIAN_POINT ( 'NONE',  ( 1.593403307200061292, 0.6097984806595578844, 9.912102921405024247 ) ) ;
#23011=CARTESIAN_POINT ( 'NONE',  ( 3.975459390375365665, 0.2195152216756870167, 1.992221491942114397E-15 ) ) ;
#23012=CARTESIAN_POINT ( 'NONE',  ( 0.3910393408562611861, 3.877122853646846945, 9.741991644046958498 ) ) ;
#23016=CARTESIAN_POINT ( 'NONE',  ( -33.14391172085785797, -37.72293746533095060, -8.016098858316199838 ) ) ;
#23021=CARTESIAN_POINT ( 'NONE',  ( 1.111875982684040753, 1.111927553622385378, 9.927288994922816912 ) ) ;
#23029=EDGE_CURVE ( 'NONE', #50425, #36390, #16976, .T. ) ;
#23030=CARTESIAN_POINT ( 'NONE',  ( 0.8285222815141930486, 1.889008401827334094, 9.886433018048068178 ) ) ;
#23035=CARTESIAN_POINT ( 'NONE',  ( 9.919534718721870092, -1.461167986676253916, 9.524510970297029644 ) ) ;
#23051=B_SPLINE_CURVE_WITH_KNOTS ( 'NONE', 3,
 ( #5240, #48294, #40655, #5491 ),
 .UNSPECIFIED., .F., .F.,
 ( 4, 4 ),
 ( 5.536300823665787423E-16, 0.009782300387714815831 ),
 .UNSPECIFIED. ) ;
#23052=CARTESIAN_POINT ( 'NONE',  ( 0.1469336902871260508, 1.496274467947966258, 9.953784399990622589 ) ) ;
#23065=CARTESIAN_POINT ( 'NONE',  ( -14.48769039275601145, -30.44468701195584970, 8.807470649214879543 ) ) ;
#23075=ORIENTED_EDGE ( 'NONE', *, *, #8107, .T. ) ;
#23077=CARTESIAN_POINT ( 'NONE',  ( 49.89397392339123627, -8.245536726716670373, 7.906207997025717304 ) ) ;
#23079=ORIENTED_EDGE ( 'NONE', *, *, #6489, .F. ) ;
#23087=ADVANCED_FACE ( 'NONE', ( #4560 ), #7216, .T. ) ;
#23091=ORIENTED_EDGE ( 'NONE', *, *, #48296, .F. ) ;
#23096=EDGE_CURVE ( 'NONE', #16958, #26846, #47558, .T. ) ;
#23103=CARTESIAN_POINT ( 'NONE',  ( -9.174209336589896679, -3.979181203266159095, 9.646707543097347681 ) ) ;
#23120=CARTESIAN_POINT ( 'NONE',  ( -34.95136153415531766, 36.40974830873496870, 8.356839323120299312 ) ) ;
#23121=FACE_OUTER_BOUND ( 'NONE', #9037, .T. ) ;
#23133=CARTESIAN_POINT ( 'NONE',  ( 2.188678504086826848, -0.3267089737525829540, 9.881002359080282460 ) ) ;
#23144=B_SPLINE_CURVE_WITH_KNOTS ( 'NONE', 3,
 ( #25660, #48194, #41052, #49205 ),
 .UNSPECIFIED., .F., .F.,
 ( 4, 4 ),
 ( 0.001403500796105026753, 0.001586656765098990764 ),
 .UNSPECIFIED. ) ;
#23151=ORIENTED_EDGE ( 'NONE', *, *, #41866, .T. ) ;
#23153=CARTESIAN_POINT ( 'NONE',  ( 33.43156050989131955, -4.370686678976570150, 8.807470649214879543 ) ) ;
#23155=ORIENTED_EDGE ( 'NONE', *, *, #29637, .F. ) ;
#23159=CARTESIAN_POINT ( 'NONE',  ( -4.207128120815918256E-14, 3.058192377181588826E-14, 10.00000000000000000 ) ) ;
#23160=EDGE_CURVE ( 'NONE', #45145, #19313, #35988, .T. ) ;
#23163=ORIENTED_EDGE ( 'NONE', *, *, #21429, .F. ) ;
#23169=CARTESIAN_POINT ( 'NONE',  ( -10.30302290646040575, -13.08520913973572419, -9.683996418299976483 ) ) ;
#23171=ORIENTED_EDGE ( 'NONE', *, *, #25288, .T. ) ;
#23174=ADVANCED_FACE ( 'NONE', ( #48871 ), #34682, .T. ) ;
#23183=CARTESIAN_POINT ( 'NONE',  ( -14.29087950072019098, -9.652079258044555132, 8.727788335465566760 ) ) ;
#23184=EDGE_LOOP ( 'NONE', ( #17502, #32904, #42528, #38393 ) ) ;
#23198=B_SPLINE_SURFACE_WITH_KNOTS ( 'NONE', 3, 3, ( 
 ( #38064, #30358, #38580, #26500 ),
 ( #2875, #33953, #14695, #10845 ),
 ( #42137, #7002, #22646, #50046 ),
 ( #38325, #3134, #34731, #18784 ) ),
 .UNSPECIFIED., .F., .F., .F.,
 ( 4, 4 ),
 ( 4, 4 ),
 ( 0.000000000000000000, 1.000000000000000000 ),
 ( 0.000000000000000000, 1.000000000000000000 ),
 .UNSPECIFIED. ) ;
#23215=CARTESIAN_POINT ( 'NONE',  ( 3.996390545799824334, -16.57371371864897469, 8.953103998512858652 ) ) ;
#23221=CARTESIAN_POINT ( 'NONE',  ( -3.229232847726260403, 16.57333684275945629, 9.178419661560148768 ) ) ;
#23227=CARTESIAN_POINT ( 'NONE',  ( 1.419290803332528661, 0.2086015876289408766, 9.950105812514292936 ) ) ;
#23230=CARTESIAN_POINT ( 'NONE',  ( 1.072341519475944915, -1.326978504731018083, 9.912102921405038458 ) ) ;
#23231=CARTESIAN_POINT ( 'NONE',  ( 23.79193388295309219, 28.98609808355011452, -9.422646554964176246 ) ) ;
#23239=CARTESIAN_POINT ( 'NONE',  ( 44.99506233596247995, 23.32283626942318833, 7.455576670931136185 ) ) ;
#23241=VERTEX_POINT ( 'NONE', #46037 ) ;
#23242=DIRECTION ( 'NONE',  ( 0.4374820812098862421, -0.3178493372392685590, -0.8411784753765542133 ) ) ;
#23246=CARTESIAN_POINT ( 'NONE',  ( 12.15085308559846844, -11.68662139125803989, 2.590526750877053086 ) ) ;
#23256=VERTEX_POINT ( 'NONE', #37901 ) ;
#23258=CARTESIAN_POINT ( 'NONE',  ( -33.43156050989129824, 4.370686678976795747, 8.807470649214879543 ) ) ;
#23264=ORIENTED_EDGE ( 'NONE', *, *, #35405, .F. ) ;
#23276=CIRCLE ( 'NONE', #41308, 10.00000000000000000 ) ;
#23277=CARTESIAN_POINT ( 'NONE',  ( -49.46074318306825290, 9.578883844007165749, 8.807470649214879543 ) ) ;
#23281=CARTESIAN_POINT ( 'NONE',  ( 0.4402948852767718524, -2.015117899693914527, 9.894754715216725671 ) ) ;
#23284=B_SPLINE_CURVE_WITH_KNOTS ( 'NONE', 3,
 ( #5537, #2205, #32248, #1456, #47842, #36362 ),
 .UNSPECIFIED., .F., .F.,
 ( 4, 2, 4 ),
 ( 8.498374721940738929E-18, 0.009877169331704831884, 0.01975433866340964989 ),
 .UNSPECIFIED. ) ;
#23291=CARTESIAN_POINT ( 'NONE',  ( 35.51846793572394034, -35.99772139009119343, 7.906207997025717304 ) ) ;
#23302=FACE_OUTER_BOUND ( 'NONE', #14771, .T. ) ;
#23306=CARTESIAN_POINT ( 'NONE',  ( -45.42829307628559832, -21.98948915213271960, 8.356839323120299312 ) ) ;
#23310=CARTESIAN_POINT ( 'NONE',  ( 6.174150299305392053, -50.00000000000000711, 8.807470649214879543 ) ) ;
#23321=EDGE_CURVE ( 'NONE', #31351, #11996, #6570, .T. ) ;
#23325=CARTESIAN_POINT ( 'NONE',  ( -46.11867747200561496, 19.86470446310265103, -8.016098858316205167 ) ) ;
#23335=ORIENTED_EDGE ( 'NONE', *, *, #11099, .F. ) ;
#23336=CARTESIAN_POINT ( 'NONE',  ( 0.1287570809895575430, 0.3962735484563150168, 10.00000000000000000 ) ) ;
#23379=CARTESIAN_POINT ( 'NONE',  ( 0.3862712429686727678, 1.188820645368945605, 3.333333333333333481 ) ) ;
#23381=CARTESIAN_POINT ( 'NONE',  ( 20.40054609052976531, -26.26366202847973597, -3.760136334089591248 ) ) ;
#23393=ORIENTED_EDGE ( 'NONE', *, *, #11712, .T. ) ;
#23398=CARTESIAN_POINT ( 'NONE',  ( -0.3862712429686809279, -1.188820645368943163, 3.333333333333333481 ) ) ;
#23416=AXIS2_PLACEMENT_3D ( 'NONE', #26297, #18576, #2437 ) ;
#23429=VERTEX_POINT ( 'NONE', #1853 ) ;
#23438=ORIENTED_EDGE ( 'NONE', *, *, #34657, .T. ) ;
#23445=ORIENTED_EDGE ( 'NONE', *, *, #48086, .T. ) ;
#23450=CARTESIAN_POINT ( 'NONE',  ( 2.637606039711250183, 0.1407378881970818563, 9.847478953136986846 ) ) ;
#23452=CARTESIAN_POINT ( 'NONE',  ( -1.057156451998854996, 0.7920882637787067804, 9.943883492372851407 ) ) ;
#23457=CARTESIAN_POINT ( 'NONE',  ( -34.08355720199904226, 2.371364769369340042, 7.455576670931136185 ) ) ;
#23461=CARTESIAN_POINT ( 'NONE',  ( 4.763548243873389154, -16.57409059453848599, 8.727788335465566760 ) ) ;
#23475=CARTESIAN_POINT ( 'NONE',  ( 36.01122090644292228, 10.59066248886193407, -2.490396854064191867 ) ) ;
#23476=ORIENTED_EDGE ( 'NONE', *, *, #11162, .F. ) ;
#23495=CARTESIAN_POINT ( 'NONE',  ( -0.4166666666666664631, 0.000000000000000000, 10.00000000000000000 ) ) ;
#23496=CARTESIAN_POINT ( 'NONE',  ( -8.277096487746778308, 50.00000000000000711, 7.455576670931136185 ) ) ;
#23513=CARTESIAN_POINT ( 'NONE',  ( 4.353119224256710496, 9.002796955358187247, 0.000000000000000000 ) ) ;
#23517=FACE_OUTER_BOUND ( 'NONE', #33735, .T. ) ;
#23523=VERTEX_POINT ( 'NONE', #30826 ) ;
#23524=CARTESIAN_POINT ( 'NONE',  ( 1.377509002708426689, -0.6027468487254984408, 9.927319414211227766 ) ) ;
#23525=B_SPLINE_CURVE_WITH_KNOTS ( 'NONE', 3,
 ( #36807, #13427, #48031, #28329 ),
 .UNSPECIFIED., .F., .F.,
 ( 4, 4 ),
 ( 0.0009679537044784459771, 0.001281751046851268335 ),
 .UNSPECIFIED. ) ;
#23528=AXIS2_PLACEMENT_3D ( 'NONE', #15599, #34863, #4050 ) ;
#23530=CARTESIAN_POINT ( 'NONE',  ( -0.3862712429686977478, 1.188820645368937390, -10.00000000000000000 ) ) ;
#23549=CARTESIAN_POINT ( 'NONE',  ( 30.77287599203632951, 12.70002479445995824, 3.199614146704519602 ) ) ;
#23550=CARTESIAN_POINT ( 'NONE',  ( -0.3139796262078424216, 1.230474926876623076, 9.975314328424618182 ) ) ;
#23561=CARTESIAN_POINT ( 'NONE',  ( 13.59579750444771307, -10.60877755095900632, 8.727788335465566760 ) ) ;
#23566=FACE_OUTER_BOUND ( 'NONE', #12209, .T. ) ;
#23572=CARTESIAN_POINT ( 'NONE',  ( -6.875132362119187768, 50.00000000000000711, 8.356839323120299312 ) ) ;
#23578=CARTESIAN_POINT ( 'NONE',  ( 33.38053581724552288, 17.16548397897151546, 4.835783797351798974 ) ) ;
#23589=CARTESIAN_POINT ( 'NONE',  ( 30.12518629743562926, 14.70074613238908157, 1.847720168420772691 ) ) ;
#23592=ORIENTED_EDGE ( 'NONE', *, *, #25591, .T. ) ;
#23593=CARTESIAN_POINT ( 'NONE',  ( 33.86622497129647513, -3.037805405904928868, 7.906207997025717304 ) ) ;
#23605=CARTESIAN_POINT ( 'NONE',  ( -26.18032376592659105, 21.95228666728381128, 7.455576670931136185 ) ) ;
#23606=CARTESIAN_POINT ( 'NONE',  ( -1.365263087672800246, 0.5437404457009007430, 9.958264684458713489 ) ) ;
#23615=CARTESIAN_POINT ( 'NONE',  ( -2.945500763482279627, -16.64098165802040086, -9.008049429158100807 ) ) ;
#23618=LINE ( 'NONE', #32, #36899 ) ;
#23620=B_SPLINE_CURVE_WITH_KNOTS ( 'NONE', 3,
 ( #32535, #8165, #20711, #9160 ),
 .UNSPECIFIED., .F., .F.,
 ( 4, 4 ),
 ( 0.000000000000000000, 0.2562577668812812681 ),
 .UNSPECIFIED. ) ;
#23622=B_SPLINE_SURFACE_WITH_KNOTS ( 'NONE', 3, 3, ( 
 ( #39079, #7509, #46456, #15964 ),
 ( #24178, #4670, #35478, #12118 ),
 ( #39835, #11347, #15448, #23909 ),
 ( #12352, #67, #23658, #27763 ) ),
 .UNSPECIFIED., .F., .F., .F.,
 ( 4, 4 ),
 ( 4, 4 ),
 ( 0.000000000000000000, 1.000000000000000000 ),
 ( 0.000000000000000000, 1.000000000000000000 ),
 .UNSPECIFIED. ) ;
#23629=CARTESIAN_POINT ( 'NONE',  ( -5.888214538810513154, -16.20866436362413410, 8.727788335465566760 ) ) ;
#23632=CARTESIAN_POINT ( 'NONE',  ( -0.1287570809895658697, 0.3962735484563123523, 10.00000000000000000 ) ) ;
#23649=CLOSED_SHELL ( 'NONE', ( #38454, #41241, #30012, #41543, #32714, #3350, #18528, #40434, #14742, #19911, #34627, #36375, #41185, #6078, #36535, #20616, #37023, #13381, #25912, #50553, #38187, #1991, #40601, #49123, #31798, #47859, #44952, #48704, #21155, #37144, #36253, #30126, #9841, #27793, #15870, #43499, #44323, #41576, #7985, #7833, #4898, #34125, #45278, #9805, #30882, #45224, #33039, #47747, #19436, #14701, #40900, #36205, #48776, #19546, #13971, #20048, #20904, #15829, #19023, #50690, #46212, #14994, #22664, #8619, #1087, #40790, #44916, #2599, #33429, #50564, #13711, #20709, #34920, #19571, #50093, #28041, #16439, #5131, #4572, #10858, #21687, #46534, #8756, #26732, #18388, #5539, #42285, #37524, #10651, #25491, #14645, #14004, #43671, #40503, #2136, #8123, #46220, #36572, #39826, #45026, #1889, #17716, #43291, #34654, #11581, #33346, #138, #42824, #25518, #32287, #38051, #13623, #29002, #10201, #14891, #21179, #13426, #32803, #29361, #18042, #48064, #39175, #23087, #32578, #24780, #29629, #29702, #4972, #49184, #13894, #22171, #7172, #25532, #21948, #49262, #28913, #27147, #21570, #32699, #8446, #15943, #41277, #108, #14938, #45843, #43032, #14150, #13252, #8994, #9610, #6083, #6693, #24637, #21754, #2289, #30842, #45000, #31344, #35071, #2034, #16031, #28226, #14941, #12441, #37446, #42162, #30869, #15936, #23174, #2797, #12941, #34957, #44115, #39295, #33355, #47074, #23971, #4304 ) ) ;
#23650=B_SPLINE_CURVE_WITH_KNOTS ( 'NONE', 3,
 ( #7678, #7430, #15879, #39495 ),
 .UNSPECIFIED., .F., .F.,
 ( 4, 4 ),
 ( 0.001152428489661413242, 0.001623376834729681802 ),
 .UNSPECIFIED. ) ;
#23657=ORIENTED_EDGE ( 'NONE', *, *, #20837, .F. ) ;
#23658=CARTESIAN_POINT ( 'NONE',  ( -5.888214538810513154, -16.20866436362413410, 8.727788335465566760 ) ) ;
#23673=EDGE_CURVE ( 'NONE', #13148, #13812, #6509, .T. ) ;
#23678=EDGE_LOOP ( 'NONE', ( #49408, #46704, #44083, #5595, #24029 ) ) ;
#23693=CARTESIAN_POINT ( 'NONE',  ( -1.249999999999999778, 0.000000000000000000, -3.333333333333333481 ) ) ;
#23711=CARTESIAN_POINT ( 'NONE',  ( -0.6440276692615888310, -16.64212148744554298, -9.683996418299976483 ) ) ;
#23726=LINE ( 'NONE', #27320, #17307 ) ;
#23729=CARTESIAN_POINT ( 'NONE',  ( 1.249999999999999778, 0.000000000000000000, 3.333333333333333481 ) ) ;
#23745=VERTEX_POINT ( 'NONE', #19503 ) ;
#23762=AXIS2_PLACEMENT_3D ( 'NONE', #41041, #33859, #2784 ) ;
#23768=DIRECTION ( 'NONE',  ( -1.000000000000000000, 0.000000000000000000, 0.000000000000000000 ) ) ;
#23782=CARTESIAN_POINT ( 'NONE',  ( 1.250000000000000222, 0.000000000000000000, -10.00000000000000000 ) ) ;
#23786=VERTEX_POINT ( 'NONE', #1037 ) ;
#23797=CARTESIAN_POINT ( 'NONE',  ( 0.6126904405382156416, 1.085824959725723016, 9.981352469109932457 ) ) ;
#23800=CARTESIAN_POINT ( 'NONE',  ( -1.222012661920452326, 0.2471648704738776681, 9.981352469109934233 ) ) ;
#23825=VECTOR ( 'NONE', #28020, 1000.000000000000114 ) ;
#23826=CARTESIAN_POINT ( 'NONE',  ( -4.672045878990125800, 33.19353511768168374, 1.847720168420772691 ) ) ;
#23832=CARTESIAN_POINT ( 'NONE',  ( 1.249999999999999778, 0.000000000000000000, 10.00000000000000000 ) ) ;
#23843=CARTESIAN_POINT ( 'NONE',  ( -38.06347959788612201, 17.13191708601497609, -8.080361901872242569 ) ) ;
#23853=ORIENTED_EDGE ( 'NONE', *, *, #4127, .T. ) ;
#23860=ORIENTED_EDGE ( 'NONE', *, *, #10516, .F. ) ;
#23873=VERTEX_POINT ( 'NONE', #44856 ) ;
#23874=CARTESIAN_POINT ( 'NONE',  ( -4.641001526964560142, -50.00000000000000711, -8.016098858316199838 ) ) ;
#23881=CARTESIAN_POINT ( 'NONE',  ( -1.042245359060422816, -0.7067879234688214662, 9.974012008644017158 ) ) ;
#23882=CARTESIAN_POINT ( 'NONE',  ( 0.3862712429686894766, -1.188820645368940276, -10.00000000000000000 ) ) ;
#23889=CARTESIAN_POINT ( 'NONE',  ( 44.99506233596247995, 23.32283626942318833, 7.455576670931136185 ) ) ;
#23909=CARTESIAN_POINT ( 'NONE',  ( 0.3370904143228959926, -0.2449105217885284291, 10.00000000000000000 ) ) ;
#23928=AXIS2_PLACEMENT_3D ( 'NONE', #14431, #21620, #13672 ) ;
#23933=CARTESIAN_POINT ( 'NONE',  ( -28.52604530808686079, -41.07801380285659576, -3.760136334089591248 ) ) ;
#23941=CARTESIAN_POINT ( 'NONE',  ( -1.066995270233474624, 50.00000000000000711, -3.760136334089591248 ) ) ;
#23953=CARTESIAN_POINT ( 'NONE',  ( -16.02661358026017879, -4.530191650547607196, -9.683996418299976483 ) ) ;
#23958=CARTESIAN_POINT ( 'NONE',  ( -2.538055338523173443, -50.00000000000000000, -9.367992836599951190 ) ) ;
#23961=CARTESIAN_POINT ( 'NONE',  ( 4.672045878990125800, -50.00000000000000711, 1.847720168420772691 ) ) ;
#23966=CARTESIAN_POINT ( 'NONE',  ( -40.32982405930701475, -10.56057144604259079, -9.387872844313825738 ) ) ;
#23971=ADVANCED_FACE ( 'NONE', ( #14590 ), #35950, .T. ) ;
#23979=EDGE_CURVE ( 'NONE', #48228, #13812, #29841, .T. ) ;
#23990=CARTESIAN_POINT ( 'NONE',  ( -1.011271242968693862, 0.7347315653655780432, 10.00000000000000000 ) ) ;
#24005=B_SPLINE_CURVE_WITH_KNOTS ( 'NONE', 3,
 ( #38095, #2906, #49820, #23452 ),
 .UNSPECIFIED., .F., .F.,
 ( 4, 4 ),
 ( 0.0006669682284780878911, 0.0007799402130919236807 ),
 .UNSPECIFIED. ) ;
#24029=ORIENTED_EDGE ( 'NONE', *, *, #20906, .F. ) ;
#24031=CARTESIAN_POINT ( 'NONE',  ( -0.02889939370780074401, 1.394750214493988283, 9.955131761384901523 ) ) ;
#24050=CARTESIAN_POINT ( 'NONE',  ( 0.2773062244624638351, -1.251557370488896481, 9.948547179989619238 ) ) ;
#24051=VERTEX_POINT ( 'NONE', #227 ) ;
#24057=B_SPLINE_SURFACE_WITH_KNOTS ( 'NONE', 3, 3, ( 
 ( #44, #31854, #16193, #24154 ),
 ( #15676, #35719, #31348, #12578 ),
 ( #16683, #4139, #43370, #299 ),
 ( #15941, #31609, #47194, #4648 ) ),
 .UNSPECIFIED., .F., .F., .F.,
 ( 4, 4 ),
 ( 4, 4 ),
 ( 0.000000000000000000, 1.000000000000000000 ),
 ( 0.000000000000000000, 1.000000000000000000 ),
 .UNSPECIFIED. ) ;
#24064=CARTESIAN_POINT ( 'NONE',  ( -1.335416683881408995, 0.4035165624839831544, 9.955131761384903299 ) ) ;
#24068=ORIENTED_EDGE ( 'NONE', *, *, #23096, .F. ) ;
#24077=VERTEX_POINT ( 'NONE', #7930 ) ;
#24083=ORIENTED_EDGE ( 'NONE', *, *, #48331, .T. ) ;
#24088=CARTESIAN_POINT ( 'NONE',  ( -14.76429217231967428, -8.192625680377590314, 9.178419661560148768 ) ) ;
#24092=FACE_BOUND ( 'NONE', #24332, .T. ) ;
#24109=CARTESIAN_POINT ( 'NONE',  ( -49.67735855322972327, 8.912210285362091255, 8.356839323120299312 ) ) ;
#24110=B_SPLINE_CURVE_WITH_KNOTS ( 'NONE', 3,
 ( #43816, #48130, #8930, #24584 ),
 .UNSPECIFIED., .F., .F.,
 ( 4, 4 ),
 ( 0.0006669682284780878911, 0.0007799402130920260294 ),
 .UNSPECIFIED. ) ;
#24130=CARTESIAN_POINT ( 'NONE',  ( -0.4426377647354682865, -1.666766018367764834, 9.928159647716134018 ) ) ;
#24133=CARTESIAN_POINT ( 'NONE',  ( -1.114871695981121125, 0.4953159757245923500, 9.963925895596188909 ) ) ;
#24148=CARTESIAN_POINT ( 'NONE',  ( -32.87128375420900284, -6.537745902885379046, -8.466730184410787174 ) ) ;
#24154=CARTESIAN_POINT ( 'NONE',  ( 0.3862712429686978033, -1.188820645368937834, 10.00000000000000000 ) ) ;
#24159=EDGE_LOOP ( 'NONE', ( #49761, #41522, #8163 ) ) ;
#24160=CARTESIAN_POINT ( 'NONE',  ( -0.3862712429686809279, -1.188820645368942941, 9.972675548442463622 ) ) ;
#24164=CARTESIAN_POINT ( 'NONE',  ( 1.104213410210670876, 0.6509177773818231039, 9.976582533991679824 ) ) ;
#24172=FACE_BOUND ( 'NONE', #12187, .T. ) ;
#24178=CARTESIAN_POINT ( 'NONE',  ( -23.82716369509181575, -44.49195112875988656, 8.356839323120299312 ) ) ;
#24186=CARTESIAN_POINT ( 'NONE',  ( -0.8282505383454070724, -1.889063466747028297, 9.894754715216727448 ) ) ;
#24192=VERTEX_POINT ( 'NONE', #40736 ) ;
#24195=ORIENTED_EDGE ( 'NONE', *, *, #39990, .T. ) ;
#24196=CARTESIAN_POINT ( 'NONE',  ( 0.8101544858819106354, 3.892041491916302220, 3.247139498068311703 ) ) ;
#24200=CARTESIAN_POINT ( 'NONE',  ( -22.69295089195507487, -45.31600496604688999, 7.455576670931136185 ) ) ;
#24203=LINE ( 'NONE', #39864, #49248 ) ;
#24212=ORIENTED_EDGE ( 'NONE', *, *, #9505, .T. ) ;
#24235=ORIENTED_EDGE ( 'NONE', *, *, #19752, .F. ) ;
#24236=EDGE_CURVE ( 'NONE', #22111, #17682, #24832, .T. ) ;
#24246=EDGE_CURVE ( 'NONE', #13764, #39166, #7768, .T. ) ;
#24258=CARTESIAN_POINT ( 'NONE',  ( 45.21167770612395742, 22.65616271077811206, 7.906207997025717304 ) ) ;
#24262=ORIENTED_EDGE ( 'NONE', *, *, #37894, .F. ) ;
#24263=ORIENTED_EDGE ( 'NONE', *, *, #37948, .F. ) ;
#24264=EDGE_CURVE ( 'NONE', #2158, #45646, #18724, .T. ) ;
#24273=CARTESIAN_POINT ( 'NONE',  ( 1.437255894074055185, -3.713052624461447682, -1.301042606982605321E-15 ) ) ;
#24274=CARTESIAN_POINT ( 'NONE',  ( -5.888214538810513154, -16.20866436362413410, 8.727788335465566760 ) ) ;
#24276=CARTESIAN_POINT ( 'NONE',  ( 29.61572577327002520, 16.11461842845735859, 8.807470649214879543 ) ) ;
#24307=CARTESIAN_POINT ( 'NONE',  ( -35.34822294759187145, -12.62826869953532416, -3.721387749823057423 ) ) ;
#24310=CARTESIAN_POINT ( 'NONE',  ( 35.51846793572394034, -35.99772139009119343, 7.906207997025717304 ) ) ;
#24313=CARTESIAN_POINT ( 'NONE',  ( 0.6803378293928957765, 1.026336842001439154, 9.975326647351305809 ) ) ;
#24316=CARTESIAN_POINT ( 'NONE',  ( -4.207128120815918256E-14, 3.058192377181588826E-14, 10.00000000000000000 ) ) ;
#24320=CARTESIAN_POINT ( 'NONE',  ( -24.47767542868268364, 23.18653802921800278, 8.807470649214879543 ) ) ;
#24332=EDGE_LOOP ( 'NONE', ( #49977, #17468 ) ) ;
#24354=CARTESIAN_POINT ( 'NONE',  ( 1.320835335343329753, -0.01943189459118491516, 9.943883492372847854 ) ) ;
#24359=ORIENTED_EDGE ( 'NONE', *, *, #43147, .T. ) ;
#24367=ORIENTED_EDGE ( 'NONE', *, *, #11162, .T. ) ;
#24379=EDGE_CURVE ( 'NONE', #4784, #47768, #24842, .T. ) ;
#24385=ORIENTED_EDGE ( 'NONE', *, *, #28846, .F. ) ;
#24399=B_SPLINE_CURVE_WITH_KNOTS ( 'NONE', 3,
 ( #19454, #15106, #46378, #19960 ),
 .UNSPECIFIED., .F., .F.,
 ( 4, 4 ),
 ( 0.000000000000000000, 0.0001252128669263166563 ),
 .UNSPECIFIED. ) ;
#24402=CARTESIAN_POINT ( 'NONE',  ( -12.97493236725075683, 11.05939663307000664, 8.953103998512858652 ) ) ;
#24403=PLANE ( 'NONE',  #1673 ) ;
#24428=ORIENTED_EDGE ( 'NONE', *, *, #30281, .T. ) ;
#24433=ORIENTED_EDGE ( 'NONE', *, *, #21429, .T. ) ;
#24440=CARTESIAN_POINT ( 'NONE',  ( 1.114871695981101585, -0.4953159757246433093, 9.963925895596188909 ) ) ;
#24447=B_SPLINE_CURVE_WITH_KNOTS ( 'NONE', 3,
 ( #50175, #14828, #34862, #3271 ),
 .UNSPECIFIED., .F., .F.,
 ( 4, 4 ),
 ( 0.9811748202683091558, 0.9878904167554123372 ),
 .UNSPECIFIED. ) ;
#24449=DIRECTION ( 'NONE',  ( 0.000000000000000000, 0.000000000000000000, -1.000000000000000000 ) ) ;
#24457=EDGE_CURVE ( 'NONE', #4784, #41616, #43192, .T. ) ;
#24475=CARTESIAN_POINT ( 'NONE',  ( -4.376737514451251698, 37.28021197136517628, 1.982731392810406668 ) ) ;
#24476=CARTESIAN_POINT ( 'NONE',  ( 2.961022939495062900, -16.59676755884084187, 2.590526750877053086 ) ) ;
#24477=ORIENTED_EDGE ( 'NONE', *, *, #43990, .T. ) ;
#24479=B_SPLINE_SURFACE_WITH_KNOTS ( 'NONE', 3, 3, ( 
 ( #37810, #17531, #10084, #13912 ),
 ( #29838, #29336, #9825, #25482 ),
 ( #5979, #17785, #33451, #11093 ),
 ( #22637, #31104, #39077, #42884 ) ),
 .UNSPECIFIED., .F., .F., .F.,
 ( 4, 4 ),
 ( 4, 4 ),
 ( 0.000000000000000000, 1.000000000000000000 ),
 ( 0.000000000000000000, 1.000000000000000000 ),
 .UNSPECIFIED. ) ;
#24481=CARTESIAN_POINT ( 'NONE',  ( -0.3862712429686895876, 1.188820645368940720, -3.333333333333333481 ) ) ;
#24482=FACE_OUTER_BOUND ( 'NONE', #38583, .T. ) ;
#24491=VECTOR ( 'NONE', #6299, 1000.000000000000000 ) ;
#24493=CARTESIAN_POINT ( 'NONE',  ( 7.929028631756658285, -0.8360402172235281704, 8.538092108323347418E-15 ) ) ;
#24498=CARTESIAN_POINT ( 'NONE',  ( 0.4166666666666664631, -0.000000000000000000, -10.00000000000000000 ) ) ;
#24499=CARTESIAN_POINT ( 'NONE',  ( 49.46074318306830975, -9.578883844006833570, 8.807470649214879543 ) ) ;
#24501=ORIENTED_EDGE ( 'NONE', *, *, #27760, .T. ) ;
#24503=CARTESIAN_POINT ( 'NONE',  ( 8.277096487746778308, -45.55573069994827051, 7.455576670931136185 ) ) ;
#24533=CARTESIAN_POINT ( 'NONE',  ( 30.87089393895375267, -12.69923079256617449, -9.367992836599954742 ) ) ;
#24543=FACE_OUTER_BOUND ( 'NONE', #2646, .T. ) ;
#24547=CARTESIAN_POINT ( 'NONE',  ( -29.38926261462371770, 40.45084971874734237, 0.000000000000000000 ) ) ;
#24562=VECTOR ( 'NONE', #34176, 1000.000000000000000 ) ;
#24570=CARTESIAN_POINT ( 'NONE',  ( -1.249999999999999778, 0.000000000000000000, 10.00000000000000000 ) ) ;
#24571=CARTESIAN_POINT ( 'NONE',  ( 0.3370904143228981575, -0.2449105217885261532, 10.00000000000000000 ) ) ;
#24583=EDGE_CURVE ( 'NONE', #5629, #40397, #165, .T. ) ;
#24584=CARTESIAN_POINT ( 'NONE',  ( -0.3896797354171960270, 1.262193838292709147, 9.943883492372847854 ) ) ;
#24601=DIRECTION ( 'NONE',  ( 0.000000000000000000, 1.000000000000000000, 0.000000000000000000 ) ) ;
#24620=ORIENTED_EDGE ( 'NONE', *, *, #18086, .T. ) ;
#24627=CARTESIAN_POINT ( 'NONE',  ( -6.174150299305392053, 50.00000000000000711, 8.807470649214879543 ) ) ;
#24629=CARTESIAN_POINT ( 'NONE',  ( 0.3370904143228947158, 0.2449105217885311492, -10.00000000000000000 ) ) ;
#24636=VERTEX_POINT ( 'NONE', #48571 ) ;
#24637=ADVANCED_FACE ( 'NONE', ( #5005 ), #3510, .T. ) ;
#24646=CARTESIAN_POINT ( 'NONE',  ( -16.69947034530963847, 2.312583065866374632, 2.590526750877053086 ) ) ;
#24647=EDGE_CURVE ( 'NONE', #13851, #17745, #43748, .T. ) ;
#24648=CARTESIAN_POINT ( 'NONE',  ( 0.000000000000000000, 0.000000000000000000, 10.00000000000000000 ) ) ;
#24655=CARTESIAN_POINT ( 'NONE',  ( -36.08557433729205144, 35.58569447144795816, 7.455576670931136185 ) ) ;
#24679=VECTOR ( 'NONE', #11985, 1000.000000000000114 ) ;
#24690=CARTESIAN_POINT ( 'NONE',  ( -1.540571744149449751, 1.371626741452969034, 9.889206917020301191 ) ) ;
#24691=CARTESIAN_POINT ( 'NONE',  ( -0.3862712429686977478, 1.188820645368937390, -10.00000000000000000 ) ) ;
#24697=B_SPLINE_CURVE_WITH_KNOTS ( 'NONE', 3,
 ( #5126, #30181, #22484, #29679 ),
 .UNSPECIFIED., .F., .F.,
 ( 4, 4 ),
 ( 0.9811748202683103770, 0.9878904167554123372 ),
 .UNSPECIFIED. ) ;
#24700=CARTESIAN_POINT ( 'NONE',  ( 0.3910393408562611861, 3.877122853646846945, 9.741991644046958498 ) ) ;
#24706=CARTESIAN_POINT ( 'NONE',  ( 1.249999999999999778, -0.000000000000000000, -3.333333333333333481 ) ) ;
#24707=CARTESIAN_POINT ( 'NONE',  ( 0.3862712429686810944, 1.188820645368943607, -3.333333333333333481 ) ) ;
#24714=CARTESIAN_POINT ( 'NONE',  ( -4.207128120815918256E-14, 3.058192377181588826E-14, 10.00000000000000000 ) ) ;
#24723=CARTESIAN_POINT ( 'NONE',  ( -6.875132362119187768, 50.00000000000000711, 8.356839323120299312 ) ) ;
#24731=CARTESIAN_POINT ( 'NONE',  ( -9.281355226777547429, 3.722424633806451943, 0.000000000000000000 ) ) ;
#24739=CARTESIAN_POINT ( 'NONE',  ( 1.780432407520001536, 1.041450996408479046, 9.894754715216729224 ) ) ;
#24743=B_SPLINE_CURVE_WITH_KNOTS ( 'NONE', 3,
 ( #32363, #47961, #32879, #33131 ),
 .UNSPECIFIED., .F., .F.,
 ( 4, 4 ),
 ( 0.000000000000000000, 0.2562577668812811016 ),
 .UNSPECIFIED. ) ;
#24744=CARTESIAN_POINT ( 'NONE',  ( -5.873104089934114924, -0.6060605173725300832, 9.586754400234157814 ) ) ;
#24757=CARTESIAN_POINT ( 'NONE',  ( -0.3905129037392560676, 2.126717070043232738, 9.885585981620938156 ) ) ;
#24761=CARTESIAN_POINT ( 'NONE',  ( 29.18392875402930997, 17.44843138996603216, 7.906207997025717304 ) ) ;
#24762=CARTESIAN_POINT ( 'NONE',  ( 0.6721397084974982672, 9.977385840602783773, 2.154851817814940063E-15 ) ) ;
#24769=CARTESIAN_POINT ( 'NONE',  ( 1.011271242968683648, 0.7347315653655930312, -10.00000000000000000 ) ) ;
#24776=CARTESIAN_POINT ( 'NONE',  ( 28.96803024440893992, 18.11533787072037072, 7.455576670931136185 ) ) ;
#24778=ORIENTED_EDGE ( 'NONE', *, *, #6602, .T. ) ;
#24780=ADVANCED_FACE ( 'NONE', ( #18305 ), #39626, .T. ) ;
#24781=CARTESIAN_POINT ( 'NONE',  ( -50.11058929355264979, 7.578863168071929834, 7.455576670931136185 ) ) ;
#24782=CARTESIAN_POINT ( 'NONE',  ( -30.65355587399070814, 13.36566953343609043, -8.917361510505369182 ) ) ;
#24783=ORIENTED_EDGE ( 'NONE', *, *, #13429, .T. ) ;
#24790=LINE ( 'NONE', #44760, #18490 ) ;
#24791=CARTESIAN_POINT ( 'NONE',  ( 31.94178169330218964, -9.256608784833820991, -3.760136334089591248 ) ) ;
#24792=FACE_OUTER_BOUND ( 'NONE', #36449, .T. ) ;
#24795=CARTESIAN_POINT ( 'NONE',  ( -1.401094519807299710, 0.7138523880601858052, 9.927288994922816912 ) ) ;
#24799=CARTESIAN_POINT ( 'NONE',  ( -23.26005729352344176, -44.90397804740339183, 7.906207997025717304 ) ) ;
#24801=CARTESIAN_POINT ( 'NONE',  ( -4.339432828817248122, -37.24807810779213213, -8.192531242611266862 ) ) ;
#24803=CARTESIAN_POINT ( 'NONE',  ( 1.424818880982069880, -0.8247269902869861502, 9.936700280135882579 ) ) ;
#24806=ORIENTED_EDGE ( 'NONE', *, *, #31640, .T. ) ;
#24814=CARTESIAN_POINT ( 'NONE',  ( 2.053349722363697616, -0.3420258690444287208, 9.888808121373919846 ) ) ;
#24816=ORIENTED_EDGE ( 'NONE', *, *, #18593, .T. ) ;
#24818=CARTESIAN_POINT ( 'NONE',  ( 1.697332391510682159, 0.8495613812374117613, 9.900811091504543526 ) ) ;
#24820=CARTESIAN_POINT ( 'NONE',  ( -2.961022939495062900, 16.59676755884084187, 2.590526750877053086 ) ) ;
#24822=CARTESIAN_POINT ( 'NONE',  ( -22.69295089195507487, -45.31600496604688999, 7.455576670931136185 ) ) ;
#24826=CARTESIAN_POINT ( 'NONE',  ( 6.508636631827673824, 15.75743548351451295, 8.953103998512858652 ) ) ;
#24832=LINE ( 'NONE', #12771, #29119 ) ;
#24842=B_SPLINE_CURVE_WITH_KNOTS ( 'NONE', 3,
 ( #26344, #38161, #21723, #18373 ),
 .UNSPECIFIED., .F., .F.,
 ( 4, 4 ),
 ( 0.8097120833243712790, 0.9322955464061803976 ),
 .UNSPECIFIED. ) ;
#24844=CARTESIAN_POINT ( 'NONE',  ( 0.9987333403011454669, 1.123935354443737600, 9.936141075511214282 ) ) ;
#24850=CARTESIAN_POINT ( 'NONE',  ( 26.25702031264353664, -26.77347351953840615, 8.914903342594564961 ) ) ;
#24860=CARTESIAN_POINT ( 'NONE',  ( 3.087186397306452612, 2.514307945609885131, -2.642742795433417058E-16 ) ) ;
#24866=VERTEX_POINT ( 'NONE', #8059 ) ;
#24889=CARTESIAN_POINT ( 'NONE',  ( -1.365263087672800246, 0.5437404457009007430, 9.958264684458713489 ) ) ;
#24897=EDGE_CURVE ( 'NONE', #17906, #25205, #20458, .T. ) ;
#24898=EDGE_CURVE ( 'NONE', #19313, #48360, #33392, .T. ) ;
#24903=CARTESIAN_POINT ( 'NONE',  ( 18.38319608353691947, -32.68498281710168385, -8.192531242611265085 ) ) ;
#24904=B_SPLINE_CURVE_WITH_KNOTS ( 'NONE', 3,
 ( #36938, #12536, #36683, #4600, #13282, #747 ),
 .UNSPECIFIED., .F., .F.,
 ( 4, 2, 4 ),
 ( 5.818439421673296370E-18, 0.009877169331704830149, 0.01975433866340965683 ),
 .UNSPECIFIED. ) ;
#24912=CARTESIAN_POINT ( 'NONE',  ( 0.3862712429686810944, 1.188820645368943607, -10.00000000000000000 ) ) ;
#24915=CIRCLE ( 'NONE', #37208, 10.00000000000000000 ) ;
#24916=CARTESIAN_POINT ( 'NONE',  ( 0.3862712429686894766, -1.188820645368940276, -3.333333333333333481 ) ) ;
#24923=EDGE_CURVE ( 'NONE', #45889, #34658, #27838, .T. ) ;
#24958=CARTESIAN_POINT ( 'NONE',  ( 9.999999999999998224, 1.843143693225357538E-15, 8.340239149798797769 ) ) ;
#24967=CARTESIAN_POINT ( 'NONE',  ( -0.3862712429686729343, -1.188820645368946050, -3.333333333333333481 ) ) ;
#24972=EDGE_CURVE ( 'NONE', #36062, #23873, #2116, .T. ) ;
#24975=CARTESIAN_POINT ( 'NONE',  ( -8.277096487746778308, 50.00000000000000711, 7.455576670931136185 ) ) ;
#24985=CARTESIAN_POINT ( 'NONE',  ( -46.75893035013464072, -17.89420872045582200, 3.199614146704519602 ) ) ;
#24999=CARTESIAN_POINT ( 'NONE',  ( -15.57957361750255565, -5.755602074545403291, 3.266473740018926541 ) ) ;
#25005=CARTESIAN_POINT ( 'NONE',  ( 30.12518629743562926, 14.70074613238908157, 1.847720168420772691 ) ) ;
#25009=CARTESIAN_POINT ( 'NONE',  ( 14.52758583651987223, 8.922352469211173087, 8.953103998512858652 ) ) ;
#25010=CARTESIAN_POINT ( 'NONE',  ( 1.455748852897596812, 0.01196569884528948975, 9.938560165450791573 ) ) ;
#25024=EDGE_LOOP ( 'NONE', ( #48745, #22276, #20081, #50119, #12602 ) ) ;
#25033=CARTESIAN_POINT ( 'NONE',  ( -15.15373036401909346, 7.214190911381058058, -9.233365092205394475 ) ) ;
#25048=CARTESIAN_POINT ( 'NONE',  ( 8.277096487746778308, -50.00000000000000711, 7.455576670931136185 ) ) ;
#25050=VECTOR ( 'NONE', #12403, 1000.000000000000114 ) ;
#25071=ORIENTED_EDGE ( 'NONE', *, *, #38479, .F. ) ;
#25072=ORIENTED_EDGE ( 'NONE', *, *, #31825, .T. ) ;
#25073=CARTESIAN_POINT ( 'NONE',  ( 0.4611230188129936125, -1.144552435864506279, 9.969907203203808521 ) ) ;
#25074=CARTESIAN_POINT ( 'NONE',  ( 33.64889274059390090, -3.704246042440748621, 8.356839323120299312 ) ) ;
#25077=EDGE_LOOP ( 'NONE', ( #50603, #29978, #603 ) ) ;
#25088=B_SPLINE_CURVE_WITH_KNOTS ( 'NONE', 3,
 ( #45949, #11340, #26987, #2861 ),
 .UNSPECIFIED., .F., .F.,
 ( 4, 4 ),
 ( 0.000000000000000000, 0.001249001861321276038 ),
 .UNSPECIFIED. ) ;
#25103=CARTESIAN_POINT ( 'NONE',  ( 1.011271242968688311, -0.7347315653655855927, 10.00000000000000000 ) ) ;
#25107=CARTESIAN_POINT ( 'NONE',  ( -0.5113015165352315927, -1.175527691268679398, 9.948547179989621014 ) ) ;
#25116=CARTESIAN_POINT ( 'NONE',  ( 31.94178169330218964, -9.256608784833820991, -3.760136334089591248 ) ) ;
#25117=CARTESIAN_POINT ( 'NONE',  ( 23.13346437080453555, -39.73622551878964515, -8.016098858316205167 ) ) ;
#25118=CARTESIAN_POINT ( 'NONE',  ( 1.962558162476984114, -3.366505435497487042, 9.741991644047251597 ) ) ;
#25132=CARTESIAN_POINT ( 'NONE',  ( 29.18392875402930997, 17.44843138996603216, 7.906207997025717304 ) ) ;
#25137=ORIENTED_EDGE ( 'NONE', *, *, #10239, .F. ) ;
#25156=CARTESIAN_POINT ( 'NONE',  ( 19.00512336303704686, -32.33518880947659113, -8.600750091277033604 ) ) ;
#25162=CARTESIAN_POINT ( 'NONE',  ( -44.99506233596265048, -23.32283626942287569, 7.455576670931136185 ) ) ;
#25169=VERTEX_POINT ( 'NONE', #19198 ) ;
#25175=B_SPLINE_CURVE_WITH_KNOTS ( 'NONE', 3,
 ( #11273, #6650, #22552, #26404 ),
 .UNSPECIFIED., .F., .F.,
 ( 4, 4 ),
 ( 0.000000000000000000, 0.0001252128669263292060 ),
 .UNSPECIFIED. ) ;
#25182=CARTESIAN_POINT ( 'NONE',  ( -9.907356528110963012, 1.358045148327947427, 0.000000000000000000 ) ) ;
#25185=FACE_OUTER_BOUND ( 'NONE', #23678, .T. ) ;
#25189=EDGE_LOOP ( 'NONE', ( #6121, #39432, #1274, #12104 ) ) ;
#25195=B_SPLINE_SURFACE_WITH_KNOTS ( 'NONE', 3, 3, ( 
 ( #31699, #388, #16787, #8338 ),
 ( #896, #16034, #40398, #23729 ),
 ( #32448, #12180, #27835, #35814 ),
 ( #12920, #4474, #636, #43468 ) ),
 .UNSPECIFIED., .F., .F., .F.,
 ( 4, 4 ),
 ( 4, 4 ),
 ( 0.000000000000000000, 1.000000000000000000 ),
 ( 0.000000000000000000, 1.000000000000000000 ),
 .UNSPECIFIED. ) ;
#25205=VERTEX_POINT ( 'NONE', #4814 ) ;
#25210=CARTESIAN_POINT ( 'NONE',  ( -1.066995270233474624, 50.00000000000000711, -3.760136334089591248 ) ) ;
#25220=CARTESIAN_POINT ( 'NONE',  ( -1.057156451998854996, 0.7920882637787067804, 9.943883492372851407 ) ) ;
#25234=CARTESIAN_POINT ( 'NONE',  ( 17.51065725283127250, -28.41934970907778890, -9.367992836599951190 ) ) ;
#25237=EDGE_CURVE ( 'NONE', #15030, #39856, #16205, .T. ) ;
#25239=CARTESIAN_POINT ( 'NONE',  ( -0.3862712429686729343, -1.188820645368946050, -10.00000000000000000 ) ) ;
#25241=LINE ( 'NONE', #9092, #41739 ) ;
#25267=CARTESIAN_POINT ( 'NONE',  ( 29.18392875402930997, 17.44843138996603216, 7.906207997025717304 ) ) ;
#25273=CARTESIAN_POINT ( 'NONE',  ( 6.875132362119187768, -33.14667368551891258, 8.356839323120299312 ) ) ;
#25275=CARTESIAN_POINT ( 'NONE',  ( -0.8965959638259611841, -1.582931917743307215, 9.903764339332084887 ) ) ;
#25279=EDGE_CURVE ( 'NONE', #16425, #13764, #32743, .T. ) ;
#25283=CARTESIAN_POINT ( 'NONE',  ( -34.38425513258695077, 36.82177522737848108, 8.807470649214879543 ) ) ;
#25286=CARTESIAN_POINT ( 'NONE',  ( -1.589327968330880969, -0.05051906867692697312, 9.933337059263775970 ) ) ;
#25288=EDGE_CURVE ( 'NONE', #50205, #5524, #11934, .T. ) ;
#25292=CARTESIAN_POINT ( 'NONE',  ( 1.540662627795932105, -1.371465786296032441, 9.894754715216729224 ) ) ;
#25294=CARTESIAN_POINT ( 'NONE',  ( -1.011271242968688533, 0.7347315653655859258, 10.00000000000000000 ) ) ;
#25295=EDGE_CURVE ( 'NONE', #9096, #11140, #21098, .T. ) ;
#25297=CARTESIAN_POINT ( 'NONE',  ( -47.22310614333779455, -16.46562252335923660, -3.760136334089591248 ) ) ;
#25298=FACE_OUTER_BOUND ( 'NONE', #26278, .T. ) ;
#25299=CARTESIAN_POINT ( 'NONE',  ( -1.011271242968677875, -0.7347315653656004697, 10.00000000000000000 ) ) ;
#25302=EDGE_LOOP ( 'NONE', ( #11915, #46858, #50187, #13386, #29919, #4569, #6402, #19807, #37860, #8426, #38089, #49371, #34185, #28297 ) ) ;
#25304=B_SPLINE_SURFACE_WITH_KNOTS ( 'NONE', 3, 3, ( 
 ( #5795, #44267, #12735, #25294 ),
 ( #9139, #40951, #37123, #13486 ),
 ( #24799, #40451, #20943, #32750 ),
 ( #48344, #13232, #28894, #29393 ) ),
 .UNSPECIFIED., .F., .F., .F.,
 ( 4, 4 ),
 ( 4, 4 ),
 ( 0.000000000000000000, 1.000000000000000000 ),
 ( 0.000000000000000000, 1.000000000000000000 ),
 .UNSPECIFIED. ) ;
#25311=CARTESIAN_POINT ( 'NONE',  ( -0.4166666666666669072, 0.000000000000000000, 10.00000000000000000 ) ) ;
#25319=CARTESIAN_POINT ( 'NONE',  ( 0.2834763335391893846, -1.876787935832544107, 9.900811091504525763 ) ) ;
#25321=AXIS2_PLACEMENT_3D ( 'NONE', #39758, #24601, #40250 ) ;
#25331=CARTESIAN_POINT ( 'NONE',  ( -1.275994128725546739, 0.1230186051320636409, 9.948547179989615685 ) ) ;
#25332=ORIENTED_EDGE ( 'NONE', *, *, #1054, .F. ) ;
#25334=CARTESIAN_POINT ( 'NONE',  ( -45.64490844644706158, -21.32281559348763977, 8.807470649214879543 ) ) ;
#25335=CARTESIAN_POINT ( 'NONE',  ( -0.4266413953668892756, -1.250184266969579294, 9.943883492372849631 ) ) ;
#25337=CARTESIAN_POINT ( 'NONE',  ( -1.275994128725546739, 0.1230186051320636409, 9.948547179989615685 ) ) ;
#25340=CARTESIAN_POINT ( 'NONE',  ( 31.46770792452135268, -38.94077080897339727, 3.199614146704519602 ) ) ;
#25382=B_SPLINE_CURVE_WITH_KNOTS ( 'NONE', 3,
 ( #6503, #22160, #2403, #17804 ),
 .UNSPECIFIED., .F., .F.,
 ( 4, 4 ),
 ( 0.01012863361515542113, 0.01015667504234211808 ),
 .UNSPECIFIED. ) ;
#25397=FACE_OUTER_BOUND ( 'NONE', #12149, .T. ) ;
#25401=CARTESIAN_POINT ( 'NONE',  ( 0.9602803029231544718, -0.8490247040095941777, 9.976582533991681601 ) ) ;
#25402=CARTESIAN_POINT ( 'NONE',  ( 1.151763129092702398, -0.4096856258255446304, 9.987567862361071747 ) ) ;
#25405=CARTESIAN_POINT ( 'NONE',  ( 0.3862712429686894766, -1.188820645368940276, -3.333333333333333481 ) ) ;
#25411=CARTESIAN_POINT ( 'NONE',  ( -28.96803024440907137, -18.11533787072017176, 7.455576670931136185 ) ) ;
#25416=CARTESIAN_POINT ( 'NONE',  ( -44.99506233596265048, -23.32283626942287569, 7.455576670931136185 ) ) ;
#25417=CARTESIAN_POINT ( 'NONE',  ( -0.3862712429686895876, 1.188820645368940720, 10.00000000000000000 ) ) ;
#25421=EDGE_LOOP ( 'NONE', ( #35104, #21322, #4120, #44853 ) ) ;
#25422=FACE_OUTER_BOUND ( 'NONE', #40779, .T. ) ;
#25434=CARTESIAN_POINT ( 'NONE',  ( 0.9390173899407876501, 1.130417317737878458, 9.958264684458711713 ) ) ;
#25436=CARTESIAN_POINT ( 'NONE',  ( -0.4384710792283267322, -1.388197036929783357, 9.938560165450807560 ) ) ;
#25441=ORIENTED_EDGE ( 'NONE', *, *, #25495, .F. ) ;
#25446=B_SPLINE_CURVE_WITH_KNOTS ( 'NONE', 3,
 ( #26007, #22899, #27005, #14958 ),
 .UNSPECIFIED., .F., .F.,
 ( 4, 4 ),
 ( 1.734723475976807094E-18, 8.326314924664821488E-06 ),
 .UNSPECIFIED. ) ;
#25447=CARTESIAN_POINT ( 'NONE',  ( -22.90865447854277193, -29.73489050103202302, -2.490396854064185650 ) ) ;
#25448=CARTESIAN_POINT ( 'NONE',  ( 40.76831105797779031, 21.94948152812829889, 7.455576670931137073 ) ) ;
#25452=ORIENTED_EDGE ( 'NONE', *, *, #10948, .F. ) ;
#25457=ORIENTED_EDGE ( 'NONE', *, *, #36929, .F. ) ;
#25460=CARTESIAN_POINT ( 'NONE',  ( -3.694521163055078272, -0.7694713829383514891, 9.865049507598754985 ) ) ;
#25463=CARTESIAN_POINT ( 'NONE',  ( -1.158497635116737312, 16.61944452314319420, -3.546734833711462365 ) ) ;
#25470=CARTESIAN_POINT ( 'NONE',  ( 1.377509002708426689, -0.6027468487254984408, 9.927319414211227766 ) ) ;
#25480=CARTESIAN_POINT ( 'NONE',  ( 34.08355720199905647, -2.371364769369109116, 7.455576670931136185 ) ) ;
#25482=CARTESIAN_POINT ( 'NONE',  ( -1.011271242968688533, 0.7347315653655859258, -3.333333333333333481 ) ) ;
#25487=CARTESIAN_POINT ( 'NONE',  ( 46.55190821232867648, -18.53135734581217164, -8.917361510505369182 ) ) ;
#25490=CARTESIAN_POINT ( 'NONE',  ( 0.000000000000000000, 0.000000000000000000, 0.000000000000000000 ) ) ;
#25491=ADVANCED_FACE ( 'NONE', ( #14282 ), #29947, .F. ) ;
#25495=EDGE_CURVE ( 'NONE', #48161, #13105, #29687, .T. ) ;
#25496=CARTESIAN_POINT ( 'NONE',  ( 28.96803024440893992, 18.11533787072037072, 7.455576670931136185 ) ) ;
#25517=VERTEX_POINT ( 'NONE', #15050 ) ;
#25518=ADVANCED_FACE ( 'NONE', ( #37662 ), #3954, .T. ) ;
#25521=CARTESIAN_POINT ( 'NONE',  ( -4.353119224255007857, -9.002796955359011477, 0.000000000000000000 ) ) ;
#25524=CARTESIAN_POINT ( 'NONE',  ( -7.574282714737721633, 6.549555713337947616, 3.092310436554648767 ) ) ;
#25532=ADVANCED_FACE ( 'NONE', ( #16322 ), #8893, .T. ) ;
#25542=CARTESIAN_POINT ( 'NONE',  ( 7.576114424932982594, -33.14742743729794938, 7.906207997025717304 ) ) ;
#25547=ORIENTED_EDGE ( 'NONE', *, *, #32103, .T. ) ;
#25551=FACE_OUTER_BOUND ( 'NONE', #6517, .T. ) ;
#25556=ORIENTED_EDGE ( 'NONE', *, *, #2087, .F. ) ;
#25573=CARTESIAN_POINT ( 'NONE',  ( 5.888214538810389698, 16.20866436362417673, 8.727788335465566760 ) ) ;
#25578=CARTESIAN_POINT ( 'NONE',  ( 7.749480817862238524, 14.85497772329518895, 9.403735324607438884 ) ) ;
#25589=EDGE_CURVE ( 'NONE', #47273, #30921, #35343, .T. ) ;
#25591=EDGE_CURVE ( 'NONE', #37300, #2701, #41812, .T. ) ;
#25595=CARTESIAN_POINT ( 'NONE',  ( 20.37409433807990666, 26.28007012093483397, -2.408242355805840784 ) ) ;
#25601=DIRECTION ( 'NONE',  ( -0.8090169943749507819, 0.5877852522924685852, 0.000000000000000000 ) ) ;
#25620=ORIENTED_EDGE ( 'NONE', *, *, #8595, .T. ) ;
#25622=B_SPLINE_SURFACE_WITH_KNOTS ( 'NONE', 3, 3, ( 
 ( #46662, #23605, #26947, #19236 ),
 ( #3333, #34927, #4110, #18 ),
 ( #19491, #11815, #47170, #11561 ),
 ( #50501, #30811, #18983, #46415 ) ),
 .UNSPECIFIED., .F., .F., .F.,
 ( 4, 4 ),
 ( 4, 4 ),
 ( 0.000000000000000000, 1.000000000000000000 ),
 ( 0.000000000000000000, 1.000000000000000000 ),
 .UNSPECIFIED. ) ;
#25625=CARTESIAN_POINT ( 'NONE',  ( -4.632259510536085756, 3.749670975867693379, -2.642742795433417058E-16 ) ) ;
#25626=ORIENTED_EDGE ( 'NONE', *, *, #24264, .F. ) ;
#25645=EDGE_LOOP ( 'NONE', ( #270, #32615, #12598, #44602 ) ) ;
#25649=ORIENTED_EDGE ( 'NONE', *, *, #25237, .F. ) ;
#25653=CARTESIAN_POINT ( 'NONE',  ( 25.60949810002064098, 43.19700938445193827, 1.847720168420772691 ) ) ;
#25660=CARTESIAN_POINT ( 'NONE',  ( -0.8285222815141961572, -1.889008401827320771, 9.886433018048073507 ) ) ;
#25662=CARTESIAN_POINT ( 'NONE',  ( 0.3862712429686894766, -1.188820645368940276, 3.333333333333333481 ) ) ;
#25667=CARTESIAN_POINT ( 'NONE',  ( -1.011271242968677875, -0.7347315653656004697, 10.00000000000000000 ) ) ;
#25669=CARTESIAN_POINT ( 'NONE',  ( -1.962558162477761714, 3.366505435501197407, 9.741991644046970933 ) ) ;
#25673=CARTESIAN_POINT ( 'NONE',  ( 12.78770032058947237, 31.68259716188277864, 7.455576670931136185 ) ) ;
#25675=CARTESIAN_POINT ( 'NONE',  ( -46.10908423965022251, -19.89422939639105437, 1.847720168420772691 ) ) ;
#25680=CARTESIAN_POINT ( 'NONE',  ( -1.249999999999999778, 0.000000000000000000, 10.00000000000000000 ) ) ;
#25682=B_SPLINE_CURVE_WITH_KNOTS ( 'NONE', 3,
 ( #18487, #18953, #42559, #34635, #3561, #50209 ),
 .UNSPECIFIED., .F., .F.,
 ( 4, 2, 4 ),
 ( 5.818439421673296370E-18, 0.009877169331704830149, 0.01975433866340965683 ),
 .UNSPECIFIED. ) ;
#25690=ORIENTED_EDGE ( 'NONE', *, *, #4635, .T. ) ;
#25692=CARTESIAN_POINT ( 'NONE',  ( -0.4402948852767746279, 2.015117899693936732, 9.894754715216722118 ) ) ;
#25696=ORIENTED_EDGE ( 'NONE', *, *, #44301, .F. ) ;
#25706=ORIENTED_EDGE ( 'NONE', *, *, #11712, .F. ) ;
#25737=B_SPLINE_SURFACE_WITH_KNOTS ( 'NONE', 3, 3, ( 
 ( #1137, #20622, #16773, #32438 ),
 ( #2618, #17529, #5976, #6478 ),
 ( #29836, #9579, #21890, #32949 ),
 ( #37057, #25480, #33943, #49531 ) ),
 .UNSPECIFIED., .F., .F., .F.,
 ( 4, 4 ),
 ( 4, 4 ),
 ( 0.000000000000000000, 1.000000000000000000 ),
 ( 0.000000000000000000, 1.000000000000000000 ),
 .UNSPECIFIED. ) ;
#25742=CARTESIAN_POINT ( 'NONE',  ( -46.76852358249001895, 17.86468378716740801, -9.367992836599951190 ) ) ;
#25743=ORIENTED_EDGE ( 'NONE', *, *, #42446, .F. ) ;
#25747=CARTESIAN_POINT ( 'NONE',  ( 15.15373036401913787, -7.214190911380954141, -9.233365092205394475 ) ) ;
#25748=ORIENTED_EDGE ( 'NONE', *, *, #1117, .F. ) ;
#25750=CARTESIAN_POINT ( 'NONE',  ( 33.14391172085757375, 37.72293746533119929, -8.016098858316199838 ) ) ;
#25756=CARTESIAN_POINT ( 'NONE',  ( -30.64276258327282321, -34.28040101195678346, -8.016098858316205167 ) ) ;
#25758=CARTESIAN_POINT ( 'NONE',  ( 14.86945752723346637, 7.944783388879009145, 2.590526750877053086 ) ) ;
#25759=EDGE_CURVE ( 'NONE', #23523, #13148, #21009, .T. ) ;
#25792=CARTESIAN_POINT ( 'NONE',  ( -24.47767542868268364, 23.18653802921800278, 8.807470649214879543 ) ) ;
#25795=CARTESIAN_POINT ( 'NONE',  ( 36.08557433729230013, -35.58569447144767395, 7.455576670931136185 ) ) ;
#25797=CARTESIAN_POINT ( 'NONE',  ( -1.249999999999999778, 0.000000000000000000, 10.00000000000000000 ) ) ;
#25799=FACE_OUTER_BOUND ( 'NONE', #38226, .T. ) ;
#25804=CARTESIAN_POINT ( 'NONE',  ( 21.61731705588930552, 25.43568671410602278, -9.367992836599951190 ) ) ;
#25806=CARTESIAN_POINT ( 'NONE',  ( -28.96803024440907137, -18.11533787072017176, 7.455576670931136185 ) ) ;
#25811=VERTEX_POINT ( 'NONE', #6022 ) ;
#25820=CARTESIAN_POINT ( 'NONE',  ( 3.229232847726260403, -16.57333684275945629, 9.178419661560148768 ) ) ;
#25825=ORIENTED_EDGE ( 'NONE', *, *, #27233, .T. ) ;
#25831=CARTESIAN_POINT ( 'NONE',  ( -10.00000000000000000, 0.000000000000000000, 10.00000000000000000 ) ) ;
#25837=CARTESIAN_POINT ( 'NONE',  ( -0.3862712429686809279, -1.188820645368943163, 10.00000000000000000 ) ) ;
#25858=CARTESIAN_POINT ( 'NONE',  ( 0.9989200098981507736, 1.123829893718967687, 9.927319414211233095 ) ) ;
#25869=CARTESIAN_POINT ( 'NONE',  ( 7.726417830024686850, -6.396462539501553302, 9.390253821402620105 ) ) ;
#25873=CARTESIAN_POINT ( 'NONE',  ( -0.4401267517937272333, 2.015194695084603360, 9.889206916986893248 ) ) ;
#25897=ORIENTED_EDGE ( 'NONE', *, *, #50101, .T. ) ;
#25898=B_SPLINE_CURVE_WITH_KNOTS ( 'NONE', 3,
 ( #43114, #47425, #8738, #12074 ),
 .UNSPECIFIED., .F., .F.,
 ( 4, 4 ),
 ( 1.580408300606902237E-17, 0.009404495247862305896 ),
 .UNSPECIFIED. ) ;
#25909=CARTESIAN_POINT ( 'NONE',  ( -4.672045878990125800, 50.00000000000000711, 1.847720168420772691 ) ) ;
#25910=CARTESIAN_POINT ( 'NONE',  ( 1.275949648750062337, -0.1226307170719979495, 9.967237415621765351 ) ) ;
#25912=ADVANCED_FACE ( 'NONE', ( #4460 ), #28152, .T. ) ;
#25921=CARTESIAN_POINT ( 'NONE',  ( -2.948105490345101387, -9.555557232197246620, 9.282506307616472441 ) ) ;
#25924=CARTESIAN_POINT ( 'NONE',  ( 1.320835335343329753, -0.01943189459118491516, 9.943883492372847854 ) ) ;
#25939=VECTOR ( 'NONE', #33871, 1000.000000000000000 ) ;
#25946=EDGE_CURVE ( 'NONE', #31529, #26571, #26554, .T. ) ;
#25954=CARTESIAN_POINT ( 'NONE',  ( 0.000000000000000000, 0.000000000000000000, 0.000000000000000000 ) ) ;
#25969=CARTESIAN_POINT ( 'NONE',  ( 0.4166666666666664631, 0.000000000000000000, 10.00000000000000000 ) ) ;
#25970=CARTESIAN_POINT ( 'NONE',  ( -1.148889881503118993, -0.6106841242179669171, 9.986087673579197244 ) ) ;
#25973=CARTESIAN_POINT ( 'NONE',  ( 1.721971274562253740, 0.09408549481334846365, 9.928159647716247704 ) ) ;
#25990=CARTESIAN_POINT ( 'NONE',  ( -3.231548175622898089, 9.463461120997347820, 9.282506307616472441 ) ) ;
#25992=CARTESIAN_POINT ( 'NONE',  ( 0.9306608372802014362, 1.429911642202264854, 9.912103175172944702 ) ) ;
#25997=LINE ( 'NONE', #25742, #18781 ) ;
#26005=CARTESIAN_POINT ( 'NONE',  ( 30.43621780902783058, -14.03210827430559249, -8.466730184410787174 ) ) ;
#26007=CARTESIAN_POINT ( 'NONE',  ( -1.780432407520014415, -1.041450996408466612, 9.894754715216725671 ) ) ;
#26037=VERTEX_POINT ( 'NONE', #32942 ) ;
#26045=B_SPLINE_SURFACE_WITH_KNOTS ( 'NONE', 3, 3, ( 
 ( #26119, #29987, #45601, #10476 ),
 ( #28968, #9466, #40775, #44582 ),
 ( #41770, #25132, #21269, #36957 ),
 ( #1777, #7401, #10983, #6883 ) ),
 .UNSPECIFIED., .F., .F., .F.,
 ( 4, 4 ),
 ( 4, 4 ),
 ( 0.000000000000000000, 1.000000000000000000 ),
 ( 0.000000000000000000, 1.000000000000000000 ),
 .UNSPECIFIED. ) ;
#26046=CARTESIAN_POINT ( 'NONE',  ( -11.73320209285699889, 11.96063479729179768, 9.403735324607438884 ) ) ;
#26049=CARTESIAN_POINT ( 'NONE',  ( -1.632255792517811388, 3.624924591517729056, 3.247138655587492817 ) ) ;
#26054=CARTESIAN_POINT ( 'NONE',  ( 46.75893035013449861, 17.89420872045614885, 3.199614146704519602 ) ) ;
#26057=CARTESIAN_POINT ( 'NONE',  ( -31.28234235046239320, -11.28615439405757392, -3.760136334089591248 ) ) ;
#26058=CARTESIAN_POINT ( 'NONE',  ( -25.60949810002096783, -43.19700938445173932, 1.847720168420772691 ) ) ;
#26060=CARTESIAN_POINT ( 'NONE',  ( 37.27397286063867199, -4.111076158911552092, 7.697694107796188234 ) ) ;
#26063=CARTESIAN_POINT ( 'NONE',  ( 1.250000000000000222, 0.000000000000000000, 3.333333333333333481 ) ) ;
#26066=CARTESIAN_POINT ( 'NONE',  ( 0.4166666666666664631, 0.000000000000000000, 10.00000000000000000 ) ) ;
#26070=EDGE_CURVE ( 'NONE', #23873, #37300, #44790, .T. ) ;
#26073=CARTESIAN_POINT ( 'NONE',  ( -0.1287570809895576818, -0.3962735484563154609, 10.00000000000000000 ) ) ;
#26089=DIRECTION ( 'NONE',  ( 0.9510565162951545304, -0.3090169943749447312, 0.000000000000000000 ) ) ;
#26093=CARTESIAN_POINT ( 'NONE',  ( -36.44255557191976180, -8.993813888722101524, -5.338708898921616708 ) ) ;
#26094=CARTESIAN_POINT ( 'NONE',  ( -1.011271242968683426, -0.7347315653655928092, 10.00000000000000000 ) ) ;
#26102=CARTESIAN_POINT ( 'NONE',  ( -1.841312257079161796, -1.034875951311538422, 9.884520316594374023 ) ) ;
#26119=CARTESIAN_POINT ( 'NONE',  ( 45.64490844644691236, 21.32281559348795952, 8.807470649214879543 ) ) ;
#26128=CARTESIAN_POINT ( 'NONE',  ( 12.35406723005396046, -11.51001571518080624, 9.178419661560148768 ) ) ;
#26142=B_SPLINE_SURFACE_WITH_KNOTS ( 'NONE', 3, 3, ( 
 ( #19008, #34693, #26975, #42611 ),
 ( #38793, #3620, #19267, #50523 ),
 ( #47691, #8502, #27741, #23632 ),
 ( #23889, #43372, #31855, #32353 ) ),
 .UNSPECIFIED., .F., .F., .F.,
 ( 4, 4 ),
 ( 4, 4 ),
 ( 0.000000000000000000, 1.000000000000000000 ),
 ( 0.000000000000000000, 1.000000000000000000 ),
 .UNSPECIFIED. ) ;
#26147=B_SPLINE_CURVE_WITH_KNOTS ( 'NONE', 3,
 ( #15773, #142, #31707, #12428 ),
 .UNSPECIFIED., .F., .F.,
 ( 4, 4 ),
 ( 0.003198294599461561517, 0.003311263741940095786 ),
 .UNSPECIFIED. ) ;
#26149=ORIENTED_EDGE ( 'NONE', *, *, #44632, .T. ) ;
#26155=VERTEX_POINT ( 'NONE', #6722 ) ;
#26185=EDGE_CURVE ( 'NONE', #40610, #28209, #15458, .T. ) ;
#26193=CARTESIAN_POINT ( 'NONE',  ( -26.18032376592659105, 21.95228666728381128, 7.455576670931136185 ) ) ;
#26200=B_SPLINE_CURVE_WITH_KNOTS ( 'NONE', 3,
 ( #13330, #17442, #44604, #9485 ),
 .UNSPECIFIED., .F., .F.,
 ( 4, 4 ),
 ( 5.641302087948371272E-05, 0.0003272669002642206951 ),
 .UNSPECIFIED. ) ;
#26207=ORIENTED_EDGE ( 'NONE', *, *, #29267, .T. ) ;
#26211=ORIENTED_EDGE ( 'NONE', *, *, #11245, .F. ) ;
#26214=CARTESIAN_POINT ( 'NONE',  ( 25.04522487443081502, -22.77512090857307925, 8.356839323120299312 ) ) ;
#26222=CARTESIAN_POINT ( 'NONE',  ( 23.29043492822826167, -24.10797434788167948, 1.847720168420772691 ) ) ;
#26228=CARTESIAN_POINT ( 'NONE',  ( -23.26005729352344176, -44.90397804740339183, 7.906207997025717304 ) ) ;
#26232=CARTESIAN_POINT ( 'NONE',  ( 0.5391758413130712801, -1.495929470048738663, 9.933337059263825708 ) ) ;
#26233=CARTESIAN_POINT ( 'NONE',  ( 2.210477865340801706, 37.43479381012853224, -9.422646554964178023 ) ) ;
#26237=CARTESIAN_POINT ( 'NONE',  ( -9.907356528110963012, 1.358045148327947427, 0.000000000000000000 ) ) ;
#26253=CARTESIAN_POINT ( 'NONE',  ( 27.33593271309472073, -41.94268121623323964, -9.367992836599951190 ) ) ;
#26256=B_SPLINE_CURVE_WITH_KNOTS ( 'NONE', 3,
 ( #2572, #17965, #41082, #6430, #37755, #13624 ),
 .UNSPECIFIED., .F., .F.,
 ( 4, 2, 4 ),
 ( 7.757919228897728493E-18, 0.009877169331704830149, 0.01975433866340965336 ),
 .UNSPECIFIED. ) ;
#26278=EDGE_LOOP ( 'NONE', ( #24068, #37005, #43413 ) ) ;
#26286=CARTESIAN_POINT ( 'NONE',  ( -3.414233368894360243, -9.411746240900615845, 6.185594734181532495 ) ) ;
#26296=EDGE_LOOP ( 'NONE', ( #28197, #17262, #35767 ) ) ;
#26297=CARTESIAN_POINT ( 'NONE',  ( 0.000000000000000000, 0.000000000000000000, 0.000000000000000000 ) ) ;
#26301=B_SPLINE_CURVE_WITH_KNOTS ( 'NONE', 3,
 ( #28642, #5295, #20952, #40957 ),
 .UNSPECIFIED., .F., .F.,
 ( 4, 4 ),
 ( 0.001403500796105015260, 0.001586656765099046058 ),
 .UNSPECIFIED. ) ;
#26309=CARTESIAN_POINT ( 'NONE',  ( 15.00099850811936264, 7.462898891544210933, 9.403735324607438884 ) ) ;
#26315=CARTESIAN_POINT ( 'NONE',  ( 26.18032376592674737, -21.95228666728361233, 7.455576670931136185 ) ) ;
#26320=VERTEX_POINT ( 'NONE', #15686 ) ;
#26321=CARTESIAN_POINT ( 'NONE',  ( -2.569099690548740877, 33.19126772784019153, 3.199614146704519602 ) ) ;
#26322=CARTESIAN_POINT ( 'NONE',  ( 1.780494907546722461, 1.041382914740401011, 9.891980816076523908 ) ) ;
#26328=VERTEX_POINT ( 'NONE', #15187 ) ;
#26332=CARTESIAN_POINT ( 'NONE',  ( -9.696760411816217839, -2.443938934554997999, 0.000000000000000000 ) ) ;
#26344=CARTESIAN_POINT ( 'NONE',  ( 2.948105490344985480, 9.555557232197198658, 9.282506307616484875 ) ) ;
#26360=CARTESIAN_POINT ( 'NONE',  ( -3.808200756227646089, -0.8261963378076270237, 9.741991644047246268 ) ) ;
#26363=CARTESIAN_POINT ( 'NONE',  ( 6.174150299305392053, -33.14591993373988998, 8.807470649214879543 ) ) ;
#26368=CARTESIAN_POINT ( 'NONE',  ( -1.962712821592842882, -1.022159834731130257, 9.881002359080275355 ) ) ;
#26373=CARTESIAN_POINT ( 'NONE',  ( 18.38319608353691947, -32.68498281710168385, -8.192531242611265085 ) ) ;
#26397=CARTESIAN_POINT ( 'NONE',  ( -1.249999999999999778, 0.000000000000000000, 10.00000000000000000 ) ) ;
#26404=CARTESIAN_POINT ( 'NONE',  ( 1.011271242968683648, 0.7347315653655930312, 9.972675548442463622 ) ) ;
#26412=CARTESIAN_POINT ( 'NONE',  ( 1.315487699543018918, -0.8933127557395131868, 9.933337059263825708 ) ) ;
#26414=CARTESIAN_POINT ( 'NONE',  ( 0.3370904143228981575, -0.2449105217885261532, 10.00000000000000000 ) ) ;
#26421=B_SPLINE_CURVE_WITH_KNOTS ( 'NONE', 3,
 ( #39754, #28888, #31300, #47140 ),
 .UNSPECIFIED., .F., .F.,
 ( 4, 4 ),
 ( 0.0009539133080775338879, 0.009404495247862345794 ),
 .UNSPECIFIED. ) ;
#26428=ORIENTED_EDGE ( 'NONE', *, *, #30180, .T. ) ;
#26444=CARTESIAN_POINT ( 'NONE',  ( -33.64889274059387958, 3.704246042440976439, 8.356839323120299312 ) ) ;
#26451=DIRECTION ( 'NONE',  ( -0.000000000000000000, 0.000000000000000000, -1.000000000000000000 ) ) ;
#26457=EDGE_LOOP ( 'NONE', ( #11552, #16164, #10059, #44710 ) ) ;
#26462=CARTESIAN_POINT ( 'NONE',  ( -1.540526284687967706, 1.371707213411501147, 9.886433018048069954 ) ) ;
#26464=CARTESIAN_POINT ( 'NONE',  ( -7.129058724845069861, -15.30620660340479766, 9.178419661560148768 ) ) ;
#26465=CARTESIAN_POINT ( 'NONE',  ( -25.61277432017861955, 22.36370378792854297, 7.906207997025717304 ) ) ;
#26467=CARTESIAN_POINT ( 'NONE',  ( -0.3656201545664206076, 2.182515578491385000, 9.881002359080270026 ) ) ;
#26490=ORIENTED_EDGE ( 'NONE', *, *, #46294, .T. ) ;
#26492=CARTESIAN_POINT ( 'NONE',  ( 14.48769039275578407, 30.44468701195595983, 8.807470649214879543 ) ) ;
#26498=CARTESIAN_POINT ( 'NONE',  ( -1.377636575563021992, 0.6021164824561227036, 9.953784399990620813 ) ) ;
#26500=CARTESIAN_POINT ( 'NONE',  ( -0.3862712429686977478, 1.188820645368937390, 10.00000000000000000 ) ) ;
#26509=EDGE_CURVE ( 'NONE', #27159, #13148, #27100, .T. ) ;
#26526=CARTESIAN_POINT ( 'NONE',  ( 2.961022939495062900, -16.59676755884084187, 2.590526750877053086 ) ) ;
#26530=CARTESIAN_POINT ( 'NONE',  ( -14.76429217231967428, -8.192625680377590314, 9.178419661560148768 ) ) ;
#26531=ORIENTED_EDGE ( 'NONE', *, *, #46224, .T. ) ;
#26532=CARTESIAN_POINT ( 'NONE',  ( 0.8738110990266874101, 1.684976543153885453, 9.900811091504547079 ) ) ;
#26533=ORIENTED_EDGE ( 'NONE', *, *, #19699, .F. ) ;
#26537=CARTESIAN_POINT ( 'NONE',  ( -12.35406723005387875, 11.51001571518090039, 9.178419661560148768 ) ) ;
#26548=CARTESIAN_POINT ( 'NONE',  ( 31.44259251615245176, 38.95901822126168668, -9.367992836599951190 ) ) ;
#26550=CARTESIAN_POINT ( 'NONE',  ( -49.67735855322972327, 8.912210285362091255, 8.356839323120299312 ) ) ;
#26554=B_SPLINE_CURVE_WITH_KNOTS ( 'NONE', 3,
 ( #42431, #31682, #4213, #50345 ),
 .UNSPECIFIED., .F., .F.,
 ( 4, 4 ),
 ( 0.000000000000000000, 0.0002520763768929632940 ),
 .UNSPECIFIED. ) ;
#26561=CARTESIAN_POINT ( 'NONE',  ( 1.011271242968677653, 0.7347315653656002477, 3.333333333333333481 ) ) ;
#26571=VERTEX_POINT ( 'NONE', #18908 ) ;
#26578=ORIENTED_EDGE ( 'NONE', *, *, #11170, .T. ) ;
#26594=EDGE_CURVE ( 'NONE', #48164, #48573, #13641, .T. ) ;
#26599=CARTESIAN_POINT ( 'NONE',  ( -0.3862712429686977478, 1.188820645368937390, -10.00000000000000000 ) ) ;
#26605=CARTESIAN_POINT ( 'NONE',  ( -1.011271242968677875, -0.7347315653656004697, 10.00000000000000000 ) ) ;
#26607=CARTESIAN_POINT ( 'NONE',  ( 1.057156451998911839, -0.7920882637786250680, 9.943883492372851407 ) ) ;
#26614=CARTESIAN_POINT ( 'NONE',  ( -2.462075149652696027, 16.57295996686994499, 9.403735324607438884 ) ) ;
#26616=EDGE_CURVE ( 'NONE', #36948, #1440, #29544, .T. ) ;
#26629=ORIENTED_EDGE ( 'NONE', *, *, #16468, .T. ) ;
#26639=B_SPLINE_CURVE_WITH_KNOTS ( 'NONE', 3,
 ( #49020, #6725, #10075, #33445 ),
 .UNSPECIFIED., .F., .F.,
 ( 4, 4 ),
 ( 8.940560153363745023E-19, 0.0003726843654217072417 ),
 .UNSPECIFIED. ) ;
#26656=EDGE_CURVE ( 'NONE', #4452, #31279, #42352, .T. ) ;
#26657=CARTESIAN_POINT ( 'NONE',  ( 25.60949810002064098, 43.19700938445193827, 1.847720168420772691 ) ) ;
#26677=CARTESIAN_POINT ( 'NONE',  ( -9.221081804193374865, -13.81382350053984176, 3.266473740018926541 ) ) ;
#26687=CARTESIAN_POINT ( 'NONE',  ( 16.52264463346132572, -2.779753662172757878, 9.403735324607438884 ) ) ;
#26698=CARTESIAN_POINT ( 'NONE',  ( -0.9390173899430289683, -1.130417317737636651, 9.958264684458541183 ) ) ;
#26710=CARTESIAN_POINT ( 'NONE',  ( -47.55282581475762527, -15.45084971874758217, 0.000000000000000000 ) ) ;
#26719=ORIENTED_EDGE ( 'NONE', *, *, #21814, .T. ) ;
#26723=CARTESIAN_POINT ( 'NONE',  ( 0.5113015165352333691, 1.175527691268683395, 9.948547179989619238 ) ) ;
#26726=ORIENTED_EDGE ( 'NONE', *, *, #12037, .F. ) ;
#26732=ADVANCED_FACE ( 'NONE', ( #28148 ), #12234, .F. ) ;
#26737=CARTESIAN_POINT ( 'NONE',  ( 1.962558162476984114, -3.366505435497487042, 9.741991644047251597 ) ) ;
#26743=CARTESIAN_POINT ( 'NONE',  ( 49.46074318306830975, -9.578883844006833570, 8.807470649214879543 ) ) ;
#26744=CARTESIAN_POINT ( 'NONE',  ( 1.057156451998911839, -0.7920882637786250680, 9.943883492372851407 ) ) ;
#26758=CARTESIAN_POINT ( 'NONE',  ( 1.873480598308087330, -3.275918692700725110, 9.865049507598753209 ) ) ;
#26764=CARTESIAN_POINT ( 'NONE',  ( -5.297167662385172449, -5.958617466648796324, 3.455894424797545383E-16 ) ) ;
#26765=CARTESIAN_POINT ( 'NONE',  ( 0.000000000000000000, 0.000000000000000000, 0.000000000000000000 ) ) ;
#26774=CARTESIAN_POINT ( 'NONE',  ( -1.224837355095377500, -1.100071488488243876, 9.927568724237806563 ) ) ;
#26785=ORIENTED_EDGE ( 'NONE', *, *, #11371, .T. ) ;
#26790=CARTESIAN_POINT ( 'NONE',  ( -1.320835335343009787, 0.01943189458965158267, 9.943883492372876276 ) ) ;
#26794=CARTESIAN_POINT ( 'NONE',  ( -12.97493236725075683, 11.05939663307000664, 8.953103998512858652 ) ) ;
#26800=ORIENTED_EDGE ( 'NONE', *, *, #27225, .T. ) ;
#26810=CARTESIAN_POINT ( 'NONE',  ( -29.61572577327014955, -16.11461842845715253, 8.807470649214879543 ) ) ;
#26816=ORIENTED_EDGE ( 'NONE', *, *, #28846, .T. ) ;
#26823=CARTESIAN_POINT ( 'NONE',  ( -8.277096487746778308, 33.14818118907697198, 7.455576670931136185 ) ) ;
#26829=CARTESIAN_POINT ( 'NONE',  ( 15.00099850811936264, 7.462898891544210933, 9.403735324607438884 ) ) ;
#26835=CARTESIAN_POINT ( 'NONE',  ( -49.67735855322972327, 8.912210285362091255, 8.356839323120299312 ) ) ;
#26845=CARTESIAN_POINT ( 'NONE',  ( 3.414233368894302068, 9.411746240900633609, 6.185594734181435683 ) ) ;
#26846=VERTEX_POINT ( 'NONE', #10409 ) ;
#26853=CARTESIAN_POINT ( 'NONE',  ( -1.142975459103954705, -16.61830776097024653, -2.870787844569587133 ) ) ;
#26854=ORIENTED_EDGE ( 'NONE', *, *, #49601, .T. ) ;
#26863=FACE_OUTER_BOUND ( 'NONE', #43935, .T. ) ;
#26866=CARTESIAN_POINT ( 'NONE',  ( 1.468713901642212161, 0.3220470327672588229, 9.927319414211225990 ) ) ;
#26876=CARTESIAN_POINT ( 'NONE',  ( -0.1475726264153620626, -1.496347932843211215, 9.927319414211227766 ) ) ;
#26877=EDGE_CURVE ( 'NONE', #14899, #3733, #36842, .T. ) ;
#26879=B_SPLINE_SURFACE_WITH_KNOTS ( 'NONE', 3, 3, ( 
 ( #47791, #28337, #43969, #36310 ),
 ( #13687, #6258, #9344, #44465 ),
 ( #14178, #40892, #29592, #29851 ),
 ( #9593, #28841, #37328, #17291 ) ),
 .UNSPECIFIED., .F., .F., .F.,
 ( 4, 4 ),
 ( 4, 4 ),
 ( 0.000000000000000000, 1.000000000000000000 ),
 ( 0.000000000000000000, 1.000000000000000000 ),
 .UNSPECIFIED. ) ;
#26881=ORIENTED_EDGE ( 'NONE', *, *, #43990, .F. ) ;
#26883=ORIENTED_EDGE ( 'NONE', *, *, #44981, .T. ) ;
#26884=CARTESIAN_POINT ( 'NONE',  ( 1.962558162476984114, -3.366505435497487042, 9.741991644047251597 ) ) ;
#26891=CARTESIAN_POINT ( 'NONE',  ( -6.174150299305392053, 50.00000000000000000, 8.807470649214879543 ) ) ;
#26898=ORIENTED_EDGE ( 'NONE', *, *, #29379, .T. ) ;
#26901=B_SPLINE_CURVE_WITH_KNOTS ( 'NONE', 3,
 ( #29759, #13833, #34136, #49714 ),
 .UNSPECIFIED., .F., .F.,
 ( 4, 4 ),
 ( 2.453269466693398698E-18, 0.002466147708923231013 ),
 .UNSPECIFIED. ) ;
#26912=CARTESIAN_POINT ( 'NONE',  ( 1.011271242968683648, 0.7347315653655930312, 10.00000000000000000 ) ) ;
#26913=CARTESIAN_POINT ( 'NONE',  ( -21.61731705588949737, -25.43568671410585935, -9.367992836599954742 ) ) ;
#26920=ORIENTED_EDGE ( 'NONE', *, *, #27860, .T. ) ;
#26935=ORIENTED_EDGE ( 'NONE', *, *, #32772, .F. ) ;
#26936=EDGE_CURVE ( 'NONE', #28100, #31529, #5003, .T. ) ;
#26947=CARTESIAN_POINT ( 'NONE',  ( -13.59579750444763668, 10.60877755095910935, 8.727788335465566760 ) ) ;
#26950=ORIENTED_EDGE ( 'NONE', *, *, #2594, .F. ) ;
#26961=ORIENTED_EDGE ( 'NONE', *, *, #11657, .F. ) ;
#26962=EDGE_CURVE ( 'NONE', #49029, #50662, #22722, .T. ) ;
#26965=CARTESIAN_POINT ( 'NONE',  ( -16.73672383626882976, -2.341008440547992731, -9.008049429158102583 ) ) ;
#26970=CARTESIAN_POINT ( 'NONE',  ( 16.16402646813543242, -4.033894069732437693, -3.546734833711462365 ) ) ;
#26975=CARTESIAN_POINT ( 'NONE',  ( 15.00099850811936264, 7.462898891544210933, 9.403735324607438884 ) ) ;
#26987=CARTESIAN_POINT ( 'NONE',  ( 0.2450692849603075263, -0.3373089330821618104, 9.992737347336294818 ) ) ;
#26988=CARTESIAN_POINT ( 'NONE',  ( 34.38161489319228536, -14.98878603239685070, -8.600750091277035381 ) ) ;
#27005=CARTESIAN_POINT ( 'NONE',  ( -1.780557400379564337, -1.041314823045429661, 9.889206917020301191 ) ) ;
#27013=DIRECTION ( 'NONE',  ( -1.000000000000000000, 0.000000000000000000, 0.000000000000000000 ) ) ;
#27022=ORIENTED_EDGE ( 'NONE', *, *, #27402, .F. ) ;
#27031=CARTESIAN_POINT ( 'NONE',  ( -16.91580242619126295, -33.50775492265634625, 4.835783797351798086 ) ) ;
#27041=B_SPLINE_CURVE_WITH_KNOTS ( 'NONE', 3,
 ( #19734, #42063, #3060, #7442 ),
 .UNSPECIFIED., .F., .F.,
 ( 4, 4 ),
 ( 0.000000000000000000, 0.002466147708923234483 ),
 .UNSPECIFIED. ) ;
#27042=CARTESIAN_POINT ( 'NONE',  ( -31.94178169330213279, 9.256608784834037706, -3.760136334089591248 ) ) ;
#27046=ORIENTED_EDGE ( 'NONE', *, *, #36702, .F. ) ;
#27054=FACE_OUTER_BOUND ( 'NONE', #42, .T. ) ;
#27055=CARTESIAN_POINT ( 'NONE',  ( -45.21167770612412085, -22.65616271077779942, 7.906207997025717304 ) ) ;
#27061=ORIENTED_EDGE ( 'NONE', *, *, #44607, .F. ) ;
#27073=CARTESIAN_POINT ( 'NONE',  ( -0.4166666666666669072, 0.000000000000000000, 10.00000000000000000 ) ) ;
#27079=CARTESIAN_POINT ( 'NONE',  ( 45.21167770612395742, 22.65616271077811206, 7.906207997025717304 ) ) ;
#27087=EDGE_CURVE ( 'NONE', #5199, #30729, #47769, .T. ) ;
#27089=FACE_OUTER_BOUND ( 'NONE', #4554, .T. ) ;
#27096=CARTESIAN_POINT ( 'NONE',  ( 1.011271242968688311, -0.7347315653655854817, 9.972675548442463622 ) ) ;
#27100=B_SPLINE_CURVE_WITH_KNOTS ( 'NONE', 3,
 ( #26373, #47090, #42756, #4034, #46344, #10970 ),
 .UNSPECIFIED., .F., .F.,
 ( 4, 2, 4 ),
 ( 4.906538933386797396E-18, 0.009877169331704833619, 0.01975433866340966030 ),
 .UNSPECIFIED. ) ;
#27105=VERTEX_POINT ( 'NONE', #28086 ) ;
#27114=CARTESIAN_POINT ( 'NONE',  ( 1.011271242968677653, 0.7347315653656002477, -3.333333333333333481 ) ) ;
#27116=CARTESIAN_POINT ( 'NONE',  ( -3.566525152643847285, 1.569997364305458776, 9.741991644046965604 ) ) ;
#27120=CARTESIAN_POINT ( 'NONE',  ( 16.26331699892969951, 3.800463913881183764, -9.458680755252684591 ) ) ;
#27123=EDGE_CURVE ( 'NONE', #566, #10187, #29446, .T. ) ;
#27125=CARTESIAN_POINT ( 'NONE',  ( 6.875132362119187768, -33.14667368551891258, 8.356839323120299312 ) ) ;
#27129=DIRECTION ( 'NONE',  ( -1.000000000000000000, 0.000000000000000000, 0.000000000000000000 ) ) ;
#27141=VERTEX_POINT ( 'NONE', #4476 ) ;
#27147=ADVANCED_FACE ( 'NONE', ( #16540 ), #26879, .T. ) ;
#27149=ORIENTED_EDGE ( 'NONE', *, *, #32914, .T. ) ;
#27153=CARTESIAN_POINT ( 'NONE',  ( 9.999999999999994671, -0.7319447344931275801, 9.406212099230870649 ) ) ;
#27157=CARTESIAN_POINT ( 'NONE',  ( -0.3370904143228927730, -0.2449105217885335917, 10.00000000000000000 ) ) ;
#27159=VERTEX_POINT ( 'NONE', #48802 ) ;
#27162=CARTESIAN_POINT ( 'NONE',  ( -29.12062022658179217, 29.99172060348970348, 8.846626183609803462 ) ) ;
#27171=CARTESIAN_POINT ( 'NONE',  ( -14.52758583651993618, -8.922352469211071835, 8.953103998512858652 ) ) ;
#27190=CARTESIAN_POINT ( 'NONE',  ( -15.00099850811941948, -7.462898891544107016, 9.403735324607438884 ) ) ;
#27202=ORIENTED_EDGE ( 'NONE', *, *, #5278, .T. ) ;
#27218=EDGE_CURVE ( 'NONE', #28673, #4784, #38647, .T. ) ;
#27219=CARTESIAN_POINT ( 'NONE',  ( 45.64490844644690526, 21.32281559348795597, 8.807470649214879543 ) ) ;
#27225=EDGE_CURVE ( 'NONE', #31434, #23873, #35035, .T. ) ;
#27233=EDGE_CURVE ( 'NONE', #46411, #6309, #7835, .T. ) ;
#27255=EDGE_LOOP ( 'NONE', ( #14515, #21451, #21530, #27529, #34952, #3133, #24477, #28548, #25706, #22775, #28597, #28957, #24620, #45171 ) ) ;
#27258=CARTESIAN_POINT ( 'NONE',  ( -0.5359691244547112321, 1.100286284792928893, 9.966990753365127631 ) ) ;
#27262=CARTESIAN_POINT ( 'NONE',  ( 31.44259251615245887, 38.95901822126168668, -9.367992836599954742 ) ) ;
#27272=CARTESIAN_POINT ( 'NONE',  ( 2.595273106918288164, 2.906811120256387326, 9.741991644047248045 ) ) ;
#27274=CARTESIAN_POINT ( 'NONE',  ( 0.3862712429686894766, -1.188820645368940276, 10.00000000000000000 ) ) ;
#27275=ORIENTED_EDGE ( 'NONE', *, *, #31229, .F. ) ;
#27289=EDGE_CURVE ( 'NONE', #33462, #31257, #42391, .T. ) ;
#27308=CARTESIAN_POINT ( 'NONE',  ( 1.158497635116737312, -16.61944452314319420, -3.546734833711462365 ) ) ;
#27311=CARTESIAN_POINT ( 'NONE',  ( -33.47329838550543712, 31.99020508012724662, 7.455576670931136185 ) ) ;
#27312=B_SPLINE_SURFACE_WITH_KNOTS ( 'NONE', 3, 3, ( 
 ( #46024, #26823, #11676, #11939 ),
 ( #2952, #42963, #18597, #19108 ),
 ( #46779, #22958, #34274, #3197 ),
 ( #18845, #14762, #3973, #38639 ) ),
 .UNSPECIFIED., .F., .F., .F.,
 ( 4, 4 ),
 ( 4, 4 ),
 ( 0.000000000000000000, 1.000000000000000000 ),
 ( 0.000000000000000000, 1.000000000000000000 ),
 .UNSPECIFIED. ) ;
#27314=CARTESIAN_POINT ( 'NONE',  ( -16.15814872688569181, -4.048305257546697788, -2.870787844569587133 ) ) ;
#27315=CARTESIAN_POINT ( 'NONE',  ( -50.11058929355266400, 7.578863168071933387, 7.455576670931136185 ) ) ;
#27317=CARTESIAN_POINT ( 'NONE',  ( 36.76598589393955052, 7.383243274241862331, -8.192531242611266862 ) ) ;
#27320=CARTESIAN_POINT ( 'NONE',  ( 44.99506233596246574, 23.32283626942318477, 7.455576670931136185 ) ) ;
#27322=EDGE_LOOP ( 'NONE', ( #30021, #14329, #16986, #21314 ) ) ;
#27325=CARTESIAN_POINT ( 'NONE',  ( 1.011271242968688311, -0.7347315653655855927, -10.00000000000000000 ) ) ;
#27329=ORIENTED_EDGE ( 'NONE', *, *, #10927, .T. ) ;
#27330=CARTESIAN_POINT ( 'NONE',  ( 6.196515397221660670, 4.974751005920831304, 9.432811472610147518 ) ) ;
#27331=CARTESIAN_POINT ( 'NONE',  ( -2.595273106918313033, -2.906811120256372671, 9.741991644047246268 ) ) ;
#27336=CARTESIAN_POINT ( 'NONE',  ( 11.73320209285708415, -11.96063479729170886, 9.403735324607438884 ) ) ;
#27339=EDGE_LOOP ( 'NONE', ( #15467, #823, #8491 ) ) ;
#27341=EDGE_LOOP ( 'NONE', ( #6616, #616, #8015, #47240, #40270 ) ) ;
#27362=CARTESIAN_POINT ( 'NONE',  ( 10.70590866674922204, -12.76446523155706814, -3.546734833711462365 ) ) ;
#27366=CARTESIAN_POINT ( 'NONE',  ( 2.052581215100350853, -0.2042358160480859663, 9.886433018048069954 ) ) ;
#27372=CARTESIAN_POINT ( 'NONE',  ( 48.33712804702526000, 13.03701565032775811, -9.367992836599951190 ) ) ;
#27375=CARTESIAN_POINT ( 'NONE',  ( 4.763548243873389154, -16.57409059453848599, 8.727788335465566760 ) ) ;
#27377=CARTESIAN_POINT ( 'NONE',  ( 0.3862712429686810944, 1.188820645368943607, 10.00000000000000000 ) ) ;
#27402=EDGE_CURVE ( 'NONE', #20193, #47543, #30613, .T. ) ;
#27441=AXIS2_PLACEMENT_3D ( 'NONE', #4005, #43251, #23768 ) ;
#27442=CARTESIAN_POINT ( 'NONE',  ( -17.23491422248386584, 0.5912720620001978844, 8.727788335465566760 ) ) ;
#27450=EDGE_CURVE ( 'NONE', #12217, #28949, #19812, .T. ) ;
#27454=B_SPLINE_CURVE_WITH_KNOTS ( 'NONE', 3,
 ( #41438, #48585, #9382, #21177, #17081, #1689 ),
 .UNSPECIFIED., .F., .F.,
 ( 4, 2, 4 ),
 ( 4.683753385137379155E-17, 0.009882509389272372408, 0.01976501877854469624 ),
 .UNSPECIFIED. ) ;
#27465=CARTESIAN_POINT ( 'NONE',  ( -1.193089574352124149, -0.2545860991493743564, 9.963925895596188909 ) ) ;
#27468=CARTESIAN_POINT ( 'NONE',  ( -33.57695195286787282, -16.69845195084869616, 8.914903342594564961 ) ) ;
#27482=CARTESIAN_POINT ( 'NONE',  ( 0.8965959638259385356, 1.582931917743541028, 9.903764339332076005 ) ) ;
#27483=CARTESIAN_POINT ( 'NONE',  ( 0.1287570809895630941, -0.3962735484563133515, -10.00000000000000000 ) ) ;
#27484=DIRECTION ( 'NONE',  ( -1.000000000000000000, 0.000000000000000000, -0.000000000000000000 ) ) ;
#27487=CARTESIAN_POINT ( 'NONE',  ( -13.92102703536724384, -30.85732372859812500, 8.356839323120299312 ) ) ;
#27495=CARTESIAN_POINT ( 'NONE',  ( 1.637465050678285294, 0.1702693745679431936, 9.936700280135958963 ) ) ;
#27503=CARTESIAN_POINT ( 'NONE',  ( 31.28977333267368621, -11.25592690310905652, -2.408242355805840784 ) ) ;
#27506=CARTESIAN_POINT ( 'NONE',  ( 0.5111101921243742519, 1.175566515482123098, 9.957892297621016908 ) ) ;
#27529=ORIENTED_EDGE ( 'NONE', *, *, #999, .T. ) ;
#27535=EDGE_CURVE ( 'NONE', #23241, #43972, #1807, .T. ) ;
#27541=CARTESIAN_POINT ( 'NONE',  ( 36.70770892944851482, -7.840405911381885140, 6.057468652304065060 ) ) ;
#27546=CARTESIAN_POINT ( 'NONE',  ( -15.73090589902298042, -29.60029367929041655, 1.847720168420772691 ) ) ;
#27558=CARTESIAN_POINT ( 'NONE',  ( 2.052581215100350853, -0.2042358160480859663, 9.886433018048069954 ) ) ;
#27570=CARTESIAN_POINT ( 'NONE',  ( -2.538055338523177440, -50.00000000000000711, -9.367992836599954742 ) ) ;
#27575=CARTESIAN_POINT ( 'NONE',  ( 23.79193388295309219, 28.98609808355011452, -9.422646554964176246 ) ) ;
#27578=EDGE_CURVE ( 'NONE', #48573, #38406, #44042, .T. ) ;
#27579=CARTESIAN_POINT ( 'NONE',  ( -33.43156050989129824, 4.370686678976795747, 8.807470649214879543 ) ) ;
#27582=CARTESIAN_POINT ( 'NONE',  ( -14.76429217231967428, -8.192625680377590314, 9.178419661560148768 ) ) ;
#27585=DIRECTION ( 'NONE',  ( -0.1671032855531390249, 0.5142910309547715775, 0.8411784753765542133 ) ) ;
#27588=ORIENTED_EDGE ( 'NONE', *, *, #9544, .T. ) ;
#27594=CARTESIAN_POINT ( 'NONE',  ( 9.998889670239195837, 0.1490146381531976816, 9.282506307616472441 ) ) ;
#27603=CARTESIAN_POINT ( 'NONE',  ( 36.08557433729230723, -35.58569447144768105, 7.455576670931136185 ) ) ;
#27604=CARTESIAN_POINT ( 'NONE',  ( 0.9599924130074096729, -0.8495346730527926216, 9.948547179989617462 ) ) ;
#27619=CARTESIAN_POINT ( 'NONE',  ( 1.962712821592840662, 1.022159834731142691, 9.881002359080275355 ) ) ;
#27631=DIRECTION ( 'NONE',  ( 0.000000000000000000, 0.000000000000000000, 1.000000000000000000 ) ) ;
#27633=CARTESIAN_POINT ( 'NONE',  ( 7.749480817862238524, 14.85497772329518895, 9.403735324607438884 ) ) ;
#27638=CARTESIAN_POINT ( 'NONE',  ( -33.86622497129646092, 3.037805405905158462, 7.906207997025717304 ) ) ;
#27639=CARTESIAN_POINT ( 'NONE',  ( 45.64490844644690526, 21.32281559348795597, 8.807470649214879543 ) ) ;
#27652=CARTESIAN_POINT ( 'NONE',  ( 46.75893035013449861, 17.89420872045614885, 3.199614146704519602 ) ) ;
#27667=CARTESIAN_POINT ( 'NONE',  ( -1.249999999999999778, 0.000000000000000000, 10.00000000000000000 ) ) ;
#27672=CARTESIAN_POINT ( 'NONE',  ( -44.99506233596265048, -23.32283626942287569, 7.455576670931136185 ) ) ;
#27677=FACE_OUTER_BOUND ( 'NONE', #8904, .T. ) ;
#27678=CARTESIAN_POINT ( 'NONE',  ( -1.377551617740987888, 0.6025367262284248016, 9.936141075690080982 ) ) ;
#27679=CARTESIAN_POINT ( 'NONE',  ( 41.18776771165112649, -7.147140551973409472, 8.846626183609803462 ) ) ;
#27682=CARTESIAN_POINT ( 'NONE',  ( 36.28567981536807707, 9.465698090293649614, -9.422646554964174470 ) ) ;
#27686=B_SPLINE_CURVE_WITH_KNOTS ( 'NONE', 3,
 ( #43497, #8367, #4507, #24273 ),
 .UNSPECIFIED., .F., .F.,
 ( 4, 4 ),
 ( 3.824391573920122509E-16, 0.009762429722931327200 ),
 .UNSPECIFIED. ) ;
#27694=FACE_OUTER_BOUND ( 'NONE', #50357, .T. ) ;
#27704=EDGE_LOOP ( 'NONE', ( #27202, #21903, #36580, #46091 ) ) ;
#27718=CARTESIAN_POINT ( 'NONE',  ( 1.153670525509248312, 0.4304314044324303867, 9.975326647350893694 ) ) ;
#27726=CARTESIAN_POINT ( 'NONE',  ( 27.25836557470631760, -25.76317754842347796, 8.100132398494510610 ) ) ;
#27727=B_SPLINE_SURFACE_WITH_KNOTS ( 'NONE', 3, 3, ( 
 ( #34903, #11022, #27190, #22821 ),
 ( #50482, #38501, #3314, #15389 ),
 ( #11542, #42818, #256, #4823 ),
 ( #12048, #4347, #36158, #16640 ) ),
 .UNSPECIFIED., .F., .F., .F.,
 ( 4, 4 ),
 ( 4, 4 ),
 ( 0.000000000000000000, 1.000000000000000000 ),
 ( 0.000000000000000000, 1.000000000000000000 ),
 .UNSPECIFIED. ) ;
#27741=CARTESIAN_POINT ( 'NONE',  ( 14.52758583651987223, 8.922352469211173087, 8.953103998512858652 ) ) ;
#27748=CARTESIAN_POINT ( 'NONE',  ( -1.011271242968693862, 0.7347315653655780432, -3.333333333333333481 ) ) ;
#27760=EDGE_CURVE ( 'NONE', #36434, #47506, #15266, .T. ) ;
#27763=CARTESIAN_POINT ( 'NONE',  ( 1.011271242968688311, -0.7347315653655855927, 10.00000000000000000 ) ) ;
#27767=ORIENTED_EDGE ( 'NONE', *, *, #40945, .T. ) ;
#27779=EDGE_CURVE ( 'NONE', #41040, #12195, #15894, .T. ) ;
#27786=CARTESIAN_POINT ( 'NONE',  ( -12.78770032058971395, -31.68259716188267916, 7.455576670931136185 ) ) ;
#27793=ADVANCED_FACE ( 'NONE', ( #35692 ), #11816, .F. ) ;
#27802=B_SPLINE_CURVE_WITH_KNOTS ( 'NONE', 3,
 ( #11831, #23881, #19771, #35711 ),
 .UNSPECIFIED., .F., .F.,
 ( 4, 4 ),
 ( 0.000000000000000000, 0.0001252128669263212913 ),
 .UNSPECIFIED. ) ;
#27808=CARTESIAN_POINT ( 'NONE',  ( -31.28234235046239320, -11.28615439405757392, -3.760136334089591248 ) ) ;
#27835=CARTESIAN_POINT ( 'NONE',  ( 1.158497635116737312, -16.61944452314319420, -3.546734833711462365 ) ) ;
#27838=B_SPLINE_CURVE_WITH_KNOTS ( 'NONE', 3,
 ( #27558, #23450, #43194, #16755 ),
 .UNSPECIFIED., .F., .F.,
 ( 4, 4 ),
 ( 0.001937412222931639630, 0.003978261222106106373 ),
 .UNSPECIFIED. ) ;
#27840=ORIENTED_EDGE ( 'NONE', *, *, #12171, .T. ) ;
#27844=B_SPLINE_CURVE_WITH_KNOTS ( 'NONE', 3,
 ( #39913, #24503, #40409, #4743 ),
 .UNSPECIFIED., .F., .F.,
 ( 4, 4 ),
 ( 0.000000000000000000, 0.2637263876330695478 ),
 .UNSPECIFIED. ) ;
#27847=VERTEX_POINT ( 'NONE', #35180 ) ;
#27849=CARTESIAN_POINT ( 'NONE',  ( -0.3862712429686977478, 1.188820645368937390, 10.00000000000000000 ) ) ;
#27851=CARTESIAN_POINT ( 'NONE',  ( 0.3896797354184660667, -1.262193838292004155, 9.943883492372872723 ) ) ;
#27860=EDGE_CURVE ( 'NONE', #12051, #7897, #32445, .T. ) ;
#27862=CARTESIAN_POINT ( 'NONE',  ( 1.114871695981101585, -0.4953159757246433093, 9.963925895596188909 ) ) ;
#27867=CARTESIAN_POINT ( 'NONE',  ( 6.174150299305392053, -33.14591993373988998, 8.807470649214879543 ) ) ;
#27868=DIRECTION ( 'NONE',  ( 0.5407575913134975432, 0.000000000000000000, 0.8411784753765542133 ) ) ;
#27872=EDGE_CURVE ( 'NONE', #1058, #27141, #28167, .T. ) ;
#27873=CARTESIAN_POINT ( 'NONE',  ( 1.377636575563020438, -0.6021164824561170414, 9.953784399990622589 ) ) ;
#27875=ORIENTED_EDGE ( 'NONE', *, *, #4635, .F. ) ;
#27881=ORIENTED_EDGE ( 'NONE', *, *, #18964, .T. ) ;
#27882=CARTESIAN_POINT ( 'NONE',  ( 2.143303323993648313, -0.2858885274053867276, 9.882710035074774524 ) ) ;
#27887=B_SPLINE_CURVE_WITH_KNOTS ( 'NONE', 3,
 ( #50253, #15164, #30824, #3605 ),
 .UNSPECIFIED., .F., .F.,
 ( 4, 4 ),
 ( 0.0001265805828163032185, 0.0005567784772122129572 ),
 .UNSPECIFIED. ) ;
#27891=CARTESIAN_POINT ( 'NONE',  ( -0.3862712429686809279, -1.188820645368943163, 10.00000000000000000 ) ) ;
#27911=CARTESIAN_POINT ( 'NONE',  ( 2.816440797479290659, -7.430518950464442440, 9.432811472610140413 ) ) ;
#27913=ORIENTED_EDGE ( 'NONE', *, *, #10239, .T. ) ;
#27922=EDGE_LOOP ( 'NONE', ( #50565, #32385, #19877, #6635 ) ) ;
#27932=CARTESIAN_POINT ( 'NONE',  ( -7.216980890441389462, 6.922079660550276792, 0.000000000000000000 ) ) ;
#27934=CARTESIAN_POINT ( 'NONE',  ( 31.44259251615245176, 38.95901822126168668, -9.367992836599951190 ) ) ;
#27936=CARTESIAN_POINT ( 'NONE',  ( 1.565984505217804967, -1.491012526244388292, 9.885585981620945262 ) ) ;
#27937=CARTESIAN_POINT ( 'NONE',  ( 34.10310225234744763, 15.68274378628490773, 1.982731392810414661 ) ) ;
#27947=CARTESIAN_POINT ( 'NONE',  ( 48.33712804702526000, 13.03701565032775456, -9.367992836599954742 ) ) ;
#27950=CARTESIAN_POINT ( 'NONE',  ( -1.468713901642213493, -0.3220470327672489419, 9.927319414211227766 ) ) ;
#27957=EDGE_LOOP ( 'NONE', ( #9672, #25137, #5603, #26800 ) ) ;
#27960=ORIENTED_EDGE ( 'NONE', *, *, #8270, .T. ) ;
#27974=ORIENTED_EDGE ( 'NONE', *, *, #46763, .F. ) ;
#27979=CARTESIAN_POINT ( 'NONE',  ( 42.07173315646062406, -18.54977254542396636, -8.016098858316205167 ) ) ;
#27987=CARTESIAN_POINT ( 'NONE',  ( 0.3370904143228947158, 0.2449105217885311492, 10.00000000000000000 ) ) ;
#28007=ORIENTED_EDGE ( 'NONE', *, *, #26877, .T. ) ;
#28011=FACE_OUTER_BOUND ( 'NONE', #15595, .T. ) ;
#28020=DIRECTION ( 'NONE',  ( -0.5407575913134975432, -0.000000000000000000, 0.8411784753765542133 ) ) ;
#28022=CARTESIAN_POINT ( 'NONE',  ( -0.8284317003875021346, -1.889026769141635587, 9.889206917020304743 ) ) ;
#28037=B_SPLINE_CURVE_WITH_KNOTS ( 'NONE', 3,
 ( #28710, #25117, #16648, #40764 ),
 .UNSPECIFIED., .F., .F.,
 ( 4, 4 ),
 ( 0.000000000000000000, 0.2545280377015990969 ),
 .UNSPECIFIED. ) ;
#28039=CARTESIAN_POINT ( 'NONE',  ( -6.619412807845042046, 7.495556955913086128, 9.646707543097347681 ) ) ;
#28041=ADVANCED_FACE ( 'NONE', ( #12819 ), #32257, .T. ) ;
#28053=ORIENTED_EDGE ( 'NONE', *, *, #22075, .F. ) ;
#28057=CARTESIAN_POINT ( 'NONE',  ( 1.724908962443185922, -9.880865948510580310, 9.516222621873128062 ) ) ;
#28064=ORIENTED_EDGE ( 'NONE', *, *, #44603, .T. ) ;
#28070=B_SPLINE_CURVE_WITH_KNOTS ( 'NONE', 3,
 ( #34026, #45776, #38384, #14761 ),
 .UNSPECIFIED., .F., .F.,
 ( 4, 4 ),
 ( 0.9890644561681873892, 1.000000000000000000 ),
 .UNSPECIFIED. ) ;
#28078=B_SPLINE_CURVE_WITH_KNOTS ( 'NONE', 3,
 ( #27317, #42948, #23475, #39136, #3958, #19606 ),
 .UNSPECIFIED., .F., .F.,
 ( 4, 2, 4 ),
 ( 5.818439421673296370E-18, 0.009877169331704826680, 0.01975433866340964989 ),
 .UNSPECIFIED. ) ;
#28086=CARTESIAN_POINT ( 'NONE',  ( 37.50000000000000000, 4.592425496802574367E-15, -10.00000000000000000 ) ) ;
#28087=AXIS2_PLACEMENT_3D ( 'NONE', #5183, #1097, #16735 ) ;
#28100=VERTEX_POINT ( 'NONE', #27604 ) ;
#28114=CARTESIAN_POINT ( 'NONE',  ( -0.3862712429686977478, 1.188820645368937390, 10.00000000000000000 ) ) ;
#28119=ORIENTED_EDGE ( 'NONE', *, *, #30306, .F. ) ;
#28137=CARTESIAN_POINT ( 'NONE',  ( 0.5705203167769784534, 1.169354363542900010, 9.986087673579197244 ) ) ;
#28146=DIRECTION ( 'NONE',  ( -0.1671032855531282835, -0.5142910309547751302, -0.8411784753765542133 ) ) ;
#28147=CARTESIAN_POINT ( 'NONE',  ( 34.38425513258721367, -36.82177522737821107, 8.807470649214879543 ) ) ;
#28148=FACE_OUTER_BOUND ( 'NONE', #27704, .T. ) ;
#28151=CARTESIAN_POINT ( 'NONE',  ( 0.8784099037133200616, 0.8517617868932368941, 9.993783931180534097 ) ) ;
#28152=B_SPLINE_SURFACE_WITH_KNOTS ( 'NONE', 3, 3, ( 
 ( #34771, #31164, #23461, #46754 ),
 ( #43452, #19347, #11654, #22938 ),
 ( #20105, #47012, #27308, #42938 ),
 ( #27570, #39621, #23711, #15748 ) ),
 .UNSPECIFIED., .F., .F., .F.,
 ( 4, 4 ),
 ( 4, 4 ),
 ( 0.000000000000000000, 1.000000000000000000 ),
 ( 0.000000000000000000, 1.000000000000000000 ),
 .UNSPECIFIED. ) ;
#28159=VECTOR ( 'NONE', #27868, 1000.000000000000114 ) ;
#28161=CARTESIAN_POINT ( 'NONE',  ( -34.38425513258695077, 36.82177522737848108, 8.807470649214879543 ) ) ;
#28167=B_SPLINE_CURVE_WITH_KNOTS ( 'NONE', 3,
 ( #34928, #12069, #19, #20266 ),
 .UNSPECIFIED., .F., .F.,
 ( 4, 4 ),
 ( 0.7491799374948681089, 1.000000000000000000 ),
 .UNSPECIFIED. ) ;
#28176=ORIENTED_EDGE ( 'NONE', *, *, #47845, .F. ) ;
#28192=CARTESIAN_POINT ( 'NONE',  ( 0.3862712429686978033, -1.188820645368937834, 10.00000000000000000 ) ) ;
#28197=ORIENTED_EDGE ( 'NONE', *, *, #9544, .F. ) ;
#28209=VERTEX_POINT ( 'NONE', #27851 ) ;
#28210=CARTESIAN_POINT ( 'NONE',  ( 30.87089393895375267, -12.69923079256617449, -9.367992836599954742 ) ) ;
#28226=ADVANCED_FACE ( 'NONE', ( #36584 ), #4379, .T. ) ;
#28228=CARTESIAN_POINT ( 'NONE',  ( 10.00000000000000000, 1.224646799147353256E-15, 10.00000000000000000 ) ) ;
#28238=B_SPLINE_CURVE_WITH_KNOTS ( 'NONE', 3,
 ( #14743, #7051, #2439, #22691 ),
 .UNSPECIFIED., .F., .F.,
 ( 4, 4 ),
 ( 0.0006669682284780878911, 0.0007799402130920262462 ),
 .UNSPECIFIED. ) ;
#28239=CARTESIAN_POINT ( 'NONE',  ( 26.25702031264353664, -26.77347351953840615, 8.914903342594564961 ) ) ;
#28246=CIRCLE ( 'NONE', #6105, 10.00000000000000000 ) ;
#28251=VECTOR ( 'NONE', #31733, 1000.000000000000000 ) ;
#28253=ORIENTED_EDGE ( 'NONE', *, *, #13029, .F. ) ;
#28267=EDGE_LOOP ( 'NONE', ( #8002, #7148, #1730, #463 ) ) ;
#28272=CARTESIAN_POINT ( 'NONE',  ( 8.831420117243668599, 14.12636088103192655, -3.546734833711462365 ) ) ;
#28280=CARTESIAN_POINT ( 'NONE',  ( -0.3862712429686729343, -1.188820645368946050, 10.00000000000000000 ) ) ;
#28288=ORIENTED_EDGE ( 'NONE', *, *, #35058, .F. ) ;
#28297=ORIENTED_EDGE ( 'NONE', *, *, #34413, .T. ) ;
#28299=ORIENTED_EDGE ( 'NONE', *, *, #50101, .F. ) ;
#28301=CARTESIAN_POINT ( 'NONE',  ( -0.1425549192113998442, 1.238581250503548059, 9.981352469109934233 ) ) ;
#28303=CARTESIAN_POINT ( 'NONE',  ( -5.505322767148756569, 37.09368438467003415, 8.914903342594564961 ) ) ;
#28310=CARTESIAN_POINT ( 'NONE',  ( -6.174150299305392053, 50.00000000000000711, 8.807470649214879543 ) ) ;
#28317=FACE_OUTER_BOUND ( 'NONE', #40421, .T. ) ;
#28329=CARTESIAN_POINT ( 'NONE',  ( 1.540662627795932105, -1.371465786296032441, 9.894754715216729224 ) ) ;
#28330=EDGE_LOOP ( 'NONE', ( #50155, #29058, #15329, #2975 ) ) ;
#28337=CARTESIAN_POINT ( 'NONE',  ( 33.43156050989131955, -4.370686678976570150, 8.807470649214879543 ) ) ;
#28344=CARTESIAN_POINT ( 'NONE',  ( 32.36066692128250821, -7.813306791042813337, 3.199614146704519602 ) ) ;
#28348=B_SPLINE_CURVE_WITH_KNOTS ( 'NONE', 3,
 ( #15749, #8322, #31420, #1130 ),
 .UNSPECIFIED., .F., .F.,
 ( 4, 4 ),
 ( 0.000000000000000000, 0.002458791966311101550 ),
 .UNSPECIFIED. ) ;
#28350=CARTESIAN_POINT ( 'NONE',  ( 14.29087950072012170, 9.652079258044652832, 8.727788335465566760 ) ) ;
#28352=CARTESIAN_POINT ( 'NONE',  ( 29.61572577327002520, 16.11461842845735859, 8.807470649214879543 ) ) ;
#28355=ORIENTED_EDGE ( 'NONE', *, *, #20906, .T. ) ;
#28365=CARTESIAN_POINT ( 'NONE',  ( -1.142975459103954705, -16.61830776097024653, -2.870787844569587133 ) ) ;
#28369=EDGE_CURVE ( 'NONE', #11925, #19313, #14953, .T. ) ;
#28409=CARTESIAN_POINT ( 'NONE',  ( -0.5270093351535434234, 0.6444734225979527054, 9.985686052694763504 ) ) ;
#28420=CARTESIAN_POINT ( 'NONE',  ( -34.08406891383351933, 15.63733501198486309, -8.192531242611266862 ) ) ;
#28426=CARTESIAN_POINT ( 'NONE',  ( 7.129058724844953510, 15.30620660340485095, 9.178419661560148768 ) ) ;
#28437=CARTESIAN_POINT ( 'NONE',  ( -34.08406891383351933, 15.63733501198486309, -8.192531242611266862 ) ) ;
#28443=CARTESIAN_POINT ( 'NONE',  ( 36.28567981536807707, 9.465698090293649614, -9.422646554964174470 ) ) ;
#28465=CARTESIAN_POINT ( 'NONE',  ( 0.3862712429686727678, 1.188820645368945605, -10.00000000000000000 ) ) ;
#28469=B_SPLINE_SURFACE_WITH_KNOTS ( 'NONE', 3, 3, ( 
 ( #39226, #19711, #35390, #10998 ),
 ( #31531, #47117, #42299, #38473 ),
 ( #3285, #18933, #43807, #36137 ),
 ( #20981, #17124, #40224, #36912 ) ),
 .UNSPECIFIED., .F., .F., .F.,
 ( 4, 4 ),
 ( 4, 4 ),
 ( 0.000000000000000000, 1.000000000000000000 ),
 ( 0.000000000000000000, 1.000000000000000000 ),
 .UNSPECIFIED. ) ;
#28475=ORIENTED_EDGE ( 'NONE', *, *, #32022, .T. ) ;
#28500=CARTESIAN_POINT ( 'NONE',  ( -25.61277432017861955, 22.36370378792854297, 7.906207997025717304 ) ) ;
#28536=CARTESIAN_POINT ( 'NONE',  ( -0.3093295598751883979, 2.058753478587400654, 9.888794896520666455 ) ) ;
#28548=ORIENTED_EDGE ( 'NONE', *, *, #3586, .T. ) ;
#28551=ORIENTED_EDGE ( 'NONE', *, *, #9316, .T. ) ;
#28556=CARTESIAN_POINT ( 'NONE',  ( -47.22310614333779455, -16.46562252335923660, -3.760136334089591248 ) ) ;
#28569=B_SPLINE_SURFACE_WITH_KNOTS ( 'NONE', 3, 3, ( 
 ( #18169, #49438, #14325, #45607 ),
 ( #29992, #10481, #26128, #40378 ),
 ( #48020, #47527, #12408, #11914 ),
 ( #12906, #43453, #5216, #4461 ) ),
 .UNSPECIFIED., .F., .F., .F.,
 ( 4, 4 ),
 ( 4, 4 ),
 ( 0.000000000000000000, 1.000000000000000000 ),
 ( 0.000000000000000000, 1.000000000000000000 ),
 .UNSPECIFIED. ) ;
#28587=CARTESIAN_POINT ( 'NONE',  ( -4.641001526964561918, -50.00000000000000711, -8.016098858316205167 ) ) ;
#28593=CARTESIAN_POINT ( 'NONE',  ( -0.5953091869874307385, -3.900377600830043257, 6.494306115488110542 ) ) ;
#28597=ORIENTED_EDGE ( 'NONE', *, *, #27578, .T. ) ;
#28604=CARTESIAN_POINT ( 'NONE',  ( -4.641001526964560142, -33.28196331604080171, -8.016098858316199838 ) ) ;
#28605=CARTESIAN_POINT ( 'NONE',  ( 29.39982726364966581, 16.78152490921169360, 8.356839323120299312 ) ) ;
#28612=CARTESIAN_POINT ( 'NONE',  ( 7.608425291889091113, -36.72004717559254772, 7.697694107796188234 ) ) ;
#28620=CARTESIAN_POINT ( 'NONE',  ( -47.88254548617756967, 14.43607691413558669, -3.760136334089591248 ) ) ;
#28632=CARTESIAN_POINT ( 'NONE',  ( 1.540617191852273526, -1.371546265746151017, 9.891980816076527461 ) ) ;
#28635=FACE_OUTER_BOUND ( 'NONE', #46702, .T. ) ;
#28637=ORIENTED_EDGE ( 'NONE', *, *, #27578, .F. ) ;
#28639=CARTESIAN_POINT ( 'NONE',  ( 1.448406091252584238, -0.9360325558322883932, 9.928159647716132241 ) ) ;
#28642=CARTESIAN_POINT ( 'NONE',  ( -1.540526284687967706, 1.371707213411501147, 9.886433018048069954 ) ) ;
#28647=CARTESIAN_POINT ( 'NONE',  ( -33.64889274059387958, 3.704246042440976439, 8.356839323120299312 ) ) ;
#28648=CARTESIAN_POINT ( 'NONE',  ( 1.337801958641917199, 1.088266084286984015, 9.928159647716135794 ) ) ;
#28661=CARTESIAN_POINT ( 'NONE',  ( 0.7606162131530698201, -1.296876929034913140, 9.953784399990620813 ) ) ;
#28663=CARTESIAN_POINT ( 'NONE',  ( -4.672045878990125800, 50.00000000000000711, 1.847720168420772691 ) ) ;
#28665=CARTESIAN_POINT ( 'NONE',  ( 0.2050626648100478400, -1.807624707196173519, 9.903764339332001398 ) ) ;
#28668=FACE_OUTER_BOUND ( 'NONE', #2653, .T. ) ;
#28672=CARTESIAN_POINT ( 'NONE',  ( -1.275971930252334019, 0.1228246474626440710, 9.957892297621013356 ) ) ;
#28673=VERTEX_POINT ( 'NONE', #29798 ) ;
#28675=CARTESIAN_POINT ( 'NONE',  ( 0.9601844228325747688, -0.8491947203466810867, 9.967237415621763574 ) ) ;
#28709=CARTESIAN_POINT ( 'NONE',  ( 0.3862712429686727678, 1.188820645368945605, 10.00000000000000000 ) ) ;
#28710=CARTESIAN_POINT ( 'NONE',  ( 25.63461350838963071, -43.17876197216376255, -8.016098858316205167 ) ) ;
#28739=ORIENTED_EDGE ( 'NONE', *, *, #22995, .F. ) ;
#28755=CARTESIAN_POINT ( 'NONE',  ( -1.011271242968687867, 0.7347315653655861478, 9.972675548442463622 ) ) ;
#28761=EDGE_CURVE ( 'NONE', #10360, #45145, #18032, .T. ) ;
#28762=CARTESIAN_POINT ( 'NONE',  ( 9.907356528111447957, -1.358045148324435347, 0.000000000000000000 ) ) ;
#28766=ORIENTED_EDGE ( 'NONE', *, *, #13644, .T. ) ;
#28769=CARTESIAN_POINT ( 'NONE',  ( 25.61277432017878297, -22.36370378792834757, 7.906207997025717304 ) ) ;
#28774=CARTESIAN_POINT ( 'NONE',  ( -37.50000000000000000, 0.000000000000000000, -10.00000000000000000 ) ) ;
#28782=CARTESIAN_POINT ( 'NONE',  ( -0.1287570809895576818, -0.3962735484563154609, 10.00000000000000000 ) ) ;
#28788=ORIENTED_EDGE ( 'NONE', *, *, #29928, .T. ) ;
#28789=CARTESIAN_POINT ( 'NONE',  ( 3.566525152641073504, -1.569997364302916809, 9.741991644047246268 ) ) ;
#28806=ORIENTED_EDGE ( 'NONE', *, *, #29577, .F. ) ;
#28816=CARTESIAN_POINT ( 'NONE',  ( -7.576114424932982594, 33.14742743729794938, 7.906207997025717304 ) ) ;
#28838=CARTESIAN_POINT ( 'NONE',  ( 46.33529284216721322, -19.19803090445725502, -8.466730184410787174 ) ) ;
#28841=CARTESIAN_POINT ( 'NONE',  ( 34.08355720199905647, -2.371364769369109116, 7.455576670931136185 ) ) ;
#28845=CARTESIAN_POINT ( 'NONE',  ( 1.249999999999999778, 0.000000000000000000, 10.00000000000000000 ) ) ;
#28846=EDGE_CURVE ( 'NONE', #33857, #5897, #31510, .T. ) ;
#28856=EDGE_CURVE ( 'NONE', #21132, #29819, #16140, .T. ) ;
#28861=CARTESIAN_POINT ( 'NONE',  ( 1.011271242968683648, 0.7347315653655930312, 10.00000000000000000 ) ) ;
#28868=DIRECTION ( 'NONE',  ( -0.5407575913134976542, 0.000000000000000000, -0.8411784753765542133 ) ) ;
#28872=CARTESIAN_POINT ( 'NONE',  ( 50.11058929355270664, -7.578863168071591438, 7.455576670931136185 ) ) ;
#28879=CARTESIAN_POINT ( 'NONE',  ( 31.84561714023325507, -33.32763979208104388, 8.807470649214879543 ) ) ;
#28881=CARTESIAN_POINT ( 'NONE',  ( -17.23491422248386584, 0.5912720620001978844, 8.727788335465566760 ) ) ;
#28884=B_SPLINE_SURFACE_WITH_KNOTS ( 'NONE', 3, 3, ( 
 ( #17970, #40587, #20822, #40830 ),
 ( #5676, #5425, #21578, #29036 ),
 ( #36505, #9035, #32640, #32902 ),
 ( #17741, #17483, #21332, #24691 ) ),
 .UNSPECIFIED., .F., .F., .F.,
 ( 4, 4 ),
 ( 4, 4 ),
 ( 0.000000000000000000, 1.000000000000000000 ),
 ( 0.000000000000000000, 1.000000000000000000 ),
 .UNSPECIFIED. ) ;
#28885=CARTESIAN_POINT ( 'NONE',  ( -28.55116071645519327, 41.05976639056880373, -2.408242355805840784 ) ) ;
#28888=CARTESIAN_POINT ( 'NONE',  ( 9.999999999999998224, -0.4417425667975402037, 5.558078895815850906 ) ) ;
#28894=CARTESIAN_POINT ( 'NONE',  ( -5.888214538810513154, -16.20866436362413410, 8.727788335465566760 ) ) ;
#28898=CARTESIAN_POINT ( 'NONE',  ( 12.97493236725083676, -11.05939663306990717, 8.953103998512858652 ) ) ;
#28913=ADVANCED_FACE ( 'NONE', ( #3091 ), #18992, .F. ) ;
#28914=B_SPLINE_CURVE_WITH_KNOTS ( 'NONE', 3,
 ( #29375, #9625, #25524, #27932 ),
 .UNSPECIFIED., .F., .F.,
 ( 4, 4 ),
 ( 0.000000000000000000, 0.009404495247862304161 ),
 .UNSPECIFIED. ) ;
#28915=CARTESIAN_POINT ( 'NONE',  ( -8.277096487746778308, 50.00000000000000711, 7.455576670931136185 ) ) ;
#28916=CARTESIAN_POINT ( 'NONE',  ( -28.52604530808686079, -41.07801380285659576, -3.760136334089591248 ) ) ;
#28929=LINE ( 'NONE', #9930, #8395 ) ;
#28934=CARTESIAN_POINT ( 'NONE',  ( -1.011271242968677875, -0.7347315653656004697, -3.333333333333333481 ) ) ;
#28941=CARTESIAN_POINT ( 'NONE',  ( -36.08557433729205144, 35.58569447144795816, 7.455576670931136185 ) ) ;
#28944=CARTESIAN_POINT ( 'NONE',  ( 1.011271242968683648, 0.7347315653655930312, -10.00000000000000000 ) ) ;
#28949=VERTEX_POINT ( 'NONE', #16181 ) ;
#28957=ORIENTED_EDGE ( 'NONE', *, *, #11170, .F. ) ;
#28960=ORIENTED_EDGE ( 'NONE', *, *, #6840, .F. ) ;
#28965=FACE_OUTER_BOUND ( 'NONE', #38713, .T. ) ;
#28968=CARTESIAN_POINT ( 'NONE',  ( 45.42829307628542779, 21.98948915213303579, 8.356839323120299312 ) ) ;
#28972=CARTESIAN_POINT ( 'NONE',  ( 0.5386300094813488704, -1.098626330213929636, 9.993783931180535873 ) ) ;
#28985=B_SPLINE_SURFACE_WITH_KNOTS ( 'NONE', 3, 3, ( 
 ( #14932, #30332, #45944, #3369 ),
 ( #50279, #30851, #46445, #8511 ),
 ( #16202, #16455, #47959, #27748 ),
 ( #4398, #20046, #19524, #35212 ) ),
 .UNSPECIFIED., .F., .F., .F.,
 ( 4, 4 ),
 ( 4, 4 ),
 ( 0.000000000000000000, 1.000000000000000000 ),
 ( 0.000000000000000000, 1.000000000000000000 ),
 .UNSPECIFIED. ) ;
#28993=CARTESIAN_POINT ( 'NONE',  ( -0.2778388845795317086, 1.251314014313103851, 9.976582533991678048 ) ) ;
#29002=ADVANCED_FACE ( 'NONE', ( #20523 ), #46507, .T. ) ;
#29006=CARTESIAN_POINT ( 'NONE',  ( -29.18392875402943432, -17.44843138996582965, 7.906207997025717304 ) ) ;
#29010=CARTESIAN_POINT ( 'NONE',  ( 33.14391172085757375, 37.72293746533118508, -8.016098858316205167 ) ) ;
#29012=CARTESIAN_POINT ( 'NONE',  ( -16.02661358026017879, -4.530191650547607196, -9.683996418299976483 ) ) ;
#29013=FACE_OUTER_BOUND ( 'NONE', #25077, .T. ) ;
#29031=ORIENTED_EDGE ( 'NONE', *, *, #33777, .F. ) ;
#29034=CARTESIAN_POINT ( 'NONE',  ( 49.67735855322978011, -8.912210285361751971, 8.356839323120299312 ) ) ;
#29036=CARTESIAN_POINT ( 'NONE',  ( -0.3862712429686977478, 1.188820645368937390, 3.333333333333333481 ) ) ;
#29045=CARTESIAN_POINT ( 'NONE',  ( 0.000000000000000000, 0.000000000000000000, 0.000000000000000000 ) ) ;
#29051=CARTESIAN_POINT ( 'NONE',  ( 8.277096487746778308, -50.00000000000000711, 7.455576670931136185 ) ) ;
#29058=ORIENTED_EDGE ( 'NONE', *, *, #42506, .F. ) ;
#29059=CARTESIAN_POINT ( 'NONE',  ( -5.083187235775261215, -8.611690166631138510, 9.646707543097347681 ) ) ;
#29060=CARTESIAN_POINT ( 'NONE',  ( 15.98719783915691650, -4.501063718205879916, 3.266473740018926541 ) ) ;
#29094=ORIENTED_EDGE ( 'NONE', *, *, #15768, .T. ) ;
#29095=FACE_OUTER_BOUND ( 'NONE', #35752, .T. ) ;
#29099=ORIENTED_EDGE ( 'NONE', *, *, #19618, .F. ) ;
#29101=CARTESIAN_POINT ( 'NONE',  ( -3.239037401336969602, -33.28348308860766025, -8.917361510505369182 ) ) ;
#29106=DIRECTION ( 'NONE',  ( 0.9510565162951523099, 0.3090169943749515591, 0.000000000000000000 ) ) ;
#29119=VECTOR ( 'NONE', #44804, 1000.000000000000000 ) ;
#29124=ORIENTED_EDGE ( 'NONE', *, *, #6531, .T. ) ;
#29136=EDGE_LOOP ( 'NONE', ( #38903, #2635, #6551, #2879 ) ) ;
#29137=CARTESIAN_POINT ( 'NONE',  ( -50.11058929355266400, 7.578863168071933387, 7.455576670931136185 ) ) ;
#29147=CARTESIAN_POINT ( 'NONE',  ( 2.462075149652696027, -16.57295996686994499, 9.403735324607438884 ) ) ;
#29150=CARTESIAN_POINT ( 'NONE',  ( 0.3862712429686810944, 1.188820645368943607, 10.00000000000000000 ) ) ;
#29154=B_SPLINE_CURVE_WITH_KNOTS ( 'NONE', 3,
 ( #30556, #27718, #46154, #11308 ),
 .UNSPECIFIED., .F., .F.,
 ( 4, 4 ),
 ( 0.000000000000000000, 0.0002708531562905854440 ),
 .UNSPECIFIED. ) ;
#29158=CARTESIAN_POINT ( 'NONE',  ( -37.50000000000000000, 0.000000000000000000, 10.00000000000000000 ) ) ;
#29160=VERTEX_POINT ( 'NONE', #7149 ) ;
#29164=CARTESIAN_POINT ( 'NONE',  ( -16.76006782980216059, 2.050259795448645228, 9.178419661560148768 ) ) ;
#29168=VERTEX_POINT ( 'NONE', #34603 ) ;
#29169=CARTESIAN_POINT ( 'NONE',  ( 1.782521105131670724, -0.3635605703593869920, 9.903764339332079558 ) ) ;
#29178=CARTESIAN_POINT ( 'NONE',  ( -8.831420117243776957, -14.12636088103186260, -3.546734833711462365 ) ) ;
#29181=DIRECTION ( 'NONE',  ( 1.000000000000000000, 0.000000000000000000, 0.000000000000000000 ) ) ;
#29194=CARTESIAN_POINT ( 'NONE',  ( -1.305887768059462717, 0.05395936523972331283, 9.945465957785078359 ) ) ;
#29203=CARTESIAN_POINT ( 'NONE',  ( -30.25247992116029394, 39.82368563463828792, -3.760136334089591248 ) ) ;
#29204=CARTESIAN_POINT ( 'NONE',  ( -34.38425513258695077, 36.82177522737848108, 8.807470649214879543 ) ) ;
#29246=CARTESIAN_POINT ( 'NONE',  ( 0.6721397084974982672, 9.977385840602783773, 2.154851817814940063E-15 ) ) ;
#29257=FACE_OUTER_BOUND ( 'NONE', #4943, .T. ) ;
#29258=CARTESIAN_POINT ( 'NONE',  ( 0.3862712429686810944, 1.188820645368943607, 10.00000000000000000 ) ) ;
#29267=EDGE_CURVE ( 'NONE', #35077, #1823, #49160, .T. ) ;
#29270=CARTESIAN_POINT ( 'NONE',  ( -6.875132362119187768, 33.14667368551891258, 8.356839323120299312 ) ) ;
#29274=CARTESIAN_POINT ( 'NONE',  ( 1.578643388466006714, -1.550786058692517511, 9.881002359080275355 ) ) ;
#29276=EDGE_CURVE ( 'NONE', #8731, #35155, #37033, .T. ) ;
#29278=ORIENTED_EDGE ( 'NONE', *, *, #20548, .T. ) ;
#29286=CARTESIAN_POINT ( 'NONE',  ( -1.540662627795934769, 1.371465786296043765, 9.894754715216725671 ) ) ;
#29288=VERTEX_POINT ( 'NONE', #10487 ) ;
#29295=ORIENTED_EDGE ( 'NONE', *, *, #6477, .F. ) ;
#29303=B_SPLINE_SURFACE_WITH_KNOTS ( 'NONE', 3, 3, ( 
 ( #1425, #36331, #17992, #24769 ),
 ( #16559, #4751, #43992, #9114 ),
 ( #14140, #13203, #32716, #20393 ),
 ( #48057, #18242, #22106, #28861 ) ),
 .UNSPECIFIED., .F., .F., .F.,
 ( 4, 4 ),
 ( 4, 4 ),
 ( 0.000000000000000000, 1.000000000000000000 ),
 ( 0.000000000000000000, 1.000000000000000000 ),
 .UNSPECIFIED. ) ;
#29306=CARTESIAN_POINT ( 'NONE',  ( -14.91630425054805187, 7.943683830272224355, -9.008049429158100807 ) ) ;
#29307=CARTESIAN_POINT ( 'NONE',  ( 1.343171584779923933, -1.414327272009459291, 9.896382706792440587 ) ) ;
#29328=ORIENTED_EDGE ( 'NONE', *, *, #27289, .F. ) ;
#29333=EDGE_CURVE ( 'NONE', #31279, #32219, #14369, .T. ) ;
#29334=CARTESIAN_POINT ( 'NONE',  ( 0.3862712429686810944, 1.188820645368943607, 10.00000000000000000 ) ) ;
#29336=CARTESIAN_POINT ( 'NONE',  ( -20.37409433808010562, -26.28007012093468475, -2.408242355805840784 ) ) ;
#29338=CARTESIAN_POINT ( 'NONE',  ( 45.64490844644690526, 21.32281559348795597, 8.807470649214879543 ) ) ;
#29342=ORIENTED_EDGE ( 'NONE', *, *, #13429, .F. ) ;
#29343=B_SPLINE_CURVE_WITH_KNOTS ( 'NONE', 3,
 ( #33757, #34727, #20064, #39581 ),
 .UNSPECIFIED., .F., .F.,
 ( 4, 4 ),
 ( 0.000000000000000000, 0.001249001861321270834 ),
 .UNSPECIFIED. ) ;
#29344=CARTESIAN_POINT ( 'NONE',  ( 7.749480817862238524, 14.85497772329518895, 9.403735324607438884 ) ) ;
#29345=DIRECTION ( 'NONE',  ( 0.000000000000000000, 0.000000000000000000, -1.000000000000000000 ) ) ;
#29352=CARTESIAN_POINT ( 'NONE',  ( -0.3862712429686977478, 1.188820645368937390, -10.00000000000000000 ) ) ;
#29361=ADVANCED_FACE ( 'NONE', ( #15360 ), #46928, .T. ) ;
#29372=CARTESIAN_POINT ( 'NONE',  ( -1.769963848780949478, 9.842115015280430868, 0.000000000000000000 ) ) ;
#29375=CARTESIAN_POINT ( 'NONE',  ( -8.176860274785726190, 5.756644512789648616, 9.282506307616472441 ) ) ;
#29379=EDGE_CURVE ( 'NONE', #16336, #12217, #32538, .T. ) ;
#29381=ORIENTED_EDGE ( 'NONE', *, *, #10833, .F. ) ;
#29393=CARTESIAN_POINT ( 'NONE',  ( 1.011271242968688311, -0.7347315653655855927, 10.00000000000000000 ) ) ;
#29398=CARTESIAN_POINT ( 'NONE',  ( 36.97942854200454832, -6.226705766838405154, 8.914903342594563185 ) ) ;
#29401=B_SPLINE_SURFACE_WITH_KNOTS ( 'NONE', 3, 3, ( 
 ( #40680, #36602, #48322, #39930 ),
 ( #36850, #5516, #36086, #16067 ),
 ( #13211, #44493, #12206, #4513 ),
 ( #28872, #666, #8374, #8622 ) ),
 .UNSPECIFIED., .F., .F., .F.,
 ( 4, 4 ),
 ( 4, 4 ),
 ( 0.000000000000000000, 1.000000000000000000 ),
 ( 0.000000000000000000, 1.000000000000000000 ),
 .UNSPECIFIED. ) ;
#29413=B_SPLINE_CURVE_WITH_KNOTS ( 'NONE', 3,
 ( #38011, #49741, #47667, #11817 ),
 .UNSPECIFIED., .F., .F.,
 ( 4, 4 ),
 ( 0.7491799374948677759, 1.000000000000000000 ),
 .UNSPECIFIED. ) ;
#29414=CARTESIAN_POINT ( 'NONE',  ( -1.066995270233474624, 50.00000000000000711, -3.760136334089591248 ) ) ;
#29440=CARTESIAN_POINT ( 'NONE',  ( 12.16428377685533135, 11.73151505502934988, -9.008049429158100807 ) ) ;
#29444=CARTESIAN_POINT ( 'NONE',  ( 1.011271242968683648, 0.7347315653655930312, 3.333333333333333481 ) ) ;
#29446=B_SPLINE_CURVE_WITH_KNOTS ( 'NONE', 3,
 ( #15767, #20636, #11933, #31438 ),
 .UNSPECIFIED., .F., .F.,
 ( 4, 4 ),
 ( 0.0003850166616901197036, 0.006523527006578243477 ),
 .UNSPECIFIED. ) ;
#29448=CARTESIAN_POINT ( 'NONE',  ( -15.00099850811941948, -7.462898891544107016, 9.403735324607438884 ) ) ;
#29509=CARTESIAN_POINT ( 'NONE',  ( -1.011271242968683426, -0.7347315653655928092, 10.00000000000000000 ) ) ;
#29512=LINE ( 'NONE', #13605, #18959 ) ;
#29515=CARTESIAN_POINT ( 'NONE',  ( 0.8284317003885898201, 1.889026769141425310, 9.889206916986893248 ) ) ;
#29537=ORIENTED_EDGE ( 'NONE', *, *, #12924, .F. ) ;
#29542=ORIENTED_EDGE ( 'NONE', *, *, #24897, .T. ) ;
#29544=B_SPLINE_CURVE_WITH_KNOTS ( 'NONE', 3,
 ( #15341, #30996, #46585, #11482 ),
 .UNSPECIFIED., .F., .F.,
 ( 4, 4 ),
 ( 0.000000000000000000, 0.0001252128669263237308 ),
 .UNSPECIFIED. ) ;
#29547=B_SPLINE_CURVE_WITH_KNOTS ( 'NONE', 3,
 ( #21631, #37320, #2144, #17788 ),
 .UNSPECIFIED., .F., .F.,
 ( 4, 4 ),
 ( 0.9890644561681873892, 1.000000000000000000 ),
 .UNSPECIFIED. ) ;
#29553=ORIENTED_EDGE ( 'NONE', *, *, #24246, .F. ) ;
#29555=CARTESIAN_POINT ( 'NONE',  ( 46.11867747200574996, -19.86470446310233484, -8.016098858316199838 ) ) ;
#29558=CARTESIAN_POINT ( 'NONE',  ( 10.00000000000000000, 1.224646799147353256E-15, 0.000000000000000000 ) ) ;
#29566=CARTESIAN_POINT ( 'NONE',  ( 1.424725715586983243, -0.8249487629949646683, 9.927568724237804787 ) ) ;
#29567=CARTESIAN_POINT ( 'NONE',  ( -7.749480817862350435, -14.85497772329513211, 9.403735324607438884 ) ) ;
#29576=CARTESIAN_POINT ( 'NONE',  ( -0.3862712429686895876, 1.188820645368940720, 10.00000000000000000 ) ) ;
#29577=EDGE_CURVE ( 'NONE', #23786, #38645, #9459, .T. ) ;
#29586=CARTESIAN_POINT ( 'NONE',  ( 1.468713901642212161, 0.3220470327672588229, 9.927319414211225990 ) ) ;
#29592=CARTESIAN_POINT ( 'NONE',  ( 16.99749102614301677, -1.320765928724307425, 8.953103998512858652 ) ) ;
#29593=ORIENTED_EDGE ( 'NONE', *, *, #47857, .F. ) ;
#29595=EDGE_CURVE ( 'NONE', #36396, #9851, #38402, .T. ) ;
#29603=DIRECTION ( 'NONE',  ( 0.000000000000000000, 0.000000000000000000, -1.000000000000000000 ) ) ;
#29616=ORIENTED_EDGE ( 'NONE', *, *, #39701, .F. ) ;
#29629=ADVANCED_FACE ( 'NONE', ( #38153 ), #44112, .T. ) ;
#29631=DIRECTION ( 'NONE',  ( 0.4374820812098791922, 0.3178493372392781069, 0.8411784753765542133 ) ) ;
#29634=CARTESIAN_POINT ( 'NONE',  ( -37.09503908879538159, 5.733418411339063603, 4.835783797351798086 ) ) ;
#29637=EDGE_CURVE ( 'NONE', #6876, #35009, #7009, .T. ) ;
#29649=CARTESIAN_POINT ( 'NONE',  ( -30.77287599203642188, -12.70002479445974686, 3.199614146704519602 ) ) ;
#29656=CARTESIAN_POINT ( 'NONE',  ( 1.780432407520001536, 1.041450996408479046, 9.894754715216729224 ) ) ;
#29658=EDGE_CURVE ( 'NONE', #36434, #28673, #48529, .T. ) ;
#29659=CARTESIAN_POINT ( 'NONE',  ( 0.3370904143228947158, 0.2449105217885311492, 10.00000000000000000 ) ) ;
#29664=ORIENTED_EDGE ( 'NONE', *, *, #26185, .T. ) ;
#29668=CARTESIAN_POINT ( 'NONE',  ( 36.80807479611532784, -7.357694319819502837, 1.982731392810463067 ) ) ;
#29679=CARTESIAN_POINT ( 'NONE',  ( 0.9983599181300923942, 1.124146016603553733, 9.953784399990620813 ) ) ;
#29684=CARTESIAN_POINT ( 'NONE',  ( 2.052581215100350853, -0.2042358160480859663, 9.886433018048069954 ) ) ;
#29687=LINE ( 'NONE', #17876, #11005 ) ;
#29692=CARTESIAN_POINT ( 'NONE',  ( 1.211301556933464862, 0.1727733738854638212, 9.993783931180534097 ) ) ;
#29700=DIRECTION ( 'NONE',  ( 0.000000000000000000, 0.000000000000000000, 1.000000000000000000 ) ) ;
#29702=ADVANCED_FACE ( 'NONE', ( #35074 ), #20776, .T. ) ;
#29704=CARTESIAN_POINT ( 'NONE',  ( -4.353119224255007857, -9.002796955359011477, 0.000000000000000000 ) ) ;
#29709=VECTOR ( 'NONE', #6888, 1000.000000000000000 ) ;
#29719=B_SPLINE_SURFACE_WITH_KNOTS ( 'NONE', 3, 3, ( 
 ( #40143, #16539, #16789, #44218 ),
 ( #47789, #20885, #1649, #48290 ),
 ( #40889, #4978, #24999, #44715 ),
 ( #40400, #17290, #12676, #43968 ) ),
 .UNSPECIFIED., .F., .F., .F.,
 ( 4, 4 ),
 ( 4, 4 ),
 ( 0.000000000000000000, 1.000000000000000000 ),
 ( 0.000000000000000000, 1.000000000000000000 ),
 .UNSPECIFIED. ) ;
#29721=EDGE_LOOP ( 'NONE', ( #19883, #39954, #38920, #39317 ) ) ;
#29730=CARTESIAN_POINT ( 'NONE',  ( 3.808200756227633654, 0.8261963378076531139, 9.741991644047248045 ) ) ;
#29743=CARTESIAN_POINT ( 'NONE',  ( -1.011271242968693862, 0.7347315653655780432, -10.00000000000000000 ) ) ;
#29759=CARTESIAN_POINT ( 'NONE',  ( -36.28567981536816234, -9.465698090293395595, -9.422646554964174470 ) ) ;
#29766=CARTESIAN_POINT ( 'NONE',  ( -36.63544619771738553, -20.34968343020614512, 7.544061037322998153 ) ) ;
#29770=EDGE_CURVE ( 'NONE', #21356, #1069, #3917, .T. ) ;
#29779=CARTESIAN_POINT ( 'NONE',  ( 1.249999999999999778, 0.000000000000000000, 9.972675548442463622 ) ) ;
#29784=VERTEX_POINT ( 'NONE', #17499 ) ;
#29793=DIRECTION ( 'NONE',  ( 0.6805276818820402696, 0.4944323023722069221, 0.5407575913134970991 ) ) ;
#29795=VERTEX_POINT ( 'NONE', #14137 ) ;
#29798=CARTESIAN_POINT ( 'NONE',  ( 5.083187235775197266, 8.611690166631179366, 9.646707543097347681 ) ) ;
#29801=CARTESIAN_POINT ( 'NONE',  ( 1.468713901642212161, 0.3220470327672588229, 9.927319414211225990 ) ) ;
#29802=B_SPLINE_CURVE_WITH_KNOTS ( 'NONE', 3,
 ( #31871, #46699, #26988, #7503 ),
 .UNSPECIFIED., .F., .F.,
 ( 4, 4 ),
 ( 0.000000000000000000, 0.002466147708923230146 ),
 .UNSPECIFIED. ) ;
#29819=VERTEX_POINT ( 'NONE', #40019 ) ;
#29824=CARTESIAN_POINT ( 'NONE',  ( 6.619412807845094449, -7.495556955913033725, 9.646707543097347681 ) ) ;
#29826=CARTESIAN_POINT ( 'NONE',  ( 1.011271242968688311, -0.7347315653655855927, 10.00000000000000000 ) ) ;
#29834=CARTESIAN_POINT ( 'NONE',  ( 0.09523839817332763191, 1.466467394239034050, 9.958264684458713489 ) ) ;
#29836=CARTESIAN_POINT ( 'NONE',  ( 49.89397392339123627, -8.245536726716670373, 7.906207997025717304 ) ) ;
#29837=EDGE_LOOP ( 'NONE', ( #25452, #39224, #39917, #1144, #7462 ) ) ;
#29838=CARTESIAN_POINT ( 'NONE',  ( -30.22736451279196856, -39.84193304692609416, -2.408242355805840784 ) ) ;
#29841=B_SPLINE_CURVE_WITH_KNOTS ( 'NONE', 3,
 ( #37469, #18434, #22543, #42300 ),
 .UNSPECIFIED., .F., .F.,
 ( 4, 4 ),
 ( 0.000000000000000000, 0.2637263876330691592 ),
 .UNSPECIFIED. ) ;
#29842=DIRECTION ( 'NONE',  ( 0.6805276818820432672, -0.4944323023722019261, -0.5407575913134976542 ) ) ;
#29843=CARTESIAN_POINT ( 'NONE',  ( 1.468535767197692188, 0.3224370614409108327, 9.944962737616616977 ) ) ;
#29851=CARTESIAN_POINT ( 'NONE',  ( 0.1287570809895575430, 0.3962735484563150168, 10.00000000000000000 ) ) ;
#29881=CARTESIAN_POINT ( 'NONE',  ( -0.9300423221600405688, -1.714483250866335240, 9.896382706792437034 ) ) ;
#29885=VERTEX_POINT ( 'NONE', #20254 ) ;
#29889=CARTESIAN_POINT ( 'NONE',  ( -31.28977333267361871, 11.25592690310926969, -2.408242355805840784 ) ) ;
#29892=CARTESIAN_POINT ( 'NONE',  ( -1.721971274562257515, -0.09408549481333014497, 9.928159647716187308 ) ) ;
#29895=CARTESIAN_POINT ( 'NONE',  ( 3.229232847726260403, -16.57333684275945629, 9.178419661560148768 ) ) ;
#29898=CARTESIAN_POINT ( 'NONE',  ( 15.57957361750251302, 5.755602074545510760, 3.266473740018926541 ) ) ;
#29902=CARTESIAN_POINT ( 'NONE',  ( 9.760995290733820440, -2.173239732351728293, 9.646707543097347681 ) ) ;
#29904=FACE_OUTER_BOUND ( 'NONE', #9350, .T. ) ;
#29906=CARTESIAN_POINT ( 'NONE',  ( 0.3370904143228959926, -0.2449105217885284291, 10.00000000000000000 ) ) ;
#29913=ORIENTED_EDGE ( 'NONE', *, *, #19025, .T. ) ;
#29919=ORIENTED_EDGE ( 'NONE', *, *, #8703, .T. ) ;
#29926=CARTESIAN_POINT ( 'NONE',  ( 16.99749102614301677, -1.320765928724307425, 8.953103998512858652 ) ) ;
#29928=EDGE_CURVE ( 'NONE', #36961, #31206, #31467, .T. ) ;
#29931=CARTESIAN_POINT ( 'NONE',  ( 1.249999999999999778, 0.000000000000000000, 10.00000000000000000 ) ) ;
#29938=CARTESIAN_POINT ( 'NONE',  ( -30.87089393895367095, 12.69923079256638587, -9.367992836599954742 ) ) ;
#29947=PLANE ( 'NONE',  #34769 ) ;
#29950=CARTESIAN_POINT ( 'NONE',  ( -1.011271242968677875, -0.7347315653656004697, 3.333333333333333481 ) ) ;
#29956=LINE ( 'NONE', #25103, #41076 ) ;
#29964=CARTESIAN_POINT ( 'NONE',  ( -36.97942854200451990, 6.226705766838657397, 8.914903342594564961 ) ) ;
#29965=VECTOR ( 'NONE', #29631, 1000.000000000000114 ) ;
#29966=CARTESIAN_POINT ( 'NONE',  ( 0.2776613828612440882, -1.251395203515894172, 9.967237415621763574 ) ) ;
#29976=EDGE_LOOP ( 'NONE', ( #32718, #30577, #763, #38641, #47556 ) ) ;
#29978=ORIENTED_EDGE ( 'NONE', *, *, #4497, .F. ) ;
#29984=CARTESIAN_POINT ( 'NONE',  ( -0.3862712429686809279, -1.188820645368943163, 10.00000000000000000 ) ) ;
#29987=CARTESIAN_POINT ( 'NONE',  ( 29.61572577327002520, 16.11461842845735859, 8.807470649214879543 ) ) ;
#29990=CARTESIAN_POINT ( 'NONE',  ( 0.3910393408562611861, 3.877122853646846945, 9.741991644046958498 ) ) ;
#29992=CARTESIAN_POINT ( 'NONE',  ( 34.95136153415558056, -36.40974830873469870, 8.356839323120299312 ) ) ;
#30002=CIRCLE ( 'NONE', #7887, 37.50000000000000000 ) ;
#30012=ADVANCED_FACE ( 'NONE', ( #48939 ), #22045, .F. ) ;
#30017=CARTESIAN_POINT ( 'NONE',  ( 6.429410166934437676, 2.386389549874229132, 9.753789706659947711 ) ) ;
#30020=CARTESIAN_POINT ( 'NONE',  ( -8.831420117243776957, -14.12636088103186260, -3.546734833711462365 ) ) ;
#30021=ORIENTED_EDGE ( 'NONE', *, *, #3633, .T. ) ;
#30024=CARTESIAN_POINT ( 'NONE',  ( 28.55116071645549525, -41.05976639056858346, -2.408242355805840784 ) ) ;
#30030=CARTESIAN_POINT ( 'NONE',  ( -2.391286777839504385, 5.398370916126228103, 9.586754400233969520 ) ) ;
#30031=EDGE_LOOP ( 'NONE', ( #29616, #24385, #17304, #9115 ) ) ;
#30033=CARTESIAN_POINT ( 'NONE',  ( 24.39427009665985224, 44.07992421011656603, 8.807470649214879543 ) ) ;
#30045=VERTEX_POINT ( 'NONE', #21802 ) ;
#30055=CARTESIAN_POINT ( 'NONE',  ( -1.873480598308069123, 3.275918692700744206, 9.865049507598756762 ) ) ;
#30060=ORIENTED_EDGE ( 'NONE', *, *, #6986, .F. ) ;
#30080=CARTESIAN_POINT ( 'NONE',  ( 26.18032376592674737, -21.95228666728361233, 7.455576670931136185 ) ) ;
#30085=CARTESIAN_POINT ( 'NONE',  ( 6.219530239386670267, -7.848697864701615678, 6.429802539306459508 ) ) ;
#30100=LINE ( 'NONE', #37812, #42629 ) ;
#30101=CARTESIAN_POINT ( 'NONE',  ( 1.326845121651809789, -0.3624933883365012988, 9.972175347158398040 ) ) ;
#30121=FACE_OUTER_BOUND ( 'NONE', #23184, .T. ) ;
#30122=ORIENTED_EDGE ( 'NONE', *, *, #37837, .F. ) ;
#30126=ADVANCED_FACE ( 'NONE', ( #15110 ), #16674, .T. ) ;
#30132=CARTESIAN_POINT ( 'NONE',  ( -2.769930902779030646, 9.621092503091231762, 6.185716040203081079 ) ) ;
#30136=B_SPLINE_CURVE_WITH_KNOTS ( 'NONE', 3,
 ( #30422, #19626, #11425, #27331 ),
 .UNSPECIFIED., .F., .F.,
 ( 4, 4 ),
 ( 0.8097120833243712790, 0.9322955464062560038 ),
 .UNSPECIFIED. ) ;
#30138=FACE_OUTER_BOUND ( 'NONE', #16151, .T. ) ;
#30153=CARTESIAN_POINT ( 'NONE',  ( 32.57680531928920686, 38.13496438397469035, -8.466730184410787174 ) ) ;
#30156=CARTESIAN_POINT ( 'NONE',  ( 0.1475726264153646716, 1.496347932843221429, 9.927319414211224213 ) ) ;
#30164=CARTESIAN_POINT ( 'NONE',  ( -12.97493236725075683, 11.05939663307000664, 8.953103998512858652 ) ) ;
#30172=CARTESIAN_POINT ( 'NONE',  ( -16.07893968642797233, -33.88550589494182930, 8.100132398494514163 ) ) ;
#30180=EDGE_CURVE ( 'NONE', #21718, #34526, #30828, .T. ) ;
#30181=CARTESIAN_POINT ( 'NONE',  ( 1.224655226406667019, 1.100228625579998010, 9.936700280135880803 ) ) ;
#30196=CARTESIAN_POINT ( 'NONE',  ( -34.94239438780405749, -13.71128139791396272, 3.209567239418968487 ) ) ;
#30199=CARTESIAN_POINT ( 'NONE',  ( 48.98697415750968531, 11.03699497439252575, -8.016098858316205167 ) ) ;
#30202=CARTESIAN_POINT ( 'NONE',  ( 33.16902712922644270, -37.70469005304286725, 1.847720168420772691 ) ) ;
#30222=CARTESIAN_POINT ( 'NONE',  ( -5.923309609702550382, 5.336940278790372361, -7.724940478959219092E-16 ) ) ;
#30248=VERTEX_POINT ( 'NONE', #8692 ) ;
#30251=CARTESIAN_POINT ( 'NONE',  ( 5.888214538810389698, 16.20866436362417673, 8.727788335465566760 ) ) ;
#30259=CARTESIAN_POINT ( 'NONE',  ( -9.174209336589896679, -3.979181203266159095, 9.646707543097347681 ) ) ;
#30261=CARTESIAN_POINT ( 'NONE',  ( -0.7606162131530730397, 1.296876929034918691, 9.953784399990622589 ) ) ;
#30268=CARTESIAN_POINT ( 'NONE',  ( 1.114871695981101585, -0.4953159757246433093, 9.963925895596188909 ) ) ;
#30271=CARTESIAN_POINT ( 'NONE',  ( 8.864235763825218939, 4.693841405978110615, 9.516222621873129839 ) ) ;
#30275=CARTESIAN_POINT ( 'NONE',  ( 46.76852358249013975, -17.86468378716709537, -9.367992836599954742 ) ) ;
#30281=EDGE_CURVE ( 'NONE', #37687, #12617, #24110, .T. ) ;
#30289=ORIENTED_EDGE ( 'NONE', *, *, #12886, .T. ) ;
#30306=EDGE_CURVE ( 'NONE', #39166, #76, #7563, .T. ) ;
#30307=CARTESIAN_POINT ( 'NONE',  ( 29.38926261462401257, -40.45084971874711499, 0.000000000000000000 ) ) ;
#30308=CARTESIAN_POINT ( 'NONE',  ( 0.2553279260466790879, -1.933711247496585184, 9.896382706792378414 ) ) ;
#30316=CARTESIAN_POINT ( 'NONE',  ( 12.97493236725083676, -11.05939663306990717, 8.953103998512858652 ) ) ;
#30322=CARTESIAN_POINT ( 'NONE',  ( -12.35406723005387875, 11.51001571518090039, 9.178419661560148768 ) ) ;
#30326=VERTEX_POINT ( 'NONE', #6589 ) ;
#30332=CARTESIAN_POINT ( 'NONE',  ( 12.78770032058947237, 31.68259716188277864, 7.455576670931136185 ) ) ;
#30333=ORIENTED_EDGE ( 'NONE', *, *, #43147, .F. ) ;
#30335=CARTESIAN_POINT ( 'NONE',  ( -31.94178169330213279, 9.256608784834037706, -3.760136334089591248 ) ) ;
#30352=CARTESIAN_POINT ( 'NONE',  ( 7.398363427652524749, -15.19415887381133246, -9.008049429158102583 ) ) ;
#30358=CARTESIAN_POINT ( 'NONE',  ( 28.96803024440893992, 18.11533787072037072, 7.455576670931136185 ) ) ;
#30364=CARTESIAN_POINT ( 'NONE',  ( -25.40454589245989325, -27.58367357691681931, -8.192531242611266862 ) ) ;
#30367=ORIENTED_EDGE ( 'NONE', *, *, #13142, .F. ) ;
#30369=CARTESIAN_POINT ( 'NONE',  ( 2.134702841136851603, 5.564253780994583565, -8.944667923005411581E-16 ) ) ;
#30376=CARTESIAN_POINT ( 'NONE',  ( -46.10908423965022251, -19.89422939639105437, 1.847720168420772691 ) ) ;
#30384=CARTESIAN_POINT ( 'NONE',  ( 1.193089574352119264, 0.2545860991493882342, 9.963925895596188909 ) ) ;
#30386=CARTESIAN_POINT ( 'NONE',  ( -29.39982726364978660, -16.78152490921149109, 8.356839323120299312 ) ) ;
#30387=ORIENTED_EDGE ( 'NONE', *, *, #16580, .F. ) ;
#30388=CARTESIAN_POINT ( 'NONE',  ( 0.8965959638259385356, 1.582931917743541028, 9.903764339332076005 ) ) ;
#30392=FACE_OUTER_BOUND ( 'NONE', #48927, .T. ) ;
#30395=CARTESIAN_POINT ( 'NONE',  ( -16.16402646813540755, 4.033894069732547827, -3.546734833711462365 ) ) ;
#30414=EDGE_CURVE ( 'NONE', #42350, #45889, #45510, .T. ) ;
#30416=CARTESIAN_POINT ( 'NONE',  ( -0.9599924130074112272, 0.8495346730527952861, 9.948547179989619238 ) ) ;
#30420=ORIENTED_EDGE ( 'NONE', *, *, #24236, .T. ) ;
#30422=CARTESIAN_POINT ( 'NONE',  ( -8.001683061421429599, -5.997755262142646870, 9.282506307616484875 ) ) ;
#30425=CARTESIAN_POINT ( 'NONE',  ( 0.5107275442771160856, 1.175643901748075537, 9.976582533991678048 ) ) ;
#30433=ORIENTED_EDGE ( 'NONE', *, *, #45517, .F. ) ;
#30434=CARTESIAN_POINT ( 'NONE',  ( -34.91952936320829792, 13.67027684621028349, -9.422646554964178023 ) ) ;
#30437=ORIENTED_EDGE ( 'NONE', *, *, #41290, .F. ) ;
#30461=CARTESIAN_POINT ( 'NONE',  ( 17.51065725283126895, -28.41934970907778890, -9.367992836599954742 ) ) ;
#30462=CARTESIAN_POINT ( 'NONE',  ( -14.29087950072019098, -9.652079258044555132, 8.727788335465566760 ) ) ;
#30469=CARTESIAN_POINT ( 'NONE',  ( 1.411185367335151541, 16.64174154430383012, -9.458680755252684591 ) ) ;
#30476=ORIENTED_EDGE ( 'NONE', *, *, #11819, .F. ) ;
#30488=CARTESIAN_POINT ( 'NONE',  ( -0.9602803029231570253, 0.8490247040095960651, 9.976582533991679824 ) ) ;
#30510=CARTESIAN_POINT ( 'NONE',  ( 24.47767542868285062, -23.18653802921781448, 8.807470649214879543 ) ) ;
#30513=CARTESIAN_POINT ( 'NONE',  ( -12.78770032058971395, -31.68259716188267916, 7.455576670931136185 ) ) ;
#30518=AXIS2_PLACEMENT_3D ( 'NONE', #9848, #29603, #30818 ) ;
#30522=CARTESIAN_POINT ( 'NONE',  ( -24.39427009666018265, -44.07992421011638129, 8.807470649214879543 ) ) ;
#30524=B_SPLINE_CURVE_WITH_KNOTS ( 'NONE', 3,
 ( #32638, #32130, #12615, #43915 ),
 .UNSPECIFIED., .F., .F.,
 ( 4, 4 ),
 ( 0.001403500796105004635, 0.001586656765099030445 ),
 .UNSPECIFIED. ) ;
#30526=CARTESIAN_POINT ( 'NONE',  ( 33.01266944765062306, -5.813986777101467496, 1.847720168420772691 ) ) ;
#30527=CARTESIAN_POINT ( 'NONE',  ( -8.277096487746778308, 33.14818118907697198, 7.455576670931136185 ) ) ;
#30534=CARTESIAN_POINT ( 'NONE',  ( 17.23491422248386584, -0.5912720620000816441, 8.727788335465566760 ) ) ;
#30553=DIRECTION ( 'NONE',  ( -1.000000000000000000, 0.000000000000000000, 0.000000000000000000 ) ) ;
#30556=CARTESIAN_POINT ( 'NONE',  ( 1.133908876584335257, 0.5183204401656757998, 9.981352469109932457 ) ) ;
#30563=ORIENTED_EDGE ( 'NONE', *, *, #6602, .F. ) ;
#30566=B_SPLINE_SURFACE_WITH_KNOTS ( 'NONE', 3, 3, ( 
 ( #43460, #15501, #31171, #46759 ),
 ( #35283, #11661, #27314, #24481 ),
 ( #24985, #21118, #36552, #44699 ),
 ( #44941, #20870, #17279, #29576 ) ),
 .UNSPECIFIED., .F., .F., .F.,
 ( 4, 4 ),
 ( 4, 4 ),
 ( 0.000000000000000000, 1.000000000000000000 ),
 ( 0.000000000000000000, 1.000000000000000000 ),
 .UNSPECIFIED. ) ;
#30574=EDGE_CURVE ( 'NONE', #48305, #30605, #50297, .T. ) ;
#30577=ORIENTED_EDGE ( 'NONE', *, *, #27779, .F. ) ;
#30590=CARTESIAN_POINT ( 'NONE',  ( -0.3862712429686729343, -1.188820645368946050, 3.333333333333333481 ) ) ;
#30592=CARTESIAN_POINT ( 'NONE',  ( -0.3862712429686809279, -1.188820645368943163, -3.333333333333333481 ) ) ;
#30593=CARTESIAN_POINT ( 'NONE',  ( -0.2257686176856275040, 1.281370980887437838, 9.986087673579199020 ) ) ;
#30599=VECTOR ( 'NONE', #10398, 1000.000000000000000 ) ;
#30600=CARTESIAN_POINT ( 'NONE',  ( 7.129058724844953510, 15.30620660340485095, 9.178419661560148768 ) ) ;
#30605=VERTEX_POINT ( 'NONE', #48327 ) ;
#30610=CARTESIAN_POINT ( 'NONE',  ( 1.275994128725544741, -0.1230186051320594776, 9.948547179989619238 ) ) ;
#30613=LINE ( 'NONE', #42647, #13555 ) ;
#30617=CARTESIAN_POINT ( 'NONE',  ( -6.408332700304190332, -7.676800896350769676, 0.000000000000000000 ) ) ;
#30625=EDGE_CURVE ( 'NONE', #41656, #14966, #16098, .T. ) ;
#30644=B_SPLINE_CURVE_WITH_KNOTS ( 'NONE', 3,
 ( #41230, #1248, #21231, #44546 ),
 .UNSPECIFIED., .F., .F.,
 ( 4, 4 ),
 ( 0.000000000000000000, 0.2545280377015989859 ),
 .UNSPECIFIED. ) ;
#30645=ORIENTED_EDGE ( 'NONE', *, *, #10801, .F. ) ;
#30647=CARTESIAN_POINT ( 'NONE',  ( 0.000000000000000000, 0.000000000000000000, 10.00000000000000000 ) ) ;
#30652=CARTESIAN_POINT ( 'NONE',  ( 5.888214538810389698, 16.20866436362417673, 8.727788335465566760 ) ) ;
#30677=B_SPLINE_SURFACE_WITH_KNOTS ( 'NONE', 3, 3, ( 
 ( #36096, #40438, #938, #9879 ),
 ( #17582, #9129, #9380, #6026 ),
 ( #44761, #24791, #40693, #33256 ),
 ( #32237, #24533, #20931, #48837 ) ),
 .UNSPECIFIED., .F., .F., .F.,
 ( 4, 4 ),
 ( 4, 4 ),
 ( 0.000000000000000000, 1.000000000000000000 ),
 ( 0.000000000000000000, 1.000000000000000000 ),
 .UNSPECIFIED. ) ;
#30681=CARTESIAN_POINT ( 'NONE',  ( 6.174150299305392053, -50.00000000000000711, 8.807470649214879543 ) ) ;
#30705=EDGE_CURVE ( 'NONE', #21132, #10463, #44781, .T. ) ;
#30714=CARTESIAN_POINT ( 'NONE',  ( -1.035950918207909632, -50.00000000000000711, -2.408242355805840784 ) ) ;
#30726=CARTESIAN_POINT ( 'NONE',  ( 20.40054609052976531, -26.26366202847973597, -3.760136334089591248 ) ) ;
#30729=VERTEX_POINT ( 'NONE', #18314 ) ;
#30738=ORIENTED_EDGE ( 'NONE', *, *, #28369, .T. ) ;
#30739=CARTESIAN_POINT ( 'NONE',  ( -1.011271242968688533, 0.7347315653655859258, -10.00000000000000000 ) ) ;
#30740=ORIENTED_EDGE ( 'NONE', *, *, #22443, .T. ) ;
#30743=B_SPLINE_CURVE_WITH_KNOTS ( 'NONE', 3,
 ( #35656, #19968, #31543, #41167 ),
 .UNSPECIFIED., .F., .F.,
 ( 4, 4 ),
 ( 0.000000000000000000, 0.0002520763768929746781 ),
 .UNSPECIFIED. ) ;
#30749=CARTESIAN_POINT ( 'NONE',  ( 36.28567981536807707, 9.465698090293649614, -9.422646554964174470 ) ) ;
#30755=AXIS2_PLACEMENT_3D ( 'NONE', #24547, #20188, #8656 ) ;
#30757=CARTESIAN_POINT ( 'NONE',  ( -8.001683061421429599, -5.997755262142646870, 9.282506307616484875 ) ) ;
#30767=CARTESIAN_POINT ( 'NONE',  ( -1.249999999999999778, 0.000000000000000000, -10.00000000000000000 ) ) ;
#30770=CARTESIAN_POINT ( 'NONE',  ( -3.996390545799824334, 16.57371371864897469, 8.953103998512858652 ) ) ;
#30788=CARTESIAN_POINT ( 'NONE',  ( -27.31081730472607561, -41.96092862852123773, 3.199614146704519602 ) ) ;
#30790=CARTESIAN_POINT ( 'NONE',  ( 1.655083087279030529, -7.799304763725482204, 1.626303258728256651E-16 ) ) ;
#30797=CARTESIAN_POINT ( 'NONE',  ( 0.3862712429686727678, 1.188820645368945605, 10.00000000000000000 ) ) ;
#30805=VERTEX_POINT ( 'NONE', #37103 ) ;
#30811=CARTESIAN_POINT ( 'NONE',  ( -17.51065725283106289, 28.41934970907792746, -9.367992836599954742 ) ) ;
#30818=DIRECTION ( 'NONE',  ( -1.000000000000000000, 0.000000000000000000, -0.000000000000000000 ) ) ;
#30822=CARTESIAN_POINT ( 'NONE',  ( -9.563755223200868016, -2.971660568388000634, 3.215106848023638886 ) ) ;
#30824=CARTESIAN_POINT ( 'NONE',  ( 1.317555876316863994, 0.4584864758885041081, 9.955131761384825140 ) ) ;
#30826=CARTESIAN_POINT ( 'NONE',  ( 34.38425513258721367, -36.82177522737820397, 8.807470649214879543 ) ) ;
#30828=B_SPLINE_CURVE_WITH_KNOTS ( 'NONE', 3,
 ( #23052, #3545, #46619, #19194 ),
 .UNSPECIFIED., .F., .F.,
 ( 4, 4 ),
 ( 0.000000000000000000, 0.0003726855806051463586 ),
 .UNSPECIFIED. ) ;
#30835=CARTESIAN_POINT ( 'NONE',  ( 0.3370904143228959926, -0.2449105217885284291, 10.00000000000000000 ) ) ;
#30842=ADVANCED_FACE ( 'NONE', ( #30138 ), #33747, .F. ) ;
#30851=CARTESIAN_POINT ( 'NONE',  ( 15.73090589902275482, 29.60029367929053024, 1.847720168420772691 ) ) ;
#30869=ADVANCED_FACE ( 'NONE', ( #6784 ), #20360, .T. ) ;
#30873=DIRECTION ( 'NONE',  ( 0.1671032855531282557, 0.5142910309547750192, 0.8411784753765542133 ) ) ;
#30874=VECTOR ( 'NONE', #29181, 1000.000000000000000 ) ;
#30882=ADVANCED_FACE ( 'NONE', ( #11652 ), #39204, .T. ) ;
#30883=ORIENTED_EDGE ( 'NONE', *, *, #31938, .F. ) ;
#30888=EDGE_LOOP ( 'NONE', ( #8565, #8884, #26950, #32641 ) ) ;
#30889=CARTESIAN_POINT ( 'NONE',  ( 35.35872492446288362, -12.59883863067502929, -2.490396854064191423 ) ) ;
#30894=CARTESIAN_POINT ( 'NONE',  ( -47.22310614333779455, -16.46562252335923660, -3.760136334089591248 ) ) ;
#30898=CARTESIAN_POINT ( 'NONE',  ( 8.277096487746778308, -33.14818118907697198, 7.455576670931136185 ) ) ;
#30907=CARTESIAN_POINT ( 'NONE',  ( -15.42815683172655028, -34.17926237904570996, 7.697694107796190899 ) ) ;
#30916=CARTESIAN_POINT ( 'NONE',  ( -0.3862712429686809279, -1.188820645368943163, -3.333333333333333481 ) ) ;
#30921=VERTEX_POINT ( 'NONE', #8567 ) ;
#30927=CARTESIAN_POINT ( 'NONE',  ( -2.216591765714429396, 1.436486588196063119, 9.847478953136933555 ) ) ;
#30930=CARTESIAN_POINT ( 'NONE',  ( -14.29087950072019098, -9.652079258044555132, 8.727788335465566760 ) ) ;
#30941=EDGE_CURVE ( 'NONE', #42239, #41021, #10539, .T. ) ;
#30944=CARTESIAN_POINT ( 'NONE',  ( 8.001683061421385190, 5.997755262142701937, 9.282506307616484875 ) ) ;
#30946=CARTESIAN_POINT ( 'NONE',  ( 6.875132362119187768, -33.14667368551891258, 8.356839323120299312 ) ) ;
#30950=CARTESIAN_POINT ( 'NONE',  ( 14.76429217231961566, 8.192625680377691566, 9.178419661560148768 ) ) ;
#30951=CARTESIAN_POINT ( 'NONE',  ( -6.174150299305392053, 50.00000000000000711, 8.807470649214879543 ) ) ;
#30958=CARTESIAN_POINT ( 'NONE',  ( 6.408332700304398166, 7.676800896350598258, 0.000000000000000000 ) ) ;
#30961=CARTESIAN_POINT ( 'NONE',  ( 18.37190376999591024, 32.73290680288470611, 1.982731392810408444 ) ) ;
#30962=EDGE_LOOP ( 'NONE', ( #50393, #21665, #21434, #29342 ) ) ;
#30963=ORIENTED_EDGE ( 'NONE', *, *, #38474, .F. ) ;
#30980=CARTESIAN_POINT ( 'NONE',  ( 32.65539107884896453, 7.204654279306055287, -8.917361510505369182 ) ) ;
#30984=CARTESIAN_POINT ( 'NONE',  ( 1.249999999999999778, 0.000000000000000000, 10.00000000000000000 ) ) ;
#30987=CARTESIAN_POINT ( 'NONE',  ( -0.8784099037133121790, -0.8517617868932445546, 9.993783931180535873 ) ) ;
#30996=CARTESIAN_POINT ( 'NONE',  ( -0.9772698688233778519, 0.8109225331901841471, 9.975314328424618182 ) ) ;
#30999=CARTESIAN_POINT ( 'NONE',  ( -20.37409433808010562, -26.28007012093468475, -2.408242355805840784 ) ) ;
#31000=B_SPLINE_SURFACE_WITH_KNOTS ( 'NONE', 3, 3, ( 
 ( #42381, #26492, #35221, #42633 ),
 ( #15203, #34980, #30600, #11345 ),
 ( #50546, #6991, #7766, #65 ),
 ( #50292, #50034, #34455, #7244 ) ),
 .UNSPECIFIED., .F., .F., .F.,
 ( 4, 4 ),
 ( 4, 4 ),
 ( 0.000000000000000000, 1.000000000000000000 ),
 ( 0.000000000000000000, 1.000000000000000000 ),
 .UNSPECIFIED. ) ;
#31013=CARTESIAN_POINT ( 'NONE',  ( -34.66007756064415446, 14.33302383662612556, -9.011255500499645521 ) ) ;
#31017=CARTESIAN_POINT ( 'NONE',  ( 0.9772698688233751874, -0.8109225331901837031, 9.975314328424616406 ) ) ;
#31024=CARTESIAN_POINT ( 'NONE',  ( -36.08557433729205144, 35.58569447144795816, 7.455576670931136185 ) ) ;
#31026=CARTESIAN_POINT ( 'NONE',  ( -28.96803024440907137, -18.11533787072017176, 7.455576670931136185 ) ) ;
#31031=FACE_OUTER_BOUND ( 'NONE', #35409, .T. ) ;
#31042=DIRECTION ( 'NONE',  ( 1.000000000000000000, 0.000000000000000000, 0.000000000000000000 ) ) ;
#31043=FACE_OUTER_BOUND ( 'NONE', #10621, .T. ) ;
#31050=FACE_OUTER_BOUND ( 'NONE', #30888, .T. ) ;
#31056=VERTEX_POINT ( 'NONE', #49271 ) ;
#31062=ORIENTED_EDGE ( 'NONE', *, *, #47865, .F. ) ;
#31070=CARTESIAN_POINT ( 'NONE',  ( 37.52258785160491783, 18.42740426802386722, 8.846626183609803462 ) ) ;
#31071=CARTESIAN_POINT ( 'NONE',  ( -26.64049824243113918, 26.44234984024230073, 4.835783797351798086 ) ) ;
#31073=CARTESIAN_POINT ( 'NONE',  ( 1.721971274562253740, 0.09408549481334846365, 9.928159647716247704 ) ) ;
#31080=CARTESIAN_POINT ( 'NONE',  ( 0.5107275442771160856, 1.175643901748075537, 9.976582533991678048 ) ) ;
#31096=CARTESIAN_POINT ( 'NONE',  ( 41.59994237955810803, -5.070535260985374215, 7.544061037322996377 ) ) ;
#31104=CARTESIAN_POINT ( 'NONE',  ( -14.48769039275601145, -30.44468701195584970, 8.807470649214879543 ) ) ;
#31105=ORIENTED_EDGE ( 'NONE', *, *, #33791, .T. ) ;
#31121=EDGE_CURVE ( 'NONE', #42239, #13694, #17888, .T. ) ;
#31127=CARTESIAN_POINT ( 'NONE',  ( 0.4426377647354858835, 1.666766018367784596, 9.928159647716132241 ) ) ;
#31134=EDGE_LOOP ( 'NONE', ( #44125, #22361, #10381 ) ) ;
#31144=ORIENTED_EDGE ( 'NONE', *, *, #16711, .F. ) ;
#31151=CARTESIAN_POINT ( 'NONE',  ( 0.8282505383454039638, 1.889063466747038289, 9.894754715216722118 ) ) ;
#31155=VERTEX_POINT ( 'NONE', #496 ) ;
#31156=DIRECTION ( 'NONE',  ( -1.000000000000000000, 0.000000000000000000, 0.000000000000000000 ) ) ;
#31161=CARTESIAN_POINT ( 'NONE',  ( 0.3370904143228981575, -0.2449105217885261532, 10.00000000000000000 ) ) ;
#31164=CARTESIAN_POINT ( 'NONE',  ( 8.277096487746778308, -33.14818118907697198, 7.455576670931136185 ) ) ;
#31167=CARTESIAN_POINT ( 'NONE',  ( -1.228394325311288560, 1.341866297401936636, 9.903764339332077782 ) ) ;
#31171=CARTESIAN_POINT ( 'NONE',  ( -16.73672383626882976, -2.341008440547994063, -9.008049429158100807 ) ) ;
#31173=CARTESIAN_POINT ( 'NONE',  ( -16.99749102614300966, 1.320765928724422222, 8.953103998512858652 ) ) ;
#31179=B_SPLINE_CURVE_WITH_KNOTS ( 'NONE', 3,
 ( #44509, #24795, #6035, #37376 ),
 .UNSPECIFIED., .F., .F.,
 ( 4, 4 ),
 ( 0.0004299334430849653297, 0.0007706806524480538500 ),
 .UNSPECIFIED. ) ;
#31182=EDGE_CURVE ( 'NONE', #14966, #23429, #6913, .T. ) ;
#31195=ORIENTED_EDGE ( 'NONE', *, *, #16147, .F. ) ;
#31196=CARTESIAN_POINT ( 'NONE',  ( -2.462075149652696027, 16.57295996686994499, 9.403735324607438884 ) ) ;
#31201=ORIENTED_EDGE ( 'NONE', *, *, #44153, .T. ) ;
#31202=VECTOR ( 'NONE', #12446, 999.9999999999998863 ) ;
#31205=CARTESIAN_POINT ( 'NONE',  ( 1.320835335343329753, -0.01943189459118491516, 9.943883492372847854 ) ) ;
#31206=VERTEX_POINT ( 'NONE', #26737 ) ;
#31207=CARTESIAN_POINT ( 'NONE',  ( 1.066995270233474624, -50.00000000000000711, -3.760136334089591248 ) ) ;
#31217=EDGE_CURVE ( 'NONE', #7144, #45646, #42976, .T. ) ;
#31219=CARTESIAN_POINT ( 'NONE',  ( 32.43949840348898306, 7.871562655726499713, -9.367992836599954742 ) ) ;
#31229=EDGE_CURVE ( 'NONE', #22165, #13210, #50193, .T. ) ;
#31240=CARTESIAN_POINT ( 'NONE',  ( -0.9989200098981521059, -1.123829893718962802, 9.927319414211225990 ) ) ;
#31252=CARTESIAN_POINT ( 'NONE',  ( 0.7479701569602201783, 0.9668092547198030573, 9.969517326151114744 ) ) ;
#31257=VERTEX_POINT ( 'NONE', #34698 ) ;
#31267=LINE ( 'NONE', #26891, #38180 ) ;
#31275=CARTESIAN_POINT ( 'NONE',  ( -31.84561714023301349, 33.32763979208128546, 8.807470649214879543 ) ) ;
#31279=VERTEX_POINT ( 'NONE', #13025 ) ;
#31280=B_SPLINE_CURVE_WITH_KNOTS ( 'NONE', 3,
 ( #46060, #2495, #29692, #45313 ),
 .UNSPECIFIED., .F., .F.,
 ( 4, 4 ),
 ( 0.9895749839358300992, 1.000000000000000000 ),
 .UNSPECIFIED. ) ;
#31294=ORIENTED_EDGE ( 'NONE', *, *, #6429, .T. ) ;
#31300=CARTESIAN_POINT ( 'NONE',  ( 9.970345420962653193, -0.8985218257325291447, 2.778652340038831436 ) ) ;
#31302=CARTESIAN_POINT ( 'NONE',  ( 0.000000000000000000, 0.000000000000000000, -10.00000000000000000 ) ) ;
#31307=CARTESIAN_POINT ( 'NONE',  ( 44.99506233596247995, 23.32283626942318833, 7.455576670931136185 ) ) ;
#31313=VERTEX_POINT ( 'NONE', #40243 ) ;
#31323=CARTESIAN_POINT ( 'NONE',  ( 0.8813691545818379547, 1.919529038513666297, 9.884520277910691988 ) ) ;
#31331=CARTESIAN_POINT ( 'NONE',  ( 6.174150299305392053, -50.00000000000000711, 8.807470649214879543 ) ) ;
#31334=ORIENTED_EDGE ( 'NONE', *, *, #4189, .F. ) ;
#31344=ADVANCED_FACE ( 'NONE', ( #40749 ), #15841, .T. ) ;
#31347=CARTESIAN_POINT ( 'NONE',  ( 46.76852358249013975, -17.86468378716709537, -9.367992836599954742 ) ) ;
#31348=CARTESIAN_POINT ( 'NONE',  ( 14.76429217231961566, 8.192625680377691566, 9.178419661560148768 ) ) ;
#31349=CARTESIAN_POINT ( 'NONE',  ( -13.59579750444763668, 10.60877755095910935, 8.727788335465566760 ) ) ;
#31351=VERTEX_POINT ( 'NONE', #24354 ) ;
#31374=CARTESIAN_POINT ( 'NONE',  ( -1.228394325311288560, 1.341866297401936636, 9.903764339332077782 ) ) ;
#31384=CARTESIAN_POINT ( 'NONE',  ( 2.943113318327519767, 2.672530871845234302, 3.247139928068174530 ) ) ;
#31392=CARTESIAN_POINT ( 'NONE',  ( 36.32827987961125871, -9.445964435368829015, 3.209567239418972928 ) ) ;
#31403=ORIENTED_EDGE ( 'NONE', *, *, #11626, .F. ) ;
#31416=CARTESIAN_POINT ( 'NONE',  ( 22.69295089195473736, 45.31600496604706052, 7.455576670931136185 ) ) ;
#31417=LINE ( 'NONE', #23958, #25050 ) ;
#31420=CARTESIAN_POINT ( 'NONE',  ( -27.25836557470613286, 25.76317754842369112, 8.100132398494515940 ) ) ;
#31425=B_SPLINE_SURFACE_WITH_KNOTS ( 'NONE', 3, 3, ( 
 ( #34642, #3062, #11284, #45639 ),
 ( #14877, #30526, #15125, #18460 ),
 ( #34148, #42566, #49721, #7180 ),
 ( #30275, #45884, #10762, #38742 ) ),
 .UNSPECIFIED., .F., .F., .F.,
 ( 4, 4 ),
 ( 4, 4 ),
 ( 0.000000000000000000, 1.000000000000000000 ),
 ( 0.000000000000000000, 1.000000000000000000 ),
 .UNSPECIFIED. ) ;
#31427=CARTESIAN_POINT ( 'NONE',  ( -0.2778388845795317086, 1.251314014313103851, 9.976582533991678048 ) ) ;
#31430=CARTESIAN_POINT ( 'NONE',  ( -0.3862712429686895876, 1.188820645368940720, 10.00000000000000000 ) ) ;
#31434=VERTEX_POINT ( 'NONE', #5844 ) ;
#31438=CARTESIAN_POINT ( 'NONE',  ( 3.975459390375365665, 0.2195152216756870167, 1.992221491942114397E-15 ) ) ;
#31446=EDGE_LOOP ( 'NONE', ( #38203, #12932, #42216, #33633, #30963 ) ) ;
#31454=CARTESIAN_POINT ( 'NONE',  ( -17.23491422248386584, 0.5912720620001978844, 8.727788335465566760 ) ) ;
#31457=CARTESIAN_POINT ( 'NONE',  ( -1.250000000000000222, 0.000000000000000000, 10.00000000000000000 ) ) ;
#31467=B_SPLINE_CURVE_WITH_KNOTS ( 'NONE', 3,
 ( #9454, #8959, #40516, #25118 ),
 .UNSPECIFIED., .F., .F.,
 ( 4, 4 ),
 ( 0.001937412222931636377, 0.003978261222106059536 ),
 .UNSPECIFIED. ) ;
#31481=CARTESIAN_POINT ( 'NONE',  ( -8.176860274785726190, 5.756644512789648616, 9.282506307616472441 ) ) ;
#31485=EDGE_CURVE ( 'NONE', #44630, #44983, #47757, .T. ) ;
#31492=CARTESIAN_POINT ( 'NONE',  ( 8.813458710706171928, 4.724716452304571490, 0.000000000000000000 ) ) ;
#31497=EDGE_LOOP ( 'NONE', ( #47182, #16613, #35641, #18132 ) ) ;
#31504=EDGE_CURVE ( 'NONE', #4426, #42650, #31280, .T. ) ;
#31510=B_SPLINE_CURVE_WITH_KNOTS ( 'NONE', 3,
 ( #27219, #46161, #31070, #6695 ),
 .UNSPECIFIED., .F., .F.,
 ( 4, 4 ),
 ( 0.000000000000000000, 0.2562577668812813236 ),
 .UNSPECIFIED. ) ;
#31525=B_SPLINE_CURVE_WITH_KNOTS ( 'NONE', 3,
 ( #1543, #40539, #783, #20526 ),
 .UNSPECIFIED., .F., .F.,
 ( 4, 4 ),
 ( 0.0006669682284780829038, 0.0007799402130931998951 ),
 .UNSPECIFIED. ) ;
#31529=VERTEX_POINT ( 'NONE', #11220 ) ;
#31530=ORIENTED_EDGE ( 'NONE', *, *, #7471, .T. ) ;
#31531=CARTESIAN_POINT ( 'NONE',  ( 30.22736451279166658, 39.84193304692632154, -2.408242355805840784 ) ) ;
#31535=CARTESIAN_POINT ( 'NONE',  ( -1.011271242968683426, -0.7347315653655928092, 3.333333333333333481 ) ) ;
#31540=CARTESIAN_POINT ( 'NONE',  ( -7.576114424932982594, 50.00000000000000711, 7.906207997025717304 ) ) ;
#31541=CARTESIAN_POINT ( 'NONE',  ( -1.080340181645087272, 0.5751155560365547315, 9.966990753365125855 ) ) ;
#31543=CARTESIAN_POINT ( 'NONE',  ( -0.1189258207540733747, -1.297644153576902326, 9.961922210043269388 ) ) ;
#31549=CARTESIAN_POINT ( 'NONE',  ( -2.943113374786527014, -2.672530809841224375, 3.247138655587367584 ) ) ;
#31557=DIRECTION ( 'NONE',  ( 0.000000000000000000, 0.000000000000000000, 1.000000000000000000 ) ) ;
#31563=ORIENTED_EDGE ( 'NONE', *, *, #6431, .T. ) ;
#31574=EDGE_CURVE ( 'NONE', #28100, #26320, #22711, .T. ) ;
#31584=DIRECTION ( 'NONE',  ( 0.000000000000000000, 0.000000000000000000, -1.000000000000000000 ) ) ;
#31602=CARTESIAN_POINT ( 'NONE',  ( 24.87968592351591823, 28.06706927586064637, -8.600750091277037157 ) ) ;
#31608=CARTESIAN_POINT ( 'NONE',  ( -1.512516825103204177, 0.5229758018505511474, 9.919954280166521698 ) ) ;
#31609=CARTESIAN_POINT ( 'NONE',  ( 28.96803024440893992, 18.11533787072037072, 7.455576670931136185 ) ) ;
#31612=EDGE_LOOP ( 'NONE', ( #48156, #23592, #4766, #2963 ) ) ;
#31617=CARTESIAN_POINT ( 'NONE',  ( -13.59579750444763668, 10.60877755095910935, 8.727788335465566760 ) ) ;
#31618=CARTESIAN_POINT ( 'NONE',  ( 1.104477492316107146, 0.6506302558160963478, 9.957892297621020461 ) ) ;
#31632=CARTESIAN_POINT ( 'NONE',  ( 12.78770032058947237, 31.68259716188277864, 7.455576670931136185 ) ) ;
#31640=EDGE_CURVE ( 'NONE', #41927, #6309, #36188, .T. ) ;
#31648=B_SPLINE_CURVE_WITH_KNOTS ( 'NONE', 3,
 ( #14615, #34149, #49969, #33883 ),
 .UNSPECIFIED., .F., .F.,
 ( 4, 4 ),
 ( 0.000000000000000000, 0.001246897409371940492 ),
 .UNSPECIFIED. ) ;
#31663=CARTESIAN_POINT ( 'NONE',  ( -7.726417830024645994, 6.396462539501611033, 9.390253821402618328 ) ) ;
#31675=ORIENTED_EDGE ( 'NONE', *, *, #27450, .T. ) ;
#31681=CARTESIAN_POINT ( 'NONE',  ( -8.176860274785726190, 5.756644512789648616, 9.282506307616472441 ) ) ;
#31682=CARTESIAN_POINT ( 'NONE',  ( 0.7246461030033715112, -1.181777192779797314, 9.960033073700731876 ) ) ;
#31692=CARTESIAN_POINT ( 'NONE',  ( -45.42829307628559832, -21.98948915213271960, 8.356839323120299312 ) ) ;
#31693=B_SPLINE_CURVE_WITH_KNOTS ( 'NONE', 3,
 ( #1705, #44775, #20692, #1461 ),
 .UNSPECIFIED., .F., .F.,
 ( 4, 4 ),
 ( 0.000000000000000000, 0.2562577668812812681 ),
 .UNSPECIFIED. ) ;
#31699=CARTESIAN_POINT ( 'NONE',  ( 8.277096487746778308, -50.00000000000000711, 7.455576670931136185 ) ) ;
#31705=B_SPLINE_CURVE_WITH_KNOTS ( 'NONE', 3,
 ( #12700, #2592, #36073, #45678 ),
 .UNSPECIFIED., .F., .F.,
 ( 4, 4 ),
 ( 0.003717756258871352318, 0.009855839347410961029 ),
 .UNSPECIFIED. ) ;
#31707=CARTESIAN_POINT ( 'NONE',  ( 1.096405084303662569, 0.6872075889365651946, 9.947020504990323531 ) ) ;
#31710=ORIENTED_EDGE ( 'NONE', *, *, #20871, .F. ) ;
#31723=B_SPLINE_CURVE_WITH_KNOTS ( 'NONE', 3,
 ( #5166, #9027, #20816, #43910 ),
 .UNSPECIFIED., .F., .F.,
 ( 4, 4 ),
 ( 2.577543251182695844E-16, 0.009782300387714808892 ),
 .UNSPECIFIED. ) ;
#31729=CARTESIAN_POINT ( 'NONE',  ( 0.6595498452743703277, -16.59563386392009576, 3.266473740018926541 ) ) ;
#31733=DIRECTION ( 'NONE',  ( 0.2599384441937613310, 0.8000082703740953871, 0.5407575913134970991 ) ) ;
#31738=CARTESIAN_POINT ( 'NONE',  ( -2.418900724918336298, -41.61933801977895087, -9.387872844313825738 ) ) ;
#31750=CARTESIAN_POINT ( 'NONE',  ( -1.104213410210672430, -0.6509177773818179968, 9.976582533991678048 ) ) ;
#31787=CARTESIAN_POINT ( 'NONE',  ( -13.59579750444763668, 10.60877755095910935, 8.727788335465566760 ) ) ;
#31789=EDGE_CURVE ( 'NONE', #16425, #10758, #16634, .T. ) ;
#31797=CARTESIAN_POINT ( 'NONE',  ( 35.34822294759176486, 12.62826869953554976, -3.721387749823083180 ) ) ;
#31798=ADVANCED_FACE ( 'NONE', ( #24792 ), #15420, .T. ) ;
#31809=EDGE_CURVE ( 'NONE', #31434, #27847, #38108, .T. ) ;
#31818=CARTESIAN_POINT ( 'NONE',  ( 0.7139173712341854161, -1.401061409226349141, 9.927288994922818688 ) ) ;
#31823=B_SPLINE_CURVE_WITH_KNOTS ( 'NONE', 3,
 ( #24731, #20111, #884, #39890 ),
 .UNSPECIFIED., .F., .F.,
 ( 4, 4 ),
 ( 5.445986106959422297E-16, 0.009782300387714812362 ),
 .UNSPECIFIED. ) ;
#31825=EDGE_CURVE ( 'NONE', #22094, #16336, #17583, .T. ) ;
#31836=CARTESIAN_POINT ( 'NONE',  ( -8.019230367734902387, 14.74354227315965282, -9.233365092205394475 ) ) ;
#31845=B_SPLINE_SURFACE_WITH_KNOTS ( 'NONE', 3, 3, ( 
 ( #7301, #26810, #50612, #31430 ),
 ( #31692, #22947, #27582, #50095 ),
 ( #27055, #8081, #39389, #35537 ),
 ( #46262, #4225, #30930, #7060 ) ),
 .UNSPECIFIED., .F., .F., .F.,
 ( 4, 4 ),
 ( 4, 4 ),
 ( 0.000000000000000000, 1.000000000000000000 ),
 ( 0.000000000000000000, 1.000000000000000000 ),
 .UNSPECIFIED. ) ;
#31850=CARTESIAN_POINT ( 'NONE',  ( 0.4400426740873927822, -2.015233077865103972, 9.886433018048071730 ) ) ;
#31854=CARTESIAN_POINT ( 'NONE',  ( 29.61572577327002520, 16.11461842845735859, 8.807470649214879543 ) ) ;
#31855=CARTESIAN_POINT ( 'NONE',  ( 14.29087950072012170, 9.652079258044652832, 8.727788335465566760 ) ) ;
#31864=CARTESIAN_POINT ( 'NONE',  ( -1.011271242968683426, -0.7347315653655928092, -10.00000000000000000 ) ) ;
#31871=CARTESIAN_POINT ( 'NONE',  ( 34.91952936320839740, -13.67027684621004546, -9.422646554964178023 ) ) ;
#31876=ORIENTED_EDGE ( 'NONE', *, *, #38117, .F. ) ;
#31880=CARTESIAN_POINT ( 'NONE',  ( 28.52604530808654815, 41.07801380285680892, -3.760136334089591248 ) ) ;
#31884=CARTESIAN_POINT ( 'NONE',  ( 0.6883547519190692521, -1.010122381805036440, 9.969517326150320713 ) ) ;
#31900=CARTESIAN_POINT ( 'NONE',  ( -1.468446590252919348, -0.3226319952343834063, 9.953784399990620813 ) ) ;
#31916=CARTESIAN_POINT ( 'NONE',  ( -6.909265173666245374, 36.86491375218297861, 8.100132398494514163 ) ) ;
#31918=ORIENTED_EDGE ( 'NONE', *, *, #11749, .F. ) ;
#31922=VERTEX_POINT ( 'NONE', #11400 ) ;
#31923=CARTESIAN_POINT ( 'NONE',  ( 0.000000000000000000, 0.000000000000000000, 0.000000000000000000 ) ) ;
#31938=EDGE_CURVE ( 'NONE', #22255, #22371, #41080, .T. ) ;
#31950=CARTESIAN_POINT ( 'NONE',  ( 9.999999999999994671, -1.084202172485504187E-16, 9.303249460322209785 ) ) ;
#31954=CARTESIAN_POINT ( 'NONE',  ( 23.26005729352310425, 44.90397804740356236, 7.906207997025717304 ) ) ;
#31961=ORIENTED_EDGE ( 'NONE', *, *, #12367, .T. ) ;
#31970=ORIENTED_EDGE ( 'NONE', *, *, #49125, .T. ) ;
#31972=ORIENTED_EDGE ( 'NONE', *, *, #26656, .F. ) ;
#31974=CIRCLE ( 'NONE', #23762, 10.00000000000000000 ) ;
#31987=CARTESIAN_POINT ( 'NONE',  ( 36.08557433729230723, -35.58569447144768105, 7.455576670931136185 ) ) ;
#31991=CARTESIAN_POINT ( 'NONE',  ( -10.28825587112213746, 13.03847615613166333, 3.266473740018926541 ) ) ;
#31997=CARTESIAN_POINT ( 'NONE',  ( -1.468713901642213493, -0.3220470327672489419, 9.927319414211227766 ) ) ;
#32006=LINE ( 'NONE', #29158, #34703 ) ;
#32012=ORIENTED_EDGE ( 'NONE', *, *, #17830, .F. ) ;
#32016=ORIENTED_EDGE ( 'NONE', *, *, #27218, .F. ) ;
#32022=EDGE_CURVE ( 'NONE', #29885, #8231, #44685, .T. ) ;
#32027=ORIENTED_EDGE ( 'NONE', *, *, #41067, .F. ) ;
#32049=CARTESIAN_POINT ( 'NONE',  ( 15.00099850811936264, 7.462898891544210933, 9.403735324607438884 ) ) ;
#32055=DIRECTION ( 'NONE',  ( -0.9510565162951566398, 0.3090169943749383474, 0.000000000000000000 ) ) ;
#32058=CARTESIAN_POINT ( 'NONE',  ( -33.86622497129646092, 3.037805405905158462, 7.906207997025717304 ) ) ;
#32062=CARTESIAN_POINT ( 'NONE',  ( -33.14391172085786508, -37.72293746533094350, -8.016098858316205167 ) ) ;
#32063=CARTESIAN_POINT ( 'NONE',  ( 0.6215990105956902267, -1.608617984725389860, 9.928159647716132241 ) ) ;
#32065=ORIENTED_EDGE ( 'NONE', *, *, #24379, .F. ) ;
#32075=CARTESIAN_POINT ( 'NONE',  ( -1.270883027774187379, -0.2878889193224725696, 9.961922210043276493 ) ) ;
#32103=EDGE_CURVE ( 'NONE', #49222, #36524, #31823, .T. ) ;
#32117=CYLINDRICAL_SURFACE ( 'NONE', #13328, 37.50000000000000000 ) ;
#32119=CARTESIAN_POINT ( 'NONE',  ( 27.73884755486784570, -25.23502201956245017, 7.697694107796188234 ) ) ;
#32130=CARTESIAN_POINT ( 'NONE',  ( 1.553222296440332606, -1.431397764604065204, 9.884520316594379352 ) ) ;
#32151=CARTESIAN_POINT ( 'NONE',  ( -4.672045878990125800, 50.00000000000000711, 1.847720168420772691 ) ) ;
#32175=CARTESIAN_POINT ( 'NONE',  ( 8.277096487746778308, -50.00000000000000711, 7.455576670931136185 ) ) ;
#32178=VECTOR ( 'NONE', #7935, 999.9999999999998863 ) ;
#32180=FACE_OUTER_BOUND ( 'NONE', #8505, .T. ) ;
#32191=CARTESIAN_POINT ( 'NONE',  ( 3.940019464150765760, 50.00000000000000711, -8.466730184410787174 ) ) ;
#32198=FACE_OUTER_BOUND ( 'NONE', #37396, .T. ) ;
#32199=CARTESIAN_POINT ( 'NONE',  ( 15.45175104485250728, -6.222373774239001065, -2.870787844569587133 ) ) ;
#32219=VERTEX_POINT ( 'NONE', #26237 ) ;
#32220=ORIENTED_EDGE ( 'NONE', *, *, #6429, .F. ) ;
#32222=CARTESIAN_POINT ( 'NONE',  ( 2.569099690548740877, -50.00000000000000711, 3.199614146704519602 ) ) ;
#32227=CARTESIAN_POINT ( 'NONE',  ( 1.377551617740986334, -0.6025367262284159198, 9.936141075690080982 ) ) ;
#32232=CARTESIAN_POINT ( 'NONE',  ( -2.210477865340801706, -37.43479381012853224, -9.422646554964178023 ) ) ;
#32236=CARTESIAN_POINT ( 'NONE',  ( -15.62858259096117841, 5.755205073598721910, -9.683996418299976483 ) ) ;
#32237=CARTESIAN_POINT ( 'NONE',  ( 46.76852358249013975, -17.86468378716709537, -9.367992836599954742 ) ) ;
#32238=B_SPLINE_CURVE_WITH_KNOTS ( 'NONE', 3,
 ( #27096, #4503, #34815, #27862 ),
 .UNSPECIFIED., .F., .F.,
 ( 4, 4 ),
 ( 0.000000000000000000, 0.0002610106747149790337 ),
 .UNSPECIFIED. ) ;
#32244=CARTESIAN_POINT ( 'NONE',  ( -1.531049279420139131, -0.4659387722959919542, 9.919954280166518146 ) ) ;
#32247=ORIENTED_EDGE ( 'NONE', *, *, #11521, .T. ) ;
#32248=CARTESIAN_POINT ( 'NONE',  ( 22.90865447854256232, 29.73489050103220777, -2.490396854064190979 ) ) ;
#32257=B_SPLINE_SURFACE_WITH_KNOTS ( 'NONE', 3, 3, ( 
 ( #24627, #5105, #32587, #40526 ),
 ( #5364, #1530, #23221, #15293 ),
 ( #35313, #38390, #14770, #22469 ),
 ( #23496, #46785, #149, #11430 ) ),
 .UNSPECIFIED., .F., .F., .F.,
 ( 4, 4 ),
 ( 4, 4 ),
 ( 0.000000000000000000, 1.000000000000000000 ),
 ( 0.000000000000000000, 1.000000000000000000 ),
 .UNSPECIFIED. ) ;
#32260=CARTESIAN_POINT ( 'NONE',  ( -0.3978397141392489011, 0.1292659590674825332, 9.992713367193012175 ) ) ;
#32269=ORIENTED_EDGE ( 'NONE', *, *, #745, .F. ) ;
#32271=B_SPLINE_CURVE_WITH_KNOTS ( 'NONE', 3,
 ( #35735, #15955, #38808, #35973, #4153, #4662 ),
 .UNSPECIFIED., .F., .F.,
 ( 4, 2, 4 ),
 ( 4.635316164197443437E-17, 0.009882509389272372408, 0.01976501877854469624 ),
 .UNSPECIFIED. ) ;
#32277=EDGE_CURVE ( 'NONE', #26320, #19053, #50099, .T. ) ;
#32287=ADVANCED_FACE ( 'NONE', ( #38560 ), #36371, .T. ) ;
#32297=DIRECTION ( 'NONE',  ( 0.000000000000000000, 0.000000000000000000, 1.000000000000000000 ) ) ;
#32298=CARTESIAN_POINT ( 'NONE',  ( 36.46533180484010472, 8.777022568848463990, -9.011255500499647297 ) ) ;
#32332=CARTESIAN_POINT ( 'NONE',  ( -0.9600884595229873808, 0.8493647100668667571, 9.957892297621016908 ) ) ;
#32338=ORIENTED_EDGE ( 'NONE', *, *, #46294, .F. ) ;
#32348=CARTESIAN_POINT ( 'NONE',  ( -36.08557433729205144, 35.58569447144795816, 7.455576670931136185 ) ) ;
#32352=DIRECTION ( 'NONE',  ( 1.000000000000000000, 0.000000000000000000, 0.000000000000000000 ) ) ;
#32353=CARTESIAN_POINT ( 'NONE',  ( -0.3862712429686977478, 1.188820645368937390, 10.00000000000000000 ) ) ;
#32354=VERTEX_POINT ( 'NONE', #50283 ) ;
#32362=ORIENTED_EDGE ( 'NONE', *, *, #9656, .F. ) ;
#32363=CARTESIAN_POINT ( 'NONE',  ( 24.39427009665984869, 44.07992421011656603, 8.807470649214879543 ) ) ;
#32371=ORIENTED_EDGE ( 'NONE', *, *, #8597, .T. ) ;
#32378=ORIENTED_EDGE ( 'NONE', *, *, #27123, .T. ) ;
#32380=ORIENTED_EDGE ( 'NONE', *, *, #1054, .T. ) ;
#32385=ORIENTED_EDGE ( 'NONE', *, *, #17975, .T. ) ;
#32387=ORIENTED_EDGE ( 'NONE', *, *, #6489, .T. ) ;
#32400=CARTESIAN_POINT ( 'NONE',  ( -0.9358216137853901939, 0.9039474357307636376, 9.986087673579197244 ) ) ;
#32403=CARTESIAN_POINT ( 'NONE',  ( 2.538055338523177440, 50.00000000000000711, -9.367992836599954742 ) ) ;
#32411=EDGE_CURVE ( 'NONE', #50487, #12217, #25088, .T. ) ;
#32420=CARTESIAN_POINT ( 'NONE',  ( -6.174150299305392053, 33.14591993373988998, 8.807470649214879543 ) ) ;
#32438=CARTESIAN_POINT ( 'NONE',  ( -0.3862712429686729343, -1.188820645368946050, 10.00000000000000000 ) ) ;
#32445=B_SPLINE_CURVE_WITH_KNOTS ( 'NONE', 3,
 ( #23606, #533, #47171, #24133 ),
 .UNSPECIFIED., .F., .F.,
 ( 4, 4 ),
 ( 0.000000000000000000, 0.0002520763768929601498 ),
 .UNSPECIFIED. ) ;
#32448=CARTESIAN_POINT ( 'NONE',  ( 1.066995270233474624, -50.00000000000000711, -3.760136334089591248 ) ) ;
#32452=CARTESIAN_POINT ( 'NONE',  ( 9.999630309108590964, 0.09931773306215448127, 9.289350385289854017 ) ) ;
#32455=ORIENTED_EDGE ( 'NONE', *, *, #16684, .T. ) ;
#32458=CARTESIAN_POINT ( 'NONE',  ( -0.3862712429686729343, -1.188820645368946050, 3.333333333333333481 ) ) ;
#32520=VERTEX_POINT ( 'NONE', #17947 ) ;
#32524=CARTESIAN_POINT ( 'NONE',  ( 1.035950918207909632, 50.00000000000000711, -2.408242355805840784 ) ) ;
#32534=CARTESIAN_POINT ( 'NONE',  ( -4.672045878990125800, 33.19353511768168374, 1.847720168420772691 ) ) ;
#32535=CARTESIAN_POINT ( 'NONE',  ( -24.39427009666018265, -44.07992421011638129, 8.807470649214879543 ) ) ;
#32538=LINE ( 'NONE', #24570, #30874 ) ;
#32539=CARTESIAN_POINT ( 'NONE',  ( -1.011271242968693862, 0.7347315653655780432, 10.00000000000000000 ) ) ;
#32546=ORIENTED_EDGE ( 'NONE', *, *, #3976, .F. ) ;
#32548=CARTESIAN_POINT ( 'NONE',  ( -1.011271242968683426, -0.7347315653655928092, -3.333333333333333481 ) ) ;
#32560=CARTESIAN_POINT ( 'NONE',  ( -21.58778298521296080, 25.34222074689773407, 3.199614146704519602 ) ) ;
#32561=ORIENTED_EDGE ( 'NONE', *, *, #3543, .T. ) ;
#32567=B_SPLINE_CURVE_WITH_KNOTS ( 'NONE', 3,
 ( #49799, #50054, #3140, #34998 ),
 .UNSPECIFIED., .F., .F.,
 ( 4, 4 ),
 ( 1.734723475976807094E-18, 0.002458791966311097647 ),
 .UNSPECIFIED. ) ;
#32574=VERTEX_POINT ( 'NONE', #28762 ) ;
#32575=CARTESIAN_POINT ( 'NONE',  ( 3.808200756227633654, 0.8261963378076531139, 9.741991644047248045 ) ) ;
#32578=ADVANCED_FACE ( 'NONE', ( #33381 ), #19085, .T. ) ;
#32584=CARTESIAN_POINT ( 'NONE',  ( -24.39427009666018265, -44.07992421011638129, 8.807470649214879543 ) ) ;
#32587=CARTESIAN_POINT ( 'NONE',  ( -2.462075149652696027, 16.57295996686994499, 9.403735324607438884 ) ) ;
#32589=CARTESIAN_POINT ( 'NONE',  ( -9.260964247899876156, 13.84230907185616744, -9.683996418299976483 ) ) ;
#32604=CARTESIAN_POINT ( 'NONE',  ( 28.52604530808654815, 41.07801380285680892, -3.760136334089591248 ) ) ;
#32606=CARTESIAN_POINT ( 'NONE',  ( 9.174209336589868258, 3.979181203266223488, 9.646707543097347681 ) ) ;
#32612=EDGE_CURVE ( 'NONE', #41298, #12448, #41617, .T. ) ;
#32615=ORIENTED_EDGE ( 'NONE', *, *, #18001, .F. ) ;
#32628=EDGE_CURVE ( 'NONE', #20753, #15030, #42253, .T. ) ;
#32633=ORIENTED_EDGE ( 'NONE', *, *, #27123, .F. ) ;
#32635=ORIENTED_EDGE ( 'NONE', *, *, #20651, .F. ) ;
#32638=CARTESIAN_POINT ( 'NONE',  ( 1.540526284687965264, -1.371707213411490267, 9.886433018048071730 ) ) ;
#32640=CARTESIAN_POINT ( 'NONE',  ( 15.44803555374680393, 6.237487519713364570, -3.546734833711462365 ) ) ;
#32641=ORIENTED_EDGE ( 'NONE', *, *, #42891, .T. ) ;
#32647=CARTESIAN_POINT ( 'NONE',  ( -0.03684434657425742637, -1.221810944802247167, 9.969517326150317160 ) ) ;
#32662=CARTESIAN_POINT ( 'NONE',  ( -7.608425291889091113, 36.72004717559254772, 7.697694107796188234 ) ) ;
#32688=CARTESIAN_POINT ( 'NONE',  ( 30.65355587399079340, -13.36566953343588260, -8.917361510505369182 ) ) ;
#32689=LINE ( 'NONE', #36813, #13868 ) ;
#32693=CARTESIAN_POINT ( 'NONE',  ( 5.083187235775197266, 8.611690166631179366, 9.646707543097347681 ) ) ;
#32697=ORIENTED_EDGE ( 'NONE', *, *, #19919, .F. ) ;
#32699=ADVANCED_FACE ( 'NONE', ( #31043 ), #31425, .T. ) ;
#32701=VECTOR ( 'NONE', #30873, 1000.000000000000114 ) ;
#32703=ORIENTED_EDGE ( 'NONE', *, *, #41485, .T. ) ;
#32708=EDGE_LOOP ( 'NONE', ( #1214, #47945, #26961, #1564 ) ) ;
#32711=B_SPLINE_CURVE_WITH_KNOTS ( 'NONE', 3,
 ( #28039, #1104, #31663, #12144 ),
 .UNSPECIFIED., .F., .F.,
 ( 4, 4 ),
 ( 0.000000000000000000, 0.002368422649471282979 ),
 .UNSPECIFIED. ) ;
#32714=ADVANCED_FACE ( 'NONE', ( #46639 ), #27727, .T. ) ;
#32716=CARTESIAN_POINT ( 'NONE',  ( -10.28825587112213746, 13.03847615613166333, 3.266473740018926541 ) ) ;
#32718=ORIENTED_EDGE ( 'NONE', *, *, #15093, .F. ) ;
#32720=EDGE_LOOP ( 'NONE', ( #19187, #29031, #44696 ) ) ;
#32743=B_SPLINE_CURVE_WITH_KNOTS ( 'NONE', 3,
 ( #39493, #4331, #43061, #39237 ),
 .UNSPECIFIED., .F., .F.,
 ( 4, 4 ),
 ( 0.7998230999345288250, 0.9869080488566185361 ),
 .UNSPECIFIED. ) ;
#32750=CARTESIAN_POINT ( 'NONE',  ( 0.3370904143228959926, -0.2449105217885284291, 10.00000000000000000 ) ) ;
#32759=CARTESIAN_POINT ( 'NONE',  ( 1.142975459103954705, 16.61830776097024653, -2.870787844569587133 ) ) ;
#32765=CARTESIAN_POINT ( 'NONE',  ( -1.275994128725546739, 0.1230186051320636409, 9.948547179989615685 ) ) ;
#32772=EDGE_CURVE ( 'NONE', #12798, #40675, #36099, .T. ) ;
#32793=DIRECTION ( 'NONE',  ( 0.2599384441937669932, -0.8000082703740931667, -0.5407575913134976542 ) ) ;
#32798=CARTESIAN_POINT ( 'NONE',  ( 18.69789054174343690, -27.49790346457731616, -2.408242355805840784 ) ) ;
#32803=ADVANCED_FACE ( 'NONE', ( #44077 ), #8945, .F. ) ;
#32810=DIRECTION ( 'NONE',  ( -1.000000000000000000, 0.000000000000000000, 0.000000000000000000 ) ) ;
#32811=ORIENTED_EDGE ( 'NONE', *, *, #24236, .F. ) ;
#32813=CARTESIAN_POINT ( 'NONE',  ( -1.019713130072858798, -3.848720492505054658, 6.098637220230962441E-17 ) ) ;
#32815=B_SPLINE_CURVE_WITH_KNOTS ( 'NONE', 3,
 ( #10422, #21208, #21970, #14519 ),
 .UNSPECIFIED., .F., .F.,
 ( 4, 4 ),
 ( 0.0001970727314178603461, 0.006335152926028601167 ),
 .UNSPECIFIED. ) ;
#32822=B_SPLINE_CURVE_WITH_KNOTS ( 'NONE', 3,
 ( #24186, #47232, #28022, #15711 ),
 .UNSPECIFIED., .F., .F.,
 ( 4, 4 ),
 ( 0.000000000000000000, 8.326314924661335100E-06 ),
 .UNSPECIFIED. ) ;
#32825=CARTESIAN_POINT ( 'NONE',  ( 46.76852358249013975, -17.86468378716709537, -9.367992836599954742 ) ) ;
#32861=CARTESIAN_POINT ( 'NONE',  ( -26.18032376592659105, 21.95228666728381128, 7.455576670931136185 ) ) ;
#32864=CARTESIAN_POINT ( 'NONE',  ( -1.011271242968693862, 0.7347315653655780432, 3.333333333333333481 ) ) ;
#32877=CARTESIAN_POINT ( 'NONE',  ( -47.23269937569316568, 16.43609759007082616, -2.408242355805840784 ) ) ;
#32879=CARTESIAN_POINT ( 'NONE',  ( 19.52505477809945944, 36.96330698207086840, 8.846626183609803462 ) ) ;
#32880=CARTESIAN_POINT ( 'NONE',  ( -32.43949840348904701, -7.871562655726274116, -9.367992836599954742 ) ) ;
#32886=CARTESIAN_POINT ( 'NONE',  ( 34.38425513258721367, -36.82177522737821107, 8.807470649214879543 ) ) ;
#32895=B_SPLINE_CURVE_WITH_KNOTS ( 'NONE', 3,
 ( #1842, #40341, #28536, #47736 ),
 .UNSPECIFIED., .F., .F.,
 ( 4, 4 ),
 ( 0.001248798139576341119, 0.001653158300360187301 ),
 .UNSPECIFIED. ) ;
#32902=CARTESIAN_POINT ( 'NONE',  ( -0.3862712429686977478, 1.188820645368937390, -3.333333333333333481 ) ) ;
#32904=ORIENTED_EDGE ( 'NONE', *, *, #36038, .F. ) ;
#32912=DIRECTION ( 'NONE',  ( 0.000000000000000000, 0.000000000000000000, -1.000000000000000000 ) ) ;
#32914=EDGE_CURVE ( 'NONE', #45083, #42215, #8550, .T. ) ;
#32918=CARTESIAN_POINT ( 'NONE',  ( -1.424123654778022274, -0.3625862473323341328, 9.958264684458713489 ) ) ;
#32924=ORIENTED_EDGE ( 'NONE', *, *, #24897, .F. ) ;
#32942=CARTESIAN_POINT ( 'NONE',  ( 0.3656201545664388708, -2.182515578491310393, 9.881002359080277131 ) ) ;
#32949=CARTESIAN_POINT ( 'NONE',  ( 0.1287570809895575430, 0.3962735484563150168, 10.00000000000000000 ) ) ;
#32961=DIRECTION ( 'NONE',  ( 0.000000000000000000, 0.000000000000000000, -1.000000000000000000 ) ) ;
#32962=CARTESIAN_POINT ( 'NONE',  ( 1.011271242968694084, -0.7347315653655782652, 10.00000000000000000 ) ) ;
#32968=CARTESIAN_POINT ( 'NONE',  ( 47.22310614333766665, 16.46562252335956344, -3.760136334089591248 ) ) ;
#32970=ORIENTED_EDGE ( 'NONE', *, *, #23160, .F. ) ;
#32971=FACE_OUTER_BOUND ( 'NONE', #408, .T. ) ;
#32977=ORIENTED_EDGE ( 'NONE', *, *, #16468, .F. ) ;
#32980=ORIENTED_EDGE ( 'NONE', *, *, #7705, .T. ) ;
#32999=ORIENTED_EDGE ( 'NONE', *, *, #18294, .T. ) ;
#33000=CARTESIAN_POINT ( 'NONE',  ( -0.3862712429686809279, -1.188820645368943163, -10.00000000000000000 ) ) ;
#33002=B_SPLINE_SURFACE_WITH_KNOTS ( 'NONE', 3, 3, ( 
 ( #35938, #1285, #32589, #8479 ),
 ( #43860, #776, #5110, #47669 ),
 ( #16936, #17175, #31836, #24629 ),
 ( #12821, #8975, #12558, #48426 ) ),
 .UNSPECIFIED., .F., .F., .F.,
 ( 4, 4 ),
 ( 4, 4 ),
 ( 0.000000000000000000, 1.000000000000000000 ),
 ( 0.000000000000000000, 1.000000000000000000 ),
 .UNSPECIFIED. ) ;
#33006=CARTESIAN_POINT ( 'NONE',  ( 8.277096487746778308, -33.14818118907697198, 7.455576670931136185 ) ) ;
#33007=CARTESIAN_POINT ( 'NONE',  ( 0.000000000000000000, 0.000000000000000000, 10.00000000000000000 ) ) ;
#33020=CARTESIAN_POINT ( 'NONE',  ( -0.1287570809895602630, -0.3962735484563142396, 10.00000000000000000 ) ) ;
#33030=CARTESIAN_POINT ( 'NONE',  ( 16.52264463346132572, -2.779753662172757878, 9.403735324607438884 ) ) ;
#33039=ADVANCED_FACE ( 'NONE', ( #11164 ), #31845, .T. ) ;
#33040=CARTESIAN_POINT ( 'NONE',  ( -1.901953004002570502, -1.028591558669202488, 9.885585981620943485 ) ) ;
#33043=CARTESIAN_POINT ( 'NONE',  ( -10.70590866674912967, 12.76446523155714985, -3.546734833711462365 ) ) ;
#33057=CARTESIAN_POINT ( 'NONE',  ( 33.01266944765062306, -5.813986777101467496, 1.847720168420772691 ) ) ;
#33072=CARTESIAN_POINT ( 'NONE',  ( -3.630679331413954714, -37.33064849398144958, -8.600750091277037157 ) ) ;
#33075=CARTESIAN_POINT ( 'NONE',  ( 33.01266944765062306, -5.813986777101467496, 1.847720168420772691 ) ) ;
#33079=EDGE_CURVE ( 'NONE', #11140, #5897, #28078, .T. ) ;
#33085=ORIENTED_EDGE ( 'NONE', *, *, #14351, .T. ) ;
#33087=CARTESIAN_POINT ( 'NONE',  ( 1.011271242968688311, -0.7347315653655855927, 10.00000000000000000 ) ) ;
#33114=CARTESIAN_POINT ( 'NONE',  ( 1.011271242968683648, 0.7347315653655930312, 10.00000000000000000 ) ) ;
#33115=CARTESIAN_POINT ( 'NONE',  ( -0.6595498452743703277, 16.59563386392009576, 3.266473740018926541 ) ) ;
#33121=CARTESIAN_POINT ( 'NONE',  ( -30.12518629743573584, -14.70074613238887551, 1.847720168420772691 ) ) ;
#33131=CARTESIAN_POINT ( 'NONE',  ( 17.34922095635755568, 33.24536858281893359, 8.914903342594564961 ) ) ;
#33149=CARTESIAN_POINT ( 'NONE',  ( -24.39427009666018265, -44.07992421011638129, 8.807470649214879543 ) ) ;
#33157=CARTESIAN_POINT ( 'NONE',  ( -25.61277432017861955, 22.36370378792854297, 7.906207997025717304 ) ) ;
#33161=EDGE_LOOP ( 'NONE', ( #28288, #25626, #21913 ) ) ;
#33174=CARTESIAN_POINT ( 'NONE',  ( -47.23269937569316568, 16.43609759007082616, -2.408242355805840784 ) ) ;
#33183=CARTESIAN_POINT ( 'NONE',  ( -4.672045878990125800, 50.00000000000000711, 1.847720168420772691 ) ) ;
#33198=CARTESIAN_POINT ( 'NONE',  ( -0.1473596192760168455, -1.496323530725124584, 9.936141075690080982 ) ) ;
#33209=CARTESIAN_POINT ( 'NONE',  ( 8.019230367735008969, -14.74354227315958887, -9.233365092205394475 ) ) ;
#33212=EDGE_CURVE ( 'NONE', #6277, #38645, #25997, .T. ) ;
#33214=CARTESIAN_POINT ( 'NONE',  ( 13.35436367797824353, 31.26996044524050333, 7.906207997025717304 ) ) ;
#33217=CARTESIAN_POINT ( 'NONE',  ( 4.412346620047078893, 9.007664521157071391, 9.516222621873129839 ) ) ;
#33221=CARTESIAN_POINT ( 'NONE',  ( -3.940019464150765760, -50.00000000000000711, -8.466730184410787174 ) ) ;
#33231=ORIENTED_EDGE ( 'NONE', *, *, #16697, .F. ) ;
#33234=CARTESIAN_POINT ( 'NONE',  ( 1.019713130072856355, 3.848720492505100843, 4.370690007832189750E-16 ) ) ;
#33243=ORIENTED_EDGE ( 'NONE', *, *, #47892, .F. ) ;
#33256=CARTESIAN_POINT ( 'NONE',  ( 0.3862712429686727678, 1.188820645368945605, -3.333333333333333481 ) ) ;
#33257=CARTESIAN_POINT ( 'NONE',  ( -1.249999999999999778, 0.000000000000000000, 10.00000000000000000 ) ) ;
#33263=CARTESIAN_POINT ( 'NONE',  ( 0.4166666666666664631, 0.000000000000000000, 10.00000000000000000 ) ) ;
#33266=CARTESIAN_POINT ( 'NONE',  ( 29.61572577327002520, 16.11461842845735859, 8.807470649214879543 ) ) ;
#33278=ORIENTED_EDGE ( 'NONE', *, *, #8260, .F. ) ;
#33289=CARTESIAN_POINT ( 'NONE',  ( 0.1287570809895575430, 0.3962735484563150168, 10.00000000000000000 ) ) ;
#33311=CARTESIAN_POINT ( 'NONE',  ( 23.31729631074197329, 24.19776167542427814, -8.016098858316199838 ) ) ;
#33313=CARTESIAN_POINT ( 'NONE',  ( -9.260964247899874380, 13.84230907185616744, -9.683996418299976483 ) ) ;
#33314=CARTESIAN_POINT ( 'NONE',  ( -10.28825587112213746, 13.03847615613166333, 3.266473740018926541 ) ) ;
#33315=ORIENTED_EDGE ( 'NONE', *, *, #31574, .T. ) ;
#33317=CARTESIAN_POINT ( 'NONE',  ( -28.96803024440907137, -18.11533787072017176, 7.455576670931136185 ) ) ;
#33324=CARTESIAN_POINT ( 'NONE',  ( 1.193089574352119264, 0.2545860991493882342, 9.963925895596188909 ) ) ;
#33330=FACE_OUTER_BOUND ( 'NONE', #50135, .T. ) ;
#33337=EDGE_LOOP ( 'NONE', ( #39550, #46634, #12236, #7330 ) ) ;
#33345=CARTESIAN_POINT ( 'NONE',  ( -0.6126904405382037622, -1.085824959725731231, 9.981352469109934233 ) ) ;
#33346=ADVANCED_FACE ( 'NONE', ( #2141 ), #24479, .T. ) ;
#33353=DIRECTION ( 'NONE',  ( 0.000000000000000000, 0.000000000000000000, -1.000000000000000000 ) ) ;
#33355=ADVANCED_FACE ( 'NONE', ( #11608 ), #31000, .T. ) ;
#33357=EDGE_CURVE ( 'NONE', #13072, #14294, #39096, .T. ) ;
#33365=B_SPLINE_CURVE_WITH_KNOTS ( 'NONE', 3,
 ( #46026, #39151, #11428, #42460 ),
 .UNSPECIFIED., .F., .F.,
 ( 4, 4 ),
 ( 0.9890644561681869451, 1.000000000000000000 ),
 .UNSPECIFIED. ) ;
#33368=CARTESIAN_POINT ( 'NONE',  ( -0.6883547519190790220, 1.010122381805031333, 9.969517326150315384 ) ) ;
#33370=CARTESIAN_POINT ( 'NONE',  ( -16.02661358026017879, -4.530191650547607196, -9.683996418299976483 ) ) ;
#33374=CARTESIAN_POINT ( 'NONE',  ( 7.398363427652525637, -15.19415887381133246, -9.008049429158100807 ) ) ;
#33375=CARTESIAN_POINT ( 'NONE',  ( -0.1287570809895632329, 0.3962735484563137400, 10.00000000000000000 ) ) ;
#33381=FACE_OUTER_BOUND ( 'NONE', #31446, .T. ) ;
#33382=CARTESIAN_POINT ( 'NONE',  ( -8.277096487746778308, 50.00000000000000711, 7.455576670931136185 ) ) ;
#33390=CARTESIAN_POINT ( 'NONE',  ( -0.4166666666666664631, 0.000000000000000000, 10.00000000000000000 ) ) ;
#33392=B_SPLINE_CURVE_WITH_KNOTS ( 'NONE', 3,
 ( #30907, #27031, #11382, #7546, #19584, #19334 ),
 .UNSPECIFIED., .F., .F.,
 ( 4, 2, 4 ),
 ( 4.246530788431251365E-17, 0.009882509389272368938, 0.01976501877854469624 ),
 .UNSPECIFIED. ) ;
#33402=ORIENTED_EDGE ( 'NONE', *, *, #11424, .T. ) ;
#33416=CARTESIAN_POINT ( 'NONE',  ( 0.3501237319956588823, -1.209643720083640739, 9.974012008644017158 ) ) ;
#33418=B_SPLINE_SURFACE_WITH_KNOTS ( 'NONE', 3, 3, ( 
 ( #40186, #20679, #18801, #42662 ),
 ( #30376, #34486, #3929, #3152 ),
 ( #30894, #35250, #19569, #46990 ),
 ( #4188, #93, #15475, #46480 ) ),
 .UNSPECIFIED., .F., .F., .F.,
 ( 4, 4 ),
 ( 4, 4 ),
 ( 0.000000000000000000, 1.000000000000000000 ),
 ( 0.000000000000000000, 1.000000000000000000 ),
 .UNSPECIFIED. ) ;
#33424=CARTESIAN_POINT ( 'NONE',  ( -1.317555876316872210, -0.4584864758884910074, 9.955131761384825140 ) ) ;
#33425=EDGE_CURVE ( 'NONE', #39856, #20753, #31179, .T. ) ;
#33427=ORIENTED_EDGE ( 'NONE', *, *, #2418, .T. ) ;
#33429=ADVANCED_FACE ( 'NONE', ( #25799 ), #21430, .F. ) ;
#33436=ORIENTED_EDGE ( 'NONE', *, *, #18808, .T. ) ;
#33445=CARTESIAN_POINT ( 'NONE',  ( 1.080000014128428498, 0.7606467978644730898, 9.943883492372853183 ) ) ;
#33447=CARTESIAN_POINT ( 'NONE',  ( -0.1471466405331013361, -1.496299042407428503, 9.944962737616616977 ) ) ;
#33451=CARTESIAN_POINT ( 'NONE',  ( -9.221081804193374865, -13.81382350053984176, 3.266473740018926541 ) ) ;
#33458=CARTESIAN_POINT ( 'NONE',  ( 30.22736451279166658, 39.84193304692632154, -2.408242355805840784 ) ) ;
#33462=VERTEX_POINT ( 'NONE', #48847 ) ;
#33473=EDGE_CURVE ( 'NONE', #35501, #12321, #9620, .T. ) ;
#33482=CARTESIAN_POINT ( 'NONE',  ( -1.104213410210672430, -0.6509177773818179968, 9.976582533991678048 ) ) ;
#33497=B_SPLINE_CURVE_WITH_KNOTS ( 'NONE', 3,
 ( #48229, #9771, #2091, #25434 ),
 .UNSPECIFIED., .F., .F.,
 ( 4, 4 ),
 ( 0.0003760194760237283622, 0.0006307719036365527603 ),
 .UNSPECIFIED. ) ;
#33504=LINE ( 'NONE', #25795, #30599 ) ;
#33509=CARTESIAN_POINT ( 'NONE',  ( 31.44259251615245887, 38.95901822126169378, -9.367992836599951190 ) ) ;
#33512=FACE_OUTER_BOUND ( 'NONE', #19885, .T. ) ;
#33515=B_SPLINE_SURFACE_WITH_KNOTS ( 'NONE', 3, 3, ( 
 ( #48706, #44135, #13346, #24912 ),
 ( #32877, #13097, #40558, #2304 ),
 ( #21552, #37242, #48459, #44381 ),
 ( #17212, #21303, #17939, #29258 ) ),
 .UNSPECIFIED., .F., .F., .F.,
 ( 4, 4 ),
 ( 4, 4 ),
 ( 0.000000000000000000, 1.000000000000000000 ),
 ( 0.000000000000000000, 1.000000000000000000 ),
 .UNSPECIFIED. ) ;
#33520=CARTESIAN_POINT ( 'NONE',  ( 1.011271242968683648, 0.7347315653655930312, 10.00000000000000000 ) ) ;
#33526=CARTESIAN_POINT ( 'NONE',  ( -0.3910393408547386818, -3.877122853643371947, 9.741991644047244492 ) ) ;
#33527=CARTESIAN_POINT ( 'NONE',  ( 37.09503908879513290, -5.733418411338704779, 4.835783797351805191 ) ) ;
#33545=B_SPLINE_CURVE_WITH_KNOTS ( 'NONE', 3,
 ( #35152, #4082, #3307, #19978 ),
 .UNSPECIFIED., .F., .F.,
 ( 4, 4 ),
 ( 0.0001535465953327018473, 0.0005837444810856221586 ),
 .UNSPECIFIED. ) ;
#33557=CARTESIAN_POINT ( 'NONE',  ( 27.31081730472575941, 41.96092862852144378, 3.199614146704519602 ) ) ;
#33558=CARTESIAN_POINT ( 'NONE',  ( 0.8808108730164768696, 0.8497440890325094198, 9.966990753364711964 ) ) ;
#33559=CARTESIAN_POINT ( 'NONE',  ( -36.76598589393961447, -7.383243274241610088, -8.192531242611266862 ) ) ;
#33560=CARTESIAN_POINT ( 'NONE',  ( -1.011271242968683426, -0.7347315653655928092, -10.00000000000000000 ) ) ;
#33561=CARTESIAN_POINT ( 'NONE',  ( -28.55116071645519327, 41.05976639056880373, -2.408242355805840784 ) ) ;
#33564=CARTESIAN_POINT ( 'NONE',  ( 0.1287570809895630941, -0.3962735484563133515, 10.00000000000000000 ) ) ;
#33570=CARTESIAN_POINT ( 'NONE',  ( -1.780619886013952602, -1.041246721325602920, 9.886433018048069954 ) ) ;
#33575=AXIS2_PLACEMENT_3D ( 'NONE', #29045, #32912, #44663 ) ;
#33588=CARTESIAN_POINT ( 'NONE',  ( -0.3656201545664206076, 2.182515578491385000, 9.881002359080270026 ) ) ;
#33589=B_SPLINE_CURVE_WITH_KNOTS ( 'NONE', 3,
 ( #16159, #31818, #47403, #32063 ),
 .UNSPECIFIED., .F., .F.,
 ( 4, 4 ),
 ( 0.0004299334430849446756, 0.0007706806524480028925 ),
 .UNSPECIFIED. ) ;
#33602=CARTESIAN_POINT ( 'NONE',  ( -4.207128120815918256E-14, 3.058192377181588826E-14, 10.00000000000000000 ) ) ;
#33603=CARTESIAN_POINT ( 'NONE',  ( 28.52604530808654815, 41.07801380285680892, -3.760136334089591248 ) ) ;
#33629=CARTESIAN_POINT ( 'NONE',  ( 22.69295089195473736, 45.31600496604706052, 7.455576670931136185 ) ) ;
#33630=CARTESIAN_POINT ( 'NONE',  ( 0.3862712429686894766, -1.188820645368940276, 3.333333333333333481 ) ) ;
#33631=CARTESIAN_POINT ( 'NONE',  ( -0.4166666666666664631, 0.000000000000000000, 10.00000000000000000 ) ) ;
#33633=ORIENTED_EDGE ( 'NONE', *, *, #36299, .F. ) ;
#33649=LINE ( 'NONE', #49238, #16733 ) ;
#33653=CARTESIAN_POINT ( 'NONE',  ( 0.2099955233291934398, 1.205406147626143509, 9.993783931180535873 ) ) ;
#33661=CARTESIAN_POINT ( 'NONE',  ( 4.763548243873389154, -16.57409059453848599, 8.727788335465566760 ) ) ;
#33671=CARTESIAN_POINT ( 'NONE',  ( 8.176860274785711979, -5.756644512789521606, 9.282506307616484875 ) ) ;
#33685=CARTESIAN_POINT ( 'NONE',  ( -6.508636631827791064, -15.75743548351446854, 8.953103998512858652 ) ) ;
#33706=B_SPLINE_CURVE_WITH_KNOTS ( 'NONE', 3,
 ( #37743, #41571, #1822, #16969 ),
 .UNSPECIFIED., .F., .F.,
 ( 4, 4 ),
 ( 3.806888117163228439E-16, 0.009762429729296128247 ),
 .UNSPECIFIED. ) ;
#33710=CARTESIAN_POINT ( 'NONE',  ( -48.33712804702535237, -13.03701565032741705, -9.367992836599951190 ) ) ;
#33711=EDGE_CURVE ( 'NONE', #49869, #9153, #3512, .T. ) ;
#33735=EDGE_LOOP ( 'NONE', ( #48980, #38760, #28739, #43338, #47340, #27046, #46371, #25748, #31563, #12024, #14945, #25556, #25825, #17511, #22660, #7038, #29124, #18296, #41312, #16060, #3032, #47680, #45230, #12879, #29328 ) ) ;
#33736=EDGE_LOOP ( 'NONE', ( #37552, #32371, #13550, #2760 ) ) ;
#33745=CARTESIAN_POINT ( 'NONE',  ( -0.9599924130074112272, 0.8495346730527952861, 9.948547179989619238 ) ) ;
#33747=PLANE ( 'NONE',  #36716 ) ;
#33757=CARTESIAN_POINT ( 'NONE',  ( 1.222012661920449439, -0.2471648704738783342, 9.981352469109934233 ) ) ;
#33769=CARTESIAN_POINT ( 'NONE',  ( 2.774199659188286482, 2.805557815409694289, 6.494306517201427376 ) ) ;
#33772=ORIENTED_EDGE ( 'NONE', *, *, #17063, .T. ) ;
#33777=EDGE_CURVE ( 'NONE', #48573, #13052, #38445, .T. ) ;
#33790=CARTESIAN_POINT ( 'NONE',  ( 8.277096487746778308, -50.00000000000000711, 7.455576670931136185 ) ) ;
#33791=EDGE_CURVE ( 'NONE', #49222, #9732, #47572, .T. ) ;
#33801=CARTESIAN_POINT ( 'NONE',  ( -41.53730588968662829, -19.98817461849951016, 8.807470649214881320 ) ) ;
#33805=B_SPLINE_CURVE_WITH_KNOTS ( 'NONE', 3,
 ( #4086, #35154, #16384, #47642 ),
 .UNSPECIFIED., .F., .F.,
 ( 4, 4 ),
 ( 0.000000000000000000, 0.0002610106747150285275 ),
 .UNSPECIFIED. ) ;
#33819=CARTESIAN_POINT ( 'NONE',  ( 0.3862712429686894766, -1.188820645368940276, 10.00000000000000000 ) ) ;
#33835=ORIENTED_EDGE ( 'NONE', *, *, #49699, .F. ) ;
#33836=B_SPLINE_SURFACE_WITH_KNOTS ( 'NONE', 3, 3, ( 
 ( #14638, #6435, #14121, #10787 ),
 ( #2576, #22085, #18222, #48736 ),
 ( #1836, #33157, #49739, #10533 ),
 ( #37759, #26193, #6683, #33901 ) ),
 .UNSPECIFIED., .F., .F., .F.,
 ( 4, 4 ),
 ( 4, 4 ),
 ( 0.000000000000000000, 1.000000000000000000 ),
 ( 0.000000000000000000, 1.000000000000000000 ),
 .UNSPECIFIED. ) ;
#33844=CARTESIAN_POINT ( 'NONE',  ( -0.3862712429686809279, -1.188820645368943163, -3.333333333333333481 ) ) ;
#33857=VERTEX_POINT ( 'NONE', #29338 ) ;
#33859=DIRECTION ( 'NONE',  ( 0.000000000000000000, 0.000000000000000000, -1.000000000000000000 ) ) ;
#33870=CARTESIAN_POINT ( 'NONE',  ( 1.104609456715839766, 0.6504863887005235545, 9.948547179989622791 ) ) ;
#33871=DIRECTION ( 'NONE',  ( 0.000000000000000000, 0.000000000000000000, 1.000000000000000000 ) ) ;
#33872=CARTESIAN_POINT ( 'NONE',  ( -25.60949810002096783, -43.19700938445173932, 1.847720168420772691 ) ) ;
#33877=CARTESIAN_POINT ( 'NONE',  ( -29.61572577327014955, -16.11461842845715253, 8.807470649214879543 ) ) ;
#33881=CARTESIAN_POINT ( 'NONE',  ( -1.011271242968693862, 0.7347315653655780432, 10.00000000000000000 ) ) ;
#33883=CARTESIAN_POINT ( 'NONE',  ( -4.207128120815918256E-14, 3.058192377181588826E-14, 10.00000000000000000 ) ) ;
#33887=ORIENTED_EDGE ( 'NONE', *, *, #17975, .F. ) ;
#33894=ORIENTED_EDGE ( 'NONE', *, *, #13142, .T. ) ;
#33901=CARTESIAN_POINT ( 'NONE',  ( -1.011271242968683426, -0.7347315653655928092, 10.00000000000000000 ) ) ;
#33910=CARTESIAN_POINT ( 'NONE',  ( -0.9341213539222554818, -1.950087977540069684, 9.885585981620945262 ) ) ;
#33916=ORIENTED_EDGE ( 'NONE', *, *, #30306, .T. ) ;
#33943=CARTESIAN_POINT ( 'NONE',  ( 17.23491422248386584, -0.5912720620000816441, 8.727788335465566760 ) ) ;
#33953=CARTESIAN_POINT ( 'NONE',  ( 30.12518629743562926, 14.70074613238908157, 1.847720168420772691 ) ) ;
#33962=CARTESIAN_POINT ( 'NONE',  ( 14.29087950072012170, 9.652079258044652832, 8.727788335465566760 ) ) ;
#33967=CARTESIAN_POINT ( 'NONE',  ( -15.42815683172655028, -34.17926237904570996, 7.697694107796190899 ) ) ;
#33983=CARTESIAN_POINT ( 'NONE',  ( -29.61572577327014955, -16.11461842845715253, 8.807470649214879543 ) ) ;
#33986=EDGE_CURVE ( 'NONE', #15558, #9775, #1091, .T. ) ;
#34003=CARTESIAN_POINT ( 'NONE',  ( -2.188678504086925880, 0.3267089737526900350, 9.881002359080270026 ) ) ;
#34007=CARTESIAN_POINT ( 'NONE',  ( -1.810969182959400570, 3.505385724216297127, 6.494306115487985309 ) ) ;
#34020=CARTESIAN_POINT ( 'NONE',  ( -1.114871695981121125, 0.4953159757245923500, 9.963925895596188909 ) ) ;
#34023=EDGE_CURVE ( 'NONE', #1790, #15177, #30100, .T. ) ;
#34026=CARTESIAN_POINT ( 'NONE',  ( -0.9390173899430289683, -1.130417317737636651, 9.958264684458541183 ) ) ;
#34031=CARTESIAN_POINT ( 'NONE',  ( 6.174150299305392053, -33.14591993373988998, 8.807470649214879543 ) ) ;
#34042=CARTESIAN_POINT ( 'NONE',  ( -1.011271242968693862, 0.7347315653655780432, -10.00000000000000000 ) ) ;
#34051=CARTESIAN_POINT ( 'NONE',  ( -0.3862712429686809279, -1.188820645368943163, -3.333333333333333481 ) ) ;
#34061=CARTESIAN_POINT ( 'NONE',  ( 0.6595498452743703277, -16.59563386392009576, 3.266473740018926541 ) ) ;
#34076=LINE ( 'NONE', #21748, #13047 ) ;
#34084=ORIENTED_EDGE ( 'NONE', *, *, #12993, .F. ) ;
#34085=CARTESIAN_POINT ( 'NONE',  ( -0.4612239888288630074, 1.380789889681132365, 9.938560701278168708 ) ) ;
#34090=CARTESIAN_POINT ( 'NONE',  ( -27.31081730472607561, -41.96092862852123773, 3.199614146704519602 ) ) ;
#34102=CARTESIAN_POINT ( 'NONE',  ( 3.975459390375365665, 0.2195152216756870167, 1.992221491942114397E-15 ) ) ;
#34116=ORIENTED_EDGE ( 'NONE', *, *, #11657, .T. ) ;
#34125=ADVANCED_FACE ( 'NONE', ( #39320 ), #23622, .T. ) ;
#34127=CARTESIAN_POINT ( 'NONE',  ( 11.73320209285708415, -11.96063479729170886, 9.403735324607438884 ) ) ;
#34136=CARTESIAN_POINT ( 'NONE',  ( -36.62549812225767454, -8.082823558958592614, -8.600750091277035381 ) ) ;
#34143=B_SPLINE_CURVE_WITH_KNOTS ( 'NONE', 3,
 ( #10034, #5171, #1587, #25182 ),
 .UNSPECIFIED., .F., .F.,
 ( 4, 4 ),
 ( 0.0009539133080771172290, 0.009404495247862900906 ),
 .UNSPECIFIED. ) ;
#34148=CARTESIAN_POINT ( 'NONE',  ( 47.88254548617766204, -14.43607691413525984, -3.760136334089591248 ) ) ;
#34149=CARTESIAN_POINT ( 'NONE',  ( -0.7757854888975277419, -0.3020624223403916564, 9.985686052694763504 ) ) ;
#34154=EDGE_LOOP ( 'NONE', ( #38400, #36232, #42344, #3332 ) ) ;
#34171=CARTESIAN_POINT ( 'NONE',  ( -16.99749102614300966, 1.320765928724422222, 8.953103998512858652 ) ) ;
#34176=DIRECTION ( 'NONE',  ( -0.8411784753765545464, 0.000000000000000000, 0.5407575913134972101 ) ) ;
#34177=B_SPLINE_CURVE_WITH_KNOTS ( 'NONE', 3,
 ( #45269, #11174, #41955, #30156 ),
 .UNSPECIFIED., .F., .F.,
 ( 4, 4 ),
 ( 2.219577935476692653E-17, 0.0003407397535652598392 ),
 .UNSPECIFIED. ) ;
#34181=CARTESIAN_POINT ( 'NONE',  ( 35.51846793572394034, -35.99772139009119343, 7.906207997025717304 ) ) ;
#34185=ORIENTED_EDGE ( 'NONE', *, *, #29770, .T. ) ;
#34187=CARTESIAN_POINT ( 'NONE',  ( 1.011271242968683648, 0.7347315653655930312, 10.00000000000000000 ) ) ;
#34200=EDGE_LOOP ( 'NONE', ( #33887, #28475, #37891, #24433 ) ) ;
#34225=ORIENTED_EDGE ( 'NONE', *, *, #37911, .T. ) ;
#34245=CARTESIAN_POINT ( 'NONE',  ( 0.3370904143228947158, 0.2449105217885311492, 10.00000000000000000 ) ) ;
#34247=CARTESIAN_POINT ( 'NONE',  ( -1.011271242968693862, 0.7347315653655780432, 10.00000000000000000 ) ) ;
#34255=B_SPLINE_SURFACE_WITH_KNOTS ( 'NONE', 3, 3, ( 
 ( #31307, #47647, #3570, #4601 ),
 ( #11544, #23589, #42820, #35674 ),
 ( #19215, #20244, #35159, #50484 ),
 ( #27947, #15391, #7693, #1 ) ),
 .UNSPECIFIED., .F., .F., .F.,
 ( 4, 4 ),
 ( 4, 4 ),
 ( 0.000000000000000000, 1.000000000000000000 ),
 ( 0.000000000000000000, 1.000000000000000000 ),
 .UNSPECIFIED. ) ;
#34259=CARTESIAN_POINT ( 'NONE',  ( -0.5111101921243752511, -1.175566515482119989, 9.957892297621015132 ) ) ;
#34267=CARTESIAN_POINT ( 'NONE',  ( 33.16902712922644270, -37.70469005304286725, 1.847720168420772691 ) ) ;
#34274=CARTESIAN_POINT ( 'NONE',  ( -1.158497635116737312, 16.61944452314319420, -3.546734833711462365 ) ) ;
#34294=EDGE_LOOP ( 'NONE', ( #49975, #2464, #37107, #10735, #32924, #48021, #14900, #10480, #39263, #39128, #31876, #14720, #40849, #45442 ) ) ;
#34298=CARTESIAN_POINT ( 'NONE',  ( -0.4402948852767746279, 2.015117899693936732, 9.894754715216722118 ) ) ;
#34302=CARTESIAN_POINT ( 'NONE',  ( 6.174150299305392053, -50.00000000000000711, 8.807470649214879543 ) ) ;
#34303=ORIENTED_EDGE ( 'NONE', *, *, #5807, .T. ) ;
#34306=CARTESIAN_POINT ( 'NONE',  ( 1.011271242968694084, -0.7347315653655782652, 3.333333333333333481 ) ) ;
#34315=CARTESIAN_POINT ( 'NONE',  ( 10.70590866674922204, -12.76446523155706814, -3.546734833711462365 ) ) ;
#34332=CARTESIAN_POINT ( 'NONE',  ( -3.345242017215803276, 2.159124855890678596, -2.642742795433417058E-16 ) ) ;
#34337=ORIENTED_EDGE ( 'NONE', *, *, #14219, .F. ) ;
#34351=CARTESIAN_POINT ( 'NONE',  ( -34.08406891383351933, 15.63733501198486309, -8.192531242611266862 ) ) ;
#34356=CARTESIAN_POINT ( 'NONE',  ( 1.011271242968688311, -0.7347315653655854817, 9.972675548442463622 ) ) ;
#34361=CARTESIAN_POINT ( 'NONE',  ( 22.69295089195473736, 45.31600496604706052, 7.455576670931136185 ) ) ;
#34382=CARTESIAN_POINT ( 'NONE',  ( -10.69268279052439574, -12.77266927778454964, -2.870787844569587133 ) ) ;
#34386=CARTESIAN_POINT ( 'NONE',  ( -1.448406091252275818, 0.9360325558308429938, 9.928159647716187308 ) ) ;
#34405=ORIENTED_EDGE ( 'NONE', *, *, #33986, .T. ) ;
#34413=EDGE_CURVE ( 'NONE', #1069, #9737, #38990, .T. ) ;
#34423=CARTESIAN_POINT ( 'NONE',  ( 1.104213410210670876, 0.6509177773818231039, 9.976582533991679824 ) ) ;
#34429=CARTESIAN_POINT ( 'NONE',  ( -32.57170742938676256, -18.58316106410400437, 7.697694107796192675 ) ) ;
#34435=CARTESIAN_POINT ( 'NONE',  ( -7.749480817862350435, -14.85497772329513211, 9.403735324607438884 ) ) ;
#34436=CARTESIAN_POINT ( 'NONE',  ( -13.59579750444763668, 10.60877755095910935, 8.727788335465566760 ) ) ;
#34441=CARTESIAN_POINT ( 'NONE',  ( 7.608425291889091113, -36.72004717559254772, 7.697694107796188234 ) ) ;
#34448=CARTESIAN_POINT ( 'NONE',  ( -0.3862712429686729343, -1.188820645368946050, -10.00000000000000000 ) ) ;
#34455=CARTESIAN_POINT ( 'NONE',  ( 5.888214538810389698, 16.20866436362417673, 8.727788335465566760 ) ) ;
#34486=CARTESIAN_POINT ( 'NONE',  ( -30.12518629743573584, -14.70074613238887551, 1.847720168420772691 ) ) ;
#34489=CARTESIAN_POINT ( 'NONE',  ( 4.672045878990125800, -50.00000000000000711, 1.847720168420772691 ) ) ;
#34501=CARTESIAN_POINT ( 'NONE',  ( -1.011271242968683426, -0.7347315653655928092, 10.00000000000000000 ) ) ;
#34507=CARTESIAN_POINT ( 'NONE',  ( -27.73884755486766096, 25.23502201956265978, 7.697694107796191787 ) ) ;
#34511=CARTESIAN_POINT ( 'NONE',  ( 0.3862712429686810944, 1.188820645368943607, -10.00000000000000000 ) ) ;
#34513=B_SPLINE_CURVE_WITH_KNOTS ( 'NONE', 3,
 ( #22926, #10616, #7280, #41924 ),
 .UNSPECIFIED., .F., .F.,
 ( 4, 4 ),
 ( 0.000000000000000000, 0.001246897409371951551 ),
 .UNSPECIFIED. ) ;
#34517=B_SPLINE_CURVE_WITH_KNOTS ( 'NONE', 3,
 ( #15073, #34085, #38438, #18405 ),
 .UNSPECIFIED., .F., .F.,
 ( 4, 4 ),
 ( 0.0006664118838822479917, 0.001081796195657045356 ),
 .UNSPECIFIED. ) ;
#34522=CARTESIAN_POINT ( 'NONE',  ( 12.15085308559846844, -11.68662139125803989, 2.590526750877053086 ) ) ;
#34523=CARTESIAN_POINT ( 'NONE',  ( -22.69295089195507487, -45.31600496604688999, 7.455576670931136185 ) ) ;
#34526=VERTEX_POINT ( 'NONE', #22830 ) ;
#34527=CIRCLE ( 'NONE', #20566, 10.00000000000000000 ) ;
#34529=CARTESIAN_POINT ( 'NONE',  ( -6.174150299305392053, 50.00000000000000711, 8.807470649214879543 ) ) ;
#34530=CARTESIAN_POINT ( 'NONE',  ( -0.1425549192113998442, 1.238581250503548059, 9.981352469109934233 ) ) ;
#34531=ORIENTED_EDGE ( 'NONE', *, *, #49343, .T. ) ;
#34560=DIRECTION ( 'NONE',  ( 0.000000000000000000, 0.000000000000000000, -1.000000000000000000 ) ) ;
#34568=CARTESIAN_POINT ( 'NONE',  ( 30.87089393895375267, -12.69923079256617449, -9.367992836599954742 ) ) ;
#34572=FACE_OUTER_BOUND ( 'NONE', #48089, .T. ) ;
#34576=ORIENTED_EDGE ( 'NONE', *, *, #23979, .T. ) ;
#34581=CARTESIAN_POINT ( 'NONE',  ( 4.641001526964561918, 50.00000000000000711, -8.016098858316205167 ) ) ;
#34585=CARTESIAN_POINT ( 'NONE',  ( -23.31729631074215092, -24.19776167542410406, -8.016098858316199838 ) ) ;
#34592=CARTESIAN_POINT ( 'NONE',  ( -0.3862712429686809279, -1.188820645368943163, 3.333333333333333481 ) ) ;
#34603=CARTESIAN_POINT ( 'NONE',  ( 1.011271242968688311, -0.7347315653655854817, 9.972675548442463622 ) ) ;
#34618=CARTESIAN_POINT ( 'NONE',  ( -2.462075149652696027, 16.57295996686994499, 9.403735324607438884 ) ) ;
#34627=ADVANCED_FACE ( 'NONE', ( #7191 ), #19933, .T. ) ;
#34635=CARTESIAN_POINT ( 'NONE',  ( -2.242409830259191494, 37.46921084408874947, 3.209567239418970708 ) ) ;
#34642=CARTESIAN_POINT ( 'NONE',  ( 50.11058929355270664, -7.578863168071591438, 7.455576670931136185 ) ) ;
#34652=ORIENTED_EDGE ( 'NONE', *, *, #45443, .T. ) ;
#34654=ADVANCED_FACE ( 'NONE', ( #1270 ), #12167, .T. ) ;
#34657=EDGE_CURVE ( 'NONE', #50425, #24051, #37182, .T. ) ;
#34658=VERTEX_POINT ( 'NONE', #32575 ) ;
#34668=CARTESIAN_POINT ( 'NONE',  ( -6.619412807845042046, 7.495556955913086128, 9.646707543097347681 ) ) ;
#34677=DIRECTION ( 'NONE',  ( -0.5877852522924802425, 0.8090169943749422332, 0.000000000000000000 ) ) ;
#34682=B_SPLINE_SURFACE_WITH_KNOTS ( 'NONE', 3, 3, ( 
 ( #45543, #17862, #25573, #37148 ),
 ( #6829, #18360, #5817, #14263 ),
 ( #10423, #10672, #22475, #2962 ),
 ( #49623, #13756, #18116, #34042 ) ),
 .UNSPECIFIED., .F., .F., .F.,
 ( 4, 4 ),
 ( 4, 4 ),
 ( 0.000000000000000000, 1.000000000000000000 ),
 ( 0.000000000000000000, 1.000000000000000000 ),
 .UNSPECIFIED. ) ;
#34693=CARTESIAN_POINT ( 'NONE',  ( 29.61572577327002520, 16.11461842845735859, 8.807470649214879543 ) ) ;
#34695=ORIENTED_EDGE ( 'NONE', *, *, #32277, .F. ) ;
#34698=CARTESIAN_POINT ( 'NONE',  ( -9.999999999999994671, -1.598124844265358068E-11, 9.303249460319950259 ) ) ;
#34703=VECTOR ( 'NONE', #1954, 1000.000000000000000 ) ;
#34708=CARTESIAN_POINT ( 'NONE',  ( 15.45175104485250728, -6.222373774239001065, -2.870787844569587133 ) ) ;
#34727=CARTESIAN_POINT ( 'NONE',  ( 0.8065422446123827749, -0.2117385185661261604, 9.985671801905168010 ) ) ;
#34731=CARTESIAN_POINT ( 'NONE',  ( 16.02661358026014327, 4.530191650547718218, -9.683996418299976483 ) ) ;
#34739=ORIENTED_EDGE ( 'NONE', *, *, #45443, .F. ) ;
#34752=CARTESIAN_POINT ( 'NONE',  ( -23.13346437080424778, 39.73622551878982989, -8.016098858316205167 ) ) ;
#34759=CARTESIAN_POINT ( 'NONE',  ( 0.09523839817332763191, 1.466467394239034050, 9.958264684458713489 ) ) ;
#34769=AXIS2_PLACEMENT_3D ( 'NONE', #21990, #26089, #34560 ) ;
#34771=CARTESIAN_POINT ( 'NONE',  ( 8.277096487746778308, -50.00000000000000711, 7.455576670931136185 ) ) ;
#34779=EDGE_CURVE ( 'NONE', #10187, #32574, #48102, .T. ) ;
#34781=CARTESIAN_POINT ( 'NONE',  ( -1.540526284687967706, 1.371707213411501147, 9.886433018048069954 ) ) ;
#34783=AXIS2_PLACEMENT_3D ( 'NONE', #15026, #38141, #49854 ) ;
#34791=ORIENTED_EDGE ( 'NONE', *, *, #16684, .F. ) ;
#34793=CARTESIAN_POINT ( 'NONE',  ( -28.52604530808686079, -41.07801380285659576, -3.760136334089591248 ) ) ;
#34815=CARTESIAN_POINT ( 'NONE',  ( 1.080340181645069064, -0.5751155560365959207, 9.966990753365129407 ) ) ;
#34822=ORIENTED_EDGE ( 'NONE', *, *, #6840, .T. ) ;
#34841=CARTESIAN_POINT ( 'NONE',  ( 8.277096487746778308, -50.00000000000000711, 7.455576670931136185 ) ) ;
#34862=CARTESIAN_POINT ( 'NONE',  ( 0.2455008416098105606, 1.553107091521340966, 9.945241992664895392 ) ) ;
#34863=DIRECTION ( 'NONE',  ( 0.000000000000000000, 0.000000000000000000, -1.000000000000000000 ) ) ;
#34889=CARTESIAN_POINT ( 'NONE',  ( -9.999999999999994671, -1.598124844265358068E-11, 9.303249460319950259 ) ) ;
#34891=CARTESIAN_POINT ( 'NONE',  ( -31.44259251615275019, -38.95901822126145220, -9.367992836599954742 ) ) ;
#34892=B_SPLINE_CURVE_WITH_KNOTS ( 'NONE', 3,
 ( #21150, #36832, #1660, #13451 ),
 .UNSPECIFIED., .F., .F.,
 ( 4, 4 ),
 ( 0.9811748202683396869, 0.9878904167554125593 ),
 .UNSPECIFIED. ) ;
#34903=CARTESIAN_POINT ( 'NONE',  ( -45.64490844644706868, -21.32281559348764333, 8.807470649214879543 ) ) ;
#34920=ADVANCED_FACE ( 'NONE', ( #14816 ), #42854, .T. ) ;
#34927=CARTESIAN_POINT ( 'NONE',  ( -23.29043492822808759, 24.10797434788186067, 1.847720168420772691 ) ) ;
#34928=CARTESIAN_POINT ( 'NONE',  ( 34.91952936320839740, -13.67027684621004546, -9.422646554964178023 ) ) ;
#34930=ORIENTED_EDGE ( 'NONE', *, *, #1979, .F. ) ;
#34934=EDGE_CURVE ( 'NONE', #3137, #50500, #15065, .T. ) ;
#34946=FACE_BOUND ( 'NONE', #19578, .T. ) ;
#34952=ORIENTED_EDGE ( 'NONE', *, *, #36038, .T. ) ;
#34953=CARTESIAN_POINT ( 'NONE',  ( 47.88254548617766204, -14.43607691413525984, -3.760136334089591248 ) ) ;
#34957=ADVANCED_FACE ( 'NONE', ( #21134 ), #8076, .T. ) ;
#34980=CARTESIAN_POINT ( 'NONE',  ( 13.92102703536701114, 30.85732372859822803, 8.356839323120299312 ) ) ;
#34983=CARTESIAN_POINT ( 'NONE',  ( 1.250000000000000222, 0.000000000000000000, 10.00000000000000000 ) ) ;
#34991=EDGE_CURVE ( 'NONE', #38289, #29160, #32689, .T. ) ;
#34998=CARTESIAN_POINT ( 'NONE',  ( 15.42815683172628738, 34.17926237904582365, 7.697694107796191787 ) ) ;
#35009=VERTEX_POINT ( 'NONE', #14447 ) ;
#35014=CARTESIAN_POINT ( 'NONE',  ( 1.066995270233474624, -50.00000000000000711, -3.760136334089591248 ) ) ;
#35021=ORIENTED_EDGE ( 'NONE', *, *, #18868, .T. ) ;
#35026=DIRECTION ( 'NONE',  ( 1.000000000000000000, 0.000000000000000000, 0.000000000000000000 ) ) ;
#35028=CARTESIAN_POINT ( 'NONE',  ( -0.3370904143228978245, 0.2449105217885259589, 10.00000000000000000 ) ) ;
#35035=B_SPLINE_CURVE_WITH_KNOTS ( 'NONE', 3,
 ( #9837, #5734, #21640, #44716 ),
 .UNSPECIFIED., .F., .F.,
 ( 4, 4 ),
 ( 0.000000000000000000, 0.2637263876330695478 ),
 .UNSPECIFIED. ) ;
#35036=CARTESIAN_POINT ( 'NONE',  ( -26.42016489236612387, -32.24895757977012067, -9.387872844313825738 ) ) ;
#35056=CARTESIAN_POINT ( 'NONE',  ( 4.763548243873389154, -16.57409059453848599, 8.727788335465566760 ) ) ;
#35058=EDGE_CURVE ( 'NONE', #45646, #41656, #25446, .T. ) ;
#35063=FACE_OUTER_BOUND ( 'NONE', #20804, .T. ) ;
#35071=ADVANCED_FACE ( 'NONE', ( #6744 ), #23198, .T. ) ;
#35074=FACE_OUTER_BOUND ( 'NONE', #27341, .T. ) ;
#35077=VERTEX_POINT ( 'NONE', #30610 ) ;
#35080=EDGE_CURVE ( 'NONE', #20716, #45083, #48028, .T. ) ;
#35089=CARTESIAN_POINT ( 'NONE',  ( 0.9390173899407876501, 1.130417317737878458, 9.958264684458711713 ) ) ;
#35097=CARTESIAN_POINT ( 'NONE',  ( 8.813458710706171928, 4.724716452304571490, 0.000000000000000000 ) ) ;
#35099=DIRECTION ( 'NONE',  ( 0.000000000000000000, 0.000000000000000000, -1.000000000000000000 ) ) ;
#35100=EDGE_CURVE ( 'NONE', #30729, #34658, #38282, .T. ) ;
#35104=ORIENTED_EDGE ( 'NONE', *, *, #18204, .T. ) ;
#35106=CARTESIAN_POINT ( 'NONE',  ( 5.951573025415589413, -0.3107723916541159093, 1.992221491942114397E-15 ) ) ;
#35111=B_SPLINE_SURFACE_WITH_KNOTS ( 'NONE', 3, 3, ( 
 ( #36579, #4483, #904, #16546 ),
 ( #20130, #35821, #32199, #47798 ),
 ( #12683, #28344, #16796, #32458 ),
 ( #24499, #43975, #8843, #40148 ) ),
 .UNSPECIFIED., .F., .F., .F.,
 ( 4, 4 ),
 ( 4, 4 ),
 ( 0.000000000000000000, 1.000000000000000000 ),
 ( 0.000000000000000000, 1.000000000000000000 ),
 .UNSPECIFIED. ) ;
#35112=B_SPLINE_CURVE_WITH_KNOTS ( 'NONE', 3,
 ( #2111, #17758, #33424, #48997 ),
 .UNSPECIFIED., .F., .F.,
 ( 4, 4 ),
 ( 0.0001535465953326577474, 0.0005837444810855837779 ),
 .UNSPECIFIED. ) ;
#35114=ORIENTED_EDGE ( 'NONE', *, *, #42205, .T. ) ;
#35120=LINE ( 'NONE', #50172, #5751 ) ;
#35131=CARTESIAN_POINT ( 'NONE',  ( 25.61277432017878297, -22.36370378792834757, 7.906207997025717304 ) ) ;
#35142=FACE_OUTER_BOUND ( 'NONE', #48625, .T. ) ;
#35147=DIRECTION ( 'NONE',  ( 1.000000000000000000, 0.000000000000000000, 0.000000000000000000 ) ) ;
#35152=CARTESIAN_POINT ( 'NONE',  ( -0.5113015165352315927, -1.175527691268679398, 9.948547179989621014 ) ) ;
#35154=CARTESIAN_POINT ( 'NONE',  ( -0.9460392030597363222, -0.7922402054911648062, 9.969907203203806745 ) ) ;
#35155=VERTEX_POINT ( 'NONE', #38829 ) ;
#35156=CARTESIAN_POINT ( 'NONE',  ( -0.1469336902871204442, -1.496274467947957376, 9.953784399990622589 ) ) ;
#35159=CARTESIAN_POINT ( 'NONE',  ( 15.44803555374680393, 6.237487519713364570, -3.546734833711462365 ) ) ;
#35160=EDGE_CURVE ( 'NONE', #29819, #17812, #32822, .T. ) ;
#35165=CARTESIAN_POINT ( 'NONE',  ( 0.1471466405374506625, 1.496299042407936319, 9.944962737436833677 ) ) ;
#35180=CARTESIAN_POINT ( 'NONE',  ( -6.174150299305392053, 50.00000000000000000, 8.807470649214879543 ) ) ;
#35186=CARTESIAN_POINT ( 'NONE',  ( -1.142975459103954705, -16.61830776097024653, -2.870787844569587133 ) ) ;
#35188=ORIENTED_EDGE ( 'NONE', *, *, #49601, .F. ) ;
#35195=CARTESIAN_POINT ( 'NONE',  ( -48.55374341718683695, -12.37034209168234256, -8.917361510505369182 ) ) ;
#35212=CARTESIAN_POINT ( 'NONE',  ( -1.011271242968693862, 0.7347315653655780432, -10.00000000000000000 ) ) ;
#35214=CARTESIAN_POINT ( 'NONE',  ( 16.52264463346132572, -2.779753662172757878, 9.403735324607438884 ) ) ;
#35221=CARTESIAN_POINT ( 'NONE',  ( 7.749480817862238524, 14.85497772329518895, 9.403735324607438884 ) ) ;
#35224=CARTESIAN_POINT ( 'NONE',  ( 7.359817328027030925, 15.16751262232805431, 2.590526750877053086 ) ) ;
#35225=CARTESIAN_POINT ( 'NONE',  ( 1.011271242968694084, -0.7347315653655782652, -10.00000000000000000 ) ) ;
#35250=CARTESIAN_POINT ( 'NONE',  ( -31.28234235046239320, -11.28615439405757392, -3.760136334089591248 ) ) ;
#35255=B_SPLINE_CURVE_WITH_KNOTS ( 'NONE', 3,
 ( #27468, #38771, #3597, #19241 ),
 .UNSPECIFIED., .F., .F.,
 ( 4, 4 ),
 ( 4.906538933386796626E-18, 0.002458791966311094177 ),
 .UNSPECIFIED. ) ;
#35261=B_SPLINE_CURVE_WITH_KNOTS ( 'NONE', 3,
 ( #37931, #29966, #17887, #46069 ),
 .UNSPECIFIED., .F., .F.,
 ( 4, 4 ),
 ( 1.735570302229820823E-18, 2.804146970186932944E-05 ),
 .UNSPECIFIED. ) ;
#35264=ORIENTED_EDGE ( 'NONE', *, *, #22690, .T. ) ;
#35279=CARTESIAN_POINT ( 'NONE',  ( -36.08557433729204433, 35.58569447144795106, 7.455576670931136185 ) ) ;
#35283=CARTESIAN_POINT ( 'NONE',  ( -47.87295225382221275, -14.46560184742400423, -2.408242355805840784 ) ) ;
#35293=CARTESIAN_POINT ( 'NONE',  ( -0.1469336902871204442, -1.496274467947957376, 9.953784399990622589 ) ) ;
#35313=CARTESIAN_POINT ( 'NONE',  ( -7.576114424932982594, 50.00000000000000711, 7.906207997025717304 ) ) ;
#35323=ORIENTED_EDGE ( 'NONE', *, *, #33711, .T. ) ;
#35324=CARTESIAN_POINT ( 'NONE',  ( 1.080000014128428498, 0.7606467978644730898, 9.943883492372853183 ) ) ;
#35333=ORIENTED_EDGE ( 'NONE', *, *, #43824, .F. ) ;
#35335=CARTESIAN_POINT ( 'NONE',  ( -0.3862712429686809279, -1.188820645368943163, 10.00000000000000000 ) ) ;
#35343=LINE ( 'NONE', #15813, #8529 ) ;
#35378=B_SPLINE_CURVE_WITH_KNOTS ( 'NONE', 3,
 ( #40069, #13101, #12853, #25417 ),
 .UNSPECIFIED., .F., .F.,
 ( 4, 4 ),
 ( 0.9895749839358300992, 1.000000000000000000 ),
 .UNSPECIFIED. ) ;
#35390=CARTESIAN_POINT ( 'NONE',  ( 12.16428377685533135, 11.73151505502934988, -9.008049429158100807 ) ) ;
#35394=CARTESIAN_POINT ( 'NONE',  ( -12.15085308559838317, 11.68662139125813226, 2.590526750877053086 ) ) ;
#35401=CARTESIAN_POINT ( 'NONE',  ( 1.760168014277346593, 0.8403809255487892926, 9.896382706792421047 ) ) ;
#35403=CARTESIAN_POINT ( 'NONE',  ( 0.9602803029231544718, -0.8490247040095941777, 9.976582533991681601 ) ) ;
#35405=EDGE_CURVE ( 'NONE', #36298, #5197, #22836, .T. ) ;
#35409=EDGE_LOOP ( 'NONE', ( #391, #40203, #12082, #43159 ) ) ;
#35422=CARTESIAN_POINT ( 'NONE',  ( 0.1473596192803392213, 1.496323530725627515, 9.936141075511205401 ) ) ;
#35428=CARTESIAN_POINT ( 'NONE',  ( 32.92553608936638199, 17.96298651181805894, 8.100132398494515940 ) ) ;
#35441=CARTESIAN_POINT ( 'NONE',  ( 2.569099690548740877, -50.00000000000000711, 3.199614146704519602 ) ) ;
#35443=STYLED_ITEM('',(#50761),#5361);
#35456=ORIENTED_EDGE ( 'NONE', *, *, #40853, .T. ) ;
#35457=CARTESIAN_POINT ( 'NONE',  ( 30.87089393895375267, -12.69923079256617449, -9.367992836599954742 ) ) ;
#35464=CARTESIAN_POINT ( 'NONE',  ( -1.249999999999999778, 0.000000000000000000, 10.00000000000000000 ) ) ;
#35475=PLANE ( 'NONE',  #6487 ) ;
#35478=CARTESIAN_POINT ( 'NONE',  ( -7.129058724845069861, -15.30620660340479766, 9.178419661560148768 ) ) ;
#35501=VERTEX_POINT ( 'NONE', #26698 ) ;
#35507=CARTESIAN_POINT ( 'NONE',  ( -1.249999999999999778, 0.000000000000000000, 3.333333333333333481 ) ) ;
#35516=CARTESIAN_POINT ( 'NONE',  ( 0.1287570809895630941, -0.3962735484563133515, 10.00000000000000000 ) ) ;
#35528=CARTESIAN_POINT ( 'NONE',  ( 1.066995270233474624, -50.00000000000000711, -3.760136334089591248 ) ) ;
#35529=ORIENTED_EDGE ( 'NONE', *, *, #33711, .F. ) ;
#35532=B_SPLINE_SURFACE_WITH_KNOTS ( 'NONE', 3, 3, ( 
 ( #8509, #39815, #31617, #4656 ),
 ( #40062, #47203, #39560, #565 ),
 ( #12102, #8250, #36218, #4396 ),
 ( #44133, #20045, #16200, #31864 ) ),
 .UNSPECIFIED., .F., .F., .F.,
 ( 4, 4 ),
 ( 4, 4 ),
 ( 0.000000000000000000, 1.000000000000000000 ),
 ( 0.000000000000000000, 1.000000000000000000 ),
 .UNSPECIFIED. ) ;
#35535=B_SPLINE_CURVE_WITH_KNOTS ( 'NONE', 3,
 ( #37004, #48468, #9264, #5660 ),
 .UNSPECIFIED., .F., .F.,
 ( 4, 4 ),
 ( 0.0001535465953326810848, 0.0005837444810856193397 ),
 .UNSPECIFIED. ) ;
#35537=CARTESIAN_POINT ( 'NONE',  ( 0.1287570809895630941, -0.3962735484563133515, 10.00000000000000000 ) ) ;
#35554=CARTESIAN_POINT ( 'NONE',  ( 14.48769039275578407, 30.44468701195595983, 8.807470649214879543 ) ) ;
#35578=CARTESIAN_POINT ( 'NONE',  ( -1.250000000000000222, 0.000000000000000000, -3.333333333333333481 ) ) ;
#35581=ORIENTED_EDGE ( 'NONE', *, *, #44603, .F. ) ;
#35591=CARTESIAN_POINT ( 'NONE',  ( 4.339432828817248122, 37.24807810779213213, -8.192531242611266862 ) ) ;
#35604=CARTESIAN_POINT ( 'NONE',  ( -0.6595498452743703277, 16.59563386392009576, 3.266473740018926541 ) ) ;
#35614=CARTESIAN_POINT ( 'NONE',  ( -3.808200756227646089, -0.8261963378076270237, 9.741991644047246268 ) ) ;
#35641=ORIENTED_EDGE ( 'NONE', *, *, #28761, .T. ) ;
#35655=LINE ( 'NONE', #46332, #19782 ) ;
#35656=CARTESIAN_POINT ( 'NONE',  ( -0.09523839817533703844, -1.466467394240187350, 9.958264684458541183 ) ) ;
#35661=B_SPLINE_CURVE_WITH_KNOTS ( 'NONE', 3,
 ( #42543, #41549, #45860, #18941 ),
 .UNSPECIFIED., .F., .F.,
 ( 4, 4 ),
 ( 0.0009679537044785101619, 0.001281751046851273322 ),
 .UNSPECIFIED. ) ;
#35663=CARTESIAN_POINT ( 'NONE',  ( 1.365263087672787590, -0.5437404457008400138, 9.958264684458717042 ) ) ;
#35669=ORIENTED_EDGE ( 'NONE', *, *, #17830, .T. ) ;
#35673=VECTOR ( 'NONE', #15369, 1000.000000000000000 ) ;
#35674=CARTESIAN_POINT ( 'NONE',  ( -0.3862712429686977478, 1.188820645368937390, 3.333333333333333481 ) ) ;
#35677=CARTESIAN_POINT ( 'NONE',  ( 50.11058929355270664, -7.578863168071591438, 7.455576670931136185 ) ) ;
#35692=FACE_OUTER_BOUND ( 'NONE', #16040, .T. ) ;
#35711=CARTESIAN_POINT ( 'NONE',  ( -1.104213410210672430, -0.6509177773818179968, 9.976582533991678048 ) ) ;
#35717=ORIENTED_EDGE ( 'NONE', *, *, #31504, .T. ) ;
#35719=CARTESIAN_POINT ( 'NONE',  ( 29.39982726364966581, 16.78152490921169360, 8.356839323120299312 ) ) ;
#35721=CARTESIAN_POINT ( 'NONE',  ( -26.18032376592659105, 21.95228666728381128, 7.455576670931136185 ) ) ;
#35726=CARTESIAN_POINT ( 'NONE',  ( -7.787881821992606035, -1.707024098816393165, -7.318364664277154930E-16 ) ) ;
#35735=CARTESIAN_POINT ( 'NONE',  ( 7.608425291889091113, -36.72004717559254772, 7.697694107796188234 ) ) ;
#35743=CARTESIAN_POINT ( 'NONE',  ( 22.69295089195473736, 45.31600496604706052, 7.455576670931136185 ) ) ;
#35752=EDGE_LOOP ( 'NONE', ( #44249, #31105, #43463 ) ) ;
#35767=ORIENTED_EDGE ( 'NONE', *, *, #7975, .T. ) ;
#35768=CARTESIAN_POINT ( 'NONE',  ( 1.011271242968688311, -0.7347315653655855927, -3.333333333333333481 ) ) ;
#35770=B_SPLINE_CURVE_WITH_KNOTS ( 'NONE', 3,
 ( #48367, #1721, #17613, #33526 ),
 .UNSPECIFIED., .F., .F.,
 ( 4, 4 ),
 ( 0.001937412222931650689, 0.003978261222106149742 ),
 .UNSPECIFIED. ) ;
#35774=CARTESIAN_POINT ( 'NONE',  ( -4.763548243873389154, 16.57409059453848599, 8.727788335465566760 ) ) ;
#35814=CARTESIAN_POINT ( 'NONE',  ( 1.249999999999999778, -0.000000000000000000, -3.333333333333333481 ) ) ;
#35821=CARTESIAN_POINT ( 'NONE',  ( 31.28977333267368621, -11.25592690310905652, -2.408242355805840784 ) ) ;
#35823=ORIENTED_EDGE ( 'NONE', *, *, #35160, .F. ) ;
#35828=ORIENTED_EDGE ( 'NONE', *, *, #27760, .F. ) ;
#35830=ORIENTED_EDGE ( 'NONE', *, *, #19620, .T. ) ;
#35832=ORIENTED_EDGE ( 'NONE', *, *, #11819, .T. ) ;
#35834=LINE ( 'NONE', #8109, #31202 ) ;
#35836=ORIENTED_EDGE ( 'NONE', *, *, #14219, .T. ) ;
#35839=CARTESIAN_POINT ( 'NONE',  ( -25.60949810002096783, -43.19700938445173932, 1.847720168420772691 ) ) ;
#35840=CARTESIAN_POINT ( 'NONE',  ( 0.3862712429686978033, -1.188820645368937834, 10.00000000000000000 ) ) ;
#35841=ORIENTED_EDGE ( 'NONE', *, *, #24923, .T. ) ;
#35842=ORIENTED_EDGE ( 'NONE', *, *, #34657, .F. ) ;
#35843=CARTESIAN_POINT ( 'NONE',  ( -30.87089393895367451, 12.69923079256638232, -9.367992836599951190 ) ) ;
#35849=ORIENTED_EDGE ( 'NONE', *, *, #14281, .T. ) ;
#35880=CARTESIAN_POINT ( 'NONE',  ( -7.359817328027146388, -15.16751262232800102, 2.590526750877053086 ) ) ;
#35893=CARTESIAN_POINT ( 'NONE',  ( -20.40054609052957701, 26.26366202847989229, -3.760136334089591248 ) ) ;
#35938=CARTESIAN_POINT ( 'NONE',  ( -27.33593271309441874, 41.94268121623345991, -9.367992836599951190 ) ) ;
#35940=ORIENTED_EDGE ( 'NONE', *, *, #25279, .T. ) ;
#35950=B_SPLINE_SURFACE_WITH_KNOTS ( 'NONE', 3, 3, ( 
 ( #34361, #21795, #30251, #22796 ),
 ( #26657, #38476, #3286, #18687 ),
 ( #33603, #45853, #49944, #18182 ),
 ( #10739, #6143, #50191, #29743 ) ),
 .UNSPECIFIED., .F., .F., .F.,
 ( 4, 4 ),
 ( 4, 4 ),
 ( 0.000000000000000000, 1.000000000000000000 ),
 ( 0.000000000000000000, 1.000000000000000000 ),
 .UNSPECIFIED. ) ;
#35959=CARTESIAN_POINT ( 'NONE',  ( 1.011271242968683648, 0.7347315653655930312, 10.00000000000000000 ) ) ;
#35973=CARTESIAN_POINT ( 'NONE',  ( 1.086995624458622967, -37.52050741145076529, -3.721387749823088953 ) ) ;
#35974=CARTESIAN_POINT ( 'NONE',  ( 0.5113015165352333691, 1.175527691268683395, 9.948547179989619238 ) ) ;
#35977=FACE_BOUND ( 'NONE', #28267, .T. ) ;
#35987=ORIENTED_EDGE ( 'NONE', *, *, #6406, .F. ) ;
#35988=B_SPLINE_CURVE_WITH_KNOTS ( 'NONE', 3,
 ( #38151, #37401, #30172, #10923 ),
 .UNSPECIFIED., .F., .F.,
 ( 4, 4 ),
 ( 3.878959614448864246E-18, 0.002458791966311092876 ),
 .UNSPECIFIED. ) ;
#35989=EDGE_CURVE ( 'NONE', #11925, #39413, #35120, .T. ) ;
#35991=B_SPLINE_CURVE_WITH_KNOTS ( 'NONE', 3,
 ( #17974, #41340, #33653, #49744 ),
 .UNSPECIFIED., .F., .F.,
 ( 4, 4 ),
 ( 0.9895749839358296551, 1.000000000000000000 ),
 .UNSPECIFIED. ) ;
#36010=CARTESIAN_POINT ( 'NONE',  ( 15.42815683172628738, 34.17926237904582365, 7.697694107796191787 ) ) ;
#36026=CARTESIAN_POINT ( 'NONE',  ( 0.3862712429686894766, -1.188820645368940276, -3.333333333333333481 ) ) ;
#36029=CARTESIAN_POINT ( 'NONE',  ( 1.782521105131670724, -0.3635605703593869920, 9.903764339332079558 ) ) ;
#36038=EDGE_CURVE ( 'NONE', #45415, #31206, #43694, .T. ) ;
#36055=EDGE_CURVE ( 'NONE', #39166, #12051, #45485, .T. ) ;
#36060=CARTESIAN_POINT ( 'NONE',  ( 7.129058724844953510, 15.30620660340485095, 9.178419661560148768 ) ) ;
#36062=VERTEX_POINT ( 'NONE', #5301 ) ;
#36064=CARTESIAN_POINT ( 'NONE',  ( 28.96803024440893992, 18.11533787072037072, 7.455576670931136185 ) ) ;
#36073=CARTESIAN_POINT ( 'NONE',  ( -6.906132195718435618, -3.984195806739584178, 1.626303258728256651E-16 ) ) ;
#36080=CARTESIAN_POINT ( 'NONE',  ( -1.250000000000000222, 0.000000000000000000, -10.00000000000000000 ) ) ;
#36086=CARTESIAN_POINT ( 'NONE',  ( 16.76006782980217125, -2.050259795448531541, 9.178419661560148768 ) ) ;
#36094=ORIENTED_EDGE ( 'NONE', *, *, #130, .F. ) ;
#36096=CARTESIAN_POINT ( 'NONE',  ( 50.11058929355270664, -7.578863168071591438, 7.455576670931136185 ) ) ;
#36099=B_SPLINE_CURVE_WITH_KNOTS ( 'NONE', 3,
 ( #11790, #12793, #8201, #8711 ),
 .UNSPECIFIED., .F., .F.,
 ( 4, 4 ),
 ( 0.9688112071879413367, 0.9724175925769212858 ),
 .UNSPECIFIED. ) ;
#36101=B_SPLINE_CURVE_WITH_KNOTS ( 'NONE', 3,
 ( #8248, #4394, #22873, #34441 ),
 .UNSPECIFIED., .F., .F.,
 ( 4, 4 ),
 ( 3.127317220692750759E-18, 0.002458791966311098948 ),
 .UNSPECIFIED. ) ;
#36111=CARTESIAN_POINT ( 'NONE',  ( -4.531159320492035292, -41.49457383023836599, -8.080361901872242569 ) ) ;
#36113=LINE ( 'NONE', #40954, #19099 ) ;
#36133=CARTESIAN_POINT ( 'NONE',  ( 5.320787806771834383, -8.466948512617054945, 0.000000000000000000 ) ) ;
#36137=CARTESIAN_POINT ( 'NONE',  ( 1.011271242968694084, -0.7347315653655782652, 3.333333333333333481 ) ) ;
#36138=CARTESIAN_POINT ( 'NONE',  ( -1.275949648750062559, 0.1226307170720055406, 9.967237415621763574 ) ) ;
#36147=DIRECTION ( 'NONE',  ( -0.8090169943749507819, 0.5877852522924685852, 0.000000000000000000 ) ) ;
#36149=CARTESIAN_POINT ( 'NONE',  ( 36.97942854200454832, -6.226705766838405154, 8.914903342594563185 ) ) ;
#36157=CARTESIAN_POINT ( 'NONE',  ( -0.8995557290265571160, -5.891360144184186076, -3.659182332138577465E-16 ) ) ;
#36158=CARTESIAN_POINT ( 'NONE',  ( -14.29087950072019098, -9.652079258044555132, 8.727788335465566760 ) ) ;
#36166=CARTESIAN_POINT ( 'NONE',  ( -1.111507796622772881, -1.112188257001367697, 9.945241992664895392 ) ) ;
#36167=EDGE_CURVE ( 'NONE', #20022, #41021, #5168, .T. ) ;
#36184=DIRECTION ( 'NONE',  ( -0.2599384441937559465, -0.8000082703740970524, 0.5407575913134972101 ) ) ;
#36188=B_SPLINE_CURVE_WITH_KNOTS ( 'NONE', 3,
 ( #22753, #38422, #3238, #18886 ),
 .UNSPECIFIED., .F., .F.,
 ( 4, 4 ),
 ( 0.003717756508417797024, 0.009855839453069397890 ),
 .UNSPECIFIED. ) ;
#36193=CARTESIAN_POINT ( 'NONE',  ( -4.641001526964560142, -33.28196331604080171, -8.016098858316199838 ) ) ;
#36201=CARTESIAN_POINT ( 'NONE',  ( -50.11058929355266400, 7.578863168071933387, 7.455576670931136185 ) ) ;
#36202=CARTESIAN_POINT ( 'NONE',  ( -0.3370904143228943828, -0.2449105217885308716, 10.00000000000000000 ) ) ;
#36205=ADVANCED_FACE ( 'NONE', ( #4551 ), #7642, .T. ) ;
#36209=DIRECTION ( 'NONE',  ( 0.000000000000000000, 0.000000000000000000, 1.000000000000000000 ) ) ;
#36218=CARTESIAN_POINT ( 'NONE',  ( -10.70590866674912967, 12.76446523155714985, -3.546734833711462365 ) ) ;
#36232=ORIENTED_EDGE ( 'NONE', *, *, #29577, .T. ) ;
#36237=CARTESIAN_POINT ( 'NONE',  ( -1.011271242968693862, 0.7347315653655780432, 3.333333333333333481 ) ) ;
#36253=ADVANCED_FACE ( 'NONE', ( #41965 ), #50606, .T. ) ;
#36257=DIRECTION ( 'NONE',  ( -1.000000000000000000, 0.000000000000000000, 0.000000000000000000 ) ) ;
#36259=FACE_OUTER_BOUND ( 'NONE', #18280, .T. ) ;
#36264=B_SPLINE_SURFACE_WITH_KNOTS ( 'NONE', 3, 3, ( 
 ( #5039, #1467, #1215, #16860 ),
 ( #32524, #48104, #32759, #48357 ),
 ( #7321, #26321, #2702, #26063 ),
 ( #34529, #22957, #50110, #6811 ) ),
 .UNSPECIFIED., .F., .F., .F.,
 ( 4, 4 ),
 ( 4, 4 ),
 ( 0.000000000000000000, 1.000000000000000000 ),
 ( 0.000000000000000000, 1.000000000000000000 ),
 .UNSPECIFIED. ) ;
#36283=CARTESIAN_POINT ( 'NONE',  ( -30.12518629743573584, -14.70074613238887551, 1.847720168420772691 ) ) ;
#36286=FACE_OUTER_BOUND ( 'NONE', #26296, .T. ) ;
#36289=CARTESIAN_POINT ( 'NONE',  ( 31.44259251615245176, 38.95901822126168668, -9.367992836599951190 ) ) ;
#36290=CARTESIAN_POINT ( 'NONE',  ( -1.086995624458622967, 37.52050741145076529, -3.721387749823088953 ) ) ;
#36292=CARTESIAN_POINT ( 'NONE',  ( -2.538055338523177440, -33.28424297489108596, -9.367992836599954742 ) ) ;
#36293=EDGE_LOOP ( 'NONE', ( #32362, #31675, #21003 ) ) ;
#36298=VERTEX_POINT ( 'NONE', #42967 ) ;
#36299=EDGE_CURVE ( 'NONE', #23256, #40728, #33365, .T. ) ;
#36303=CARTESIAN_POINT ( 'NONE',  ( -3.345242017215803276, 2.159124855890678596, -2.642742795433417058E-16 ) ) ;
#36306=ORIENTED_EDGE ( 'NONE', *, *, #14634, .F. ) ;
#36310=CARTESIAN_POINT ( 'NONE',  ( -0.3862712429686729343, -1.188820645368946050, 10.00000000000000000 ) ) ;
#36315=CARTESIAN_POINT ( 'NONE',  ( 3.975459390375365665, 0.2195152216756870167, 1.992221491942114397E-15 ) ) ;
#36317=ORIENTED_EDGE ( 'NONE', *, *, #33357, .F. ) ;
#36321=CARTESIAN_POINT ( 'NONE',  ( 0.3862712429686978033, -1.188820645368937834, 10.00000000000000000 ) ) ;
#36324=ORIENTED_EDGE ( 'NONE', *, *, #46763, .T. ) ;
#36331=CARTESIAN_POINT ( 'NONE',  ( -15.80799809827351154, 29.65358618225718956, -8.016098858316199838 ) ) ;
#36332=ORIENTED_EDGE ( 'NONE', *, *, #43212, .F. ) ;
#36334=CARTESIAN_POINT ( 'NONE',  ( -1.250000000000000222, 0.000000000000000000, 10.00000000000000000 ) ) ;
#36335=CARTESIAN_POINT ( 'NONE',  ( 15.00099850811936264, 7.462898891544210933, 9.403735324607438884 ) ) ;
#36349=CARTESIAN_POINT ( 'NONE',  ( -30.87089393895367095, 12.69923079256638587, -9.367992836599954742 ) ) ;
#36350=B_SPLINE_CURVE_WITH_KNOTS ( 'NONE', 3,
 ( #9142, #48096, #36111, #24801 ),
 .UNSPECIFIED., .F., .F.,
 ( 4, 4 ),
 ( 0.000000000000000000, 0.2545280377015988749 ),
 .UNSPECIFIED. ) ;
#36357=CARTESIAN_POINT ( 'NONE',  ( -0.8589491062558242129, -0.9799133293386017574, 9.961922210043272941 ) ) ;
#36362=CARTESIAN_POINT ( 'NONE',  ( 17.34922095635755568, 33.24536858281893359, 8.914903342594564961 ) ) ;
#36367=CARTESIAN_POINT ( 'NONE',  ( 12.35406723005396046, -11.51001571518080624, 9.178419661560148768 ) ) ;
#36371=B_SPLINE_SURFACE_WITH_KNOTS ( 'NONE', 3, 3, ( 
 ( #38807, #15691, #6984, #11601 ),
 ( #18770, #11086, #42876, #23398 ),
 ( #38048, #30335, #39066, #30592 ),
 ( #22633, #19021, #3373, #3889 ) ),
 .UNSPECIFIED., .F., .F., .F.,
 ( 4, 4 ),
 ( 4, 4 ),
 ( 0.000000000000000000, 1.000000000000000000 ),
 ( 0.000000000000000000, 1.000000000000000000 ),
 .UNSPECIFIED. ) ;
#36375=ADVANCED_FACE ( 'NONE', ( #50114 ), #43281, .T. ) ;
#36380=CARTESIAN_POINT ( 'NONE',  ( -1.365263087672800246, 0.5437404457009007430, 9.958264684458713489 ) ) ;
#36390=VERTEX_POINT ( 'NONE', #36582 ) ;
#36392=CARTESIAN_POINT ( 'NONE',  ( 22.69295089195473736, 45.31600496604706052, 7.455576670931136185 ) ) ;
#36396=VERTEX_POINT ( 'NONE', #8601 ) ;
#36402=EDGE_CURVE ( 'NONE', #6007, #41927, #10083, .T. ) ;
#36422=CARTESIAN_POINT ( 'NONE',  ( -9.999999999999921840, -0.04964634317306688277, 9.296265711052123848 ) ) ;
#36434=VERTEX_POINT ( 'NONE', #20135 ) ;
#36439=CARTESIAN_POINT ( 'NONE',  ( -23.82716369509181575, -44.49195112875988656, 8.356839323120299312 ) ) ;
#36445=FACE_OUTER_BOUND ( 'NONE', #45136, .T. ) ;
#36449=EDGE_LOOP ( 'NONE', ( #44091, #26531, #43494, #36796, #24212, #33427, #39160, #8480, #49293, #40288, #23151, #42073 ) ) ;
#36461=CARTESIAN_POINT ( 'NONE',  ( 15.73090589902275482, 29.60029367929053024, 1.847720168420772691 ) ) ;
#36502=CARTESIAN_POINT ( 'NONE',  ( 36.08557433729230013, -35.58569447144767395, 7.455576670931136185 ) ) ;
#36505=CARTESIAN_POINT ( 'NONE',  ( 47.22310614333766665, 16.46562252335956344, -3.760136334089591248 ) ) ;
#36508=ORIENTED_EDGE ( 'NONE', *, *, #43212, .T. ) ;
#36519=CARTESIAN_POINT ( 'NONE',  ( -33.43156050989129824, 4.370686678976795747, 8.807470649214879543 ) ) ;
#36524=VERTEX_POINT ( 'NONE', #12434 ) ;
#36529=CARTESIAN_POINT ( 'NONE',  ( 0.000000000000000000, 50.00000000000000000, 0.000000000000000000 ) ) ;
#36535=ADVANCED_FACE ( 'NONE', ( #15156 ), #46421, .F. ) ;
#36539=CARTESIAN_POINT ( 'NONE',  ( 0.4166666666666669072, 0.000000000000000000, 10.00000000000000000 ) ) ;
#36543=AXIS2_PLACEMENT_3D ( 'NONE', #9871, #44496, #6016 ) ;
#36552=CARTESIAN_POINT ( 'NONE',  ( -15.57957361750255565, -5.755602074545403291, 3.266473740018926541 ) ) ;
#36569=CARTESIAN_POINT ( 'NONE',  ( 27.31081730472575941, 41.96092862852144378, 3.199614146704519602 ) ) ;
#36572=ADVANCED_FACE ( 'NONE', ( #32971 ), #5744, .F. ) ;
#36577=ORIENTED_EDGE ( 'NONE', *, *, #11245, .T. ) ;
#36578=CARTESIAN_POINT ( 'NONE',  ( -4.641001526964561918, -33.28196331604080171, -8.016098858316205167 ) ) ;
#36579=CARTESIAN_POINT ( 'NONE',  ( 46.11867747200574996, -19.86470446310233484, -8.016098858316199838 ) ) ;
#36580=ORIENTED_EDGE ( 'NONE', *, *, #5031, .T. ) ;
#36582=CARTESIAN_POINT ( 'NONE',  ( -1.080000014127418639, -0.7606467978654640749, 9.943883492372872723 ) ) ;
#36584=FACE_OUTER_BOUND ( 'NONE', #37060, .T. ) ;
#36598=CARTESIAN_POINT ( 'NONE',  ( -7.359817328027146388, -15.16751262232800102, 2.590526750877053086 ) ) ;
#36602=CARTESIAN_POINT ( 'NONE',  ( 33.43156050989131955, -4.370686678976570150, 8.807470649214879543 ) ) ;
#36609=AXIS2_PLACEMENT_3D ( 'NONE', #30307, #34677, #26451 ) ;
#36614=CARTESIAN_POINT ( 'NONE',  ( -33.01266944765060174, 5.813986777101691317, 1.847720168420772691 ) ) ;
#36616=CARTESIAN_POINT ( 'NONE',  ( -3.695802964311593719, -9.324875653452746604, 9.390253821402618328 ) ) ;
#36624=B_SPLINE_CURVE_WITH_KNOTS ( 'NONE', 3,
 ( #36133, #977, #4060, #12260 ),
 .UNSPECIFIED., .F., .F.,
 ( 4, 4 ),
 ( 0.001924139378288104675, 0.008062652406780950951 ),
 .UNSPECIFIED. ) ;
#36629=EDGE_CURVE ( 'NONE', #3137, #38752, #9982, .T. ) ;
#36634=CARTESIAN_POINT ( 'NONE',  ( 13.59579750444771307, -10.60877755095900632, 8.727788335465566760 ) ) ;
#36652=ORIENTED_EDGE ( 'NONE', *, *, #40589, .T. ) ;
#36653=CARTESIAN_POINT ( 'NONE',  ( 0.6108107228405675881, -1.056024183042613140, 9.963925895596188909 ) ) ;
#36672=CARTESIAN_POINT ( 'NONE',  ( -1.011271242968677875, -0.7347315653656004697, -10.00000000000000000 ) ) ;
#36678=AXIS2_PLACEMENT_3D ( 'NONE', #21539, #45862, #18692 ) ;
#36683=CARTESIAN_POINT ( 'NONE',  ( -1.055760676366898521, -37.52140099356444836, -2.490396854064190535 ) ) ;
#36692=CARTESIAN_POINT ( 'NONE',  ( -0.3370904143228963812, 0.2449105217885287067, -10.00000000000000000 ) ) ;
#36698=B_SPLINE_SURFACE_WITH_KNOTS ( 'NONE', 3, 3, ( 
 ( #3715, #14754, #18590, #50103 ),
 ( #50619, #18838, #34522, #26561 ),
 ( #6803, #15012, #46018, #22952 ),
 ( #19366, #10649, #3189, #49843 ) ),
 .UNSPECIFIED., .F., .F., .F.,
 ( 4, 4 ),
 ( 4, 4 ),
 ( 0.000000000000000000, 1.000000000000000000 ),
 ( 0.000000000000000000, 1.000000000000000000 ),
 .UNSPECIFIED. ) ;
#36702=EDGE_CURVE ( 'NONE', #21514, #44231, #25898, .T. ) ;
#36712=CARTESIAN_POINT ( 'NONE',  ( 0.6909887759939999929, -1.008432015058921438, 9.987567862361069970 ) ) ;
#36716=AXIS2_PLACEMENT_3D ( 'NONE', #17575, #45744, #49081 ) ;
#36725=CARTESIAN_POINT ( 'NONE',  ( -34.95136153415531766, 36.40974830873496870, 8.356839323120299312 ) ) ;
#36740=CARTESIAN_POINT ( 'NONE',  ( 0.1287570809895630941, -0.3962735484563133515, 10.00000000000000000 ) ) ;
#36747=CARTESIAN_POINT ( 'NONE',  ( -27.33593271309441519, 41.94268121623345280, -9.367992836599951190 ) ) ;
#36750=CARTESIAN_POINT ( 'NONE',  ( 35.51846793572394034, -35.99772139009119343, 7.906207997025717304 ) ) ;
#36753=CARTESIAN_POINT ( 'NONE',  ( -8.470991794550055687, -5.371644396275288003, 9.390253821402620105 ) ) ;
#36758=CARTESIAN_POINT ( 'NONE',  ( 0.7601424845489945792, -1.297311920616997627, 9.927319414211225990 ) ) ;
#36759=CARTESIAN_POINT ( 'NONE',  ( 34.08355720199905647, -2.371364769369109116, 7.455576670931136185 ) ) ;
#36773=CARTESIAN_POINT ( 'NONE',  ( 1.249999999999999778, 0.000000000000000000, 10.00000000000000000 ) ) ;
#36782=CARTESIAN_POINT ( 'NONE',  ( 32.36066692128250821, -7.813306791042813337, 3.199614146704519602 ) ) ;
#36783=CARTESIAN_POINT ( 'NONE',  ( -6.208157169185024138, 36.98937201184289592, 8.506357886886741326 ) ) ;
#36784=CARTESIAN_POINT ( 'NONE',  ( 9.483938762529211530, -3.217310375392752331, 3.215106848023439934 ) ) ;
#36796=ORIENTED_EDGE ( 'NONE', *, *, #15794, .F. ) ;
#36798=B_SPLINE_SURFACE_WITH_KNOTS ( 'NONE', 3, 3, ( 
 ( #33509, #25804, #71, #39081 ),
 ( #19541, #41448, #7772, #22450 ),
 ( #30153, #6552, #41703, #22206 ),
 ( #10405, #3901, #38122, #35225 ) ),
 .UNSPECIFIED., .F., .F., .F.,
 ( 4, 4 ),
 ( 4, 4 ),
 ( 0.000000000000000000, 1.000000000000000000 ),
 ( 0.000000000000000000, 1.000000000000000000 ),
 .UNSPECIFIED. ) ;
#36807=CARTESIAN_POINT ( 'NONE',  ( 1.228394325311184421, -1.341866297401743235, 9.903764339332088440 ) ) ;
#36813=CARTESIAN_POINT ( 'NONE',  ( 0.3862712429686810944, 1.188820645368943607, 10.00000000000000000 ) ) ;
#36824=CARTESIAN_POINT ( 'NONE',  ( -0.3862712429686977478, 1.188820645368937390, 10.00000000000000000 ) ) ;
#36832=CARTESIAN_POINT ( 'NONE',  ( -1.637465050678293954, -0.1702693745679247084, 9.936700280135957186 ) ) ;
#36842=B_SPLINE_CURVE_WITH_KNOTS ( 'NONE', 3,
 ( #29398, #49358, #14244, #26060 ),
 .UNSPECIFIED., .F., .F.,
 ( 4, 4 ),
 ( 1.734723475976807094E-18, 0.002458791966311101550 ),
 .UNSPECIFIED. ) ;
#36850=CARTESIAN_POINT ( 'NONE',  ( 49.67735855322978011, -8.912210285361751971, 8.356839323120299312 ) ) ;
#36851=CARTESIAN_POINT ( 'NONE',  ( 0.3862712429686810944, 1.188820645368943607, -10.00000000000000000 ) ) ;
#36866=AXIS2_PLACEMENT_3D ( 'NONE', #31302, #31557, #31042 ) ;
#36873=CARTESIAN_POINT ( 'NONE',  ( 6.875132362119187768, -50.00000000000000711, 8.356839323120299312 ) ) ;
#36876=CARTESIAN_POINT ( 'NONE',  ( 22.69295089195473025, 45.31600496604705341, 7.455576670931136185 ) ) ;
#36885=ORIENTED_EDGE ( 'NONE', *, *, #35989, .F. ) ;
#36893=B_SPLINE_CURVE_WITH_KNOTS ( 'NONE', 3,
 ( #1259, #48146, #36157, #32813 ),
 .UNSPECIFIED., .F., .F.,
 ( 4, 4 ),
 ( 0.0001426870652665898870, 0.006281196370944869614 ),
 .UNSPECIFIED. ) ;
#36899=VECTOR ( 'NONE', #15665, 1000.000000000000114 ) ;
#36910=VERTEX_POINT ( 'NONE', #33345 ) ;
#36912=CARTESIAN_POINT ( 'NONE',  ( 1.011271242968694084, -0.7347315653655782652, 10.00000000000000000 ) ) ;
#36914=ORIENTED_EDGE ( 'NONE', *, *, #39314, .F. ) ;
#36926=CARTESIAN_POINT ( 'NONE',  ( 16.15814872688565984, 4.048305257546810587, -2.870787844569587133 ) ) ;
#36929=EDGE_CURVE ( 'NONE', #22371, #22111, #41532, .T. ) ;
#36930=CARTESIAN_POINT ( 'NONE',  ( -1.011271242968683426, -0.7347315653655928092, 3.333333333333333481 ) ) ;
#36938=CARTESIAN_POINT ( 'NONE',  ( -4.339432828817248122, -37.24807810779213213, -8.192531242611266862 ) ) ;
#36945=CARTESIAN_POINT ( 'NONE',  ( -11.54386348672375107, -12.18274641659808211, -9.233365092205394475 ) ) ;
#36948=VERTEX_POINT ( 'NONE', #30488 ) ;
#36955=CARTESIAN_POINT ( 'NONE',  ( -22.69295089195507487, -45.31600496604688999, 7.455576670931136185 ) ) ;
#36957=CARTESIAN_POINT ( 'NONE',  ( -0.1287570809895658697, 0.3962735484563123523, 10.00000000000000000 ) ) ;
#36961=VERTEX_POINT ( 'NONE', #10988 ) ;
#36976=CARTESIAN_POINT ( 'NONE',  ( 1.275994128725544741, -0.1230186051320594776, 9.948547179989619238 ) ) ;
#36983=CARTESIAN_POINT ( 'NONE',  ( 0.3862712429686894766, -1.188820645368940276, 10.00000000000000000 ) ) ;
#36992=CARTESIAN_POINT ( 'NONE',  ( -23.29043492822808759, 24.10797434788186067, 1.847720168420772691 ) ) ;
#37004=CARTESIAN_POINT ( 'NONE',  ( 0.2773062244624638351, -1.251557370488896481, 9.948547179989619238 ) ) ;
#37005=ORIENTED_EDGE ( 'NONE', *, *, #3586, .F. ) ;
#37022=CARTESIAN_POINT ( 'NONE',  ( 6.646097924774390542, -4.355953743237533260, 9.432811472610147518 ) ) ;
#37023=ADVANCED_FACE ( 'NONE', ( #2528 ), #28569, .T. ) ;
#37032=CARTESIAN_POINT ( 'NONE',  ( 1.249999999999999778, 0.000000000000000000, 9.972675548442463622 ) ) ;
#37033=B_SPLINE_CURVE_WITH_KNOTS ( 'NONE', 3,
 ( #30757, #37704, #46366, #2533 ),
 .UNSPECIFIED., .F., .F.,
 ( 4, 4 ),
 ( 1.409296014025916843E-17, 0.009404495247862340590 ),
 .UNSPECIFIED. ) ;
#37041=CARTESIAN_POINT ( 'NONE',  ( 0.6440276692615888310, 16.64212148744554298, -9.683996418299976483 ) ) ;
#37054=PLANE ( 'NONE',  #23928 ) ;
#37057=CARTESIAN_POINT ( 'NONE',  ( 50.11058929355270664, -7.578863168071591438, 7.455576670931136185 ) ) ;
#37060=EDGE_LOOP ( 'NONE', ( #2316, #26428, #17116 ) ) ;
#37069=CARTESIAN_POINT ( 'NONE',  ( 7.749480817862238524, 14.85497772329518895, 9.403735324607438884 ) ) ;
#37070=DIRECTION ( 'NONE',  ( -0.2599384441937671042, 0.8000082703740934997, 0.5407575913134970991 ) ) ;
#37077=ORIENTED_EDGE ( 'NONE', *, *, #4482, .F. ) ;
#37083=VERTEX_POINT ( 'NONE', #12654 ) ;
#37084=EDGE_LOOP ( 'NONE', ( #21698, #11407, #37155 ) ) ;
#37089=ORIENTED_EDGE ( 'NONE', *, *, #18398, .T. ) ;
#37090=( GEOMETRIC_REPRESENTATION_CONTEXT ( 3 ) GLOBAL_UNCERTAINTY_ASSIGNED_CONTEXT ( ( #37392 ) ) GLOBAL_UNIT_ASSIGNED_CONTEXT ( ( #15317, #42242, #46557 ) ) REPRESENTATION_CONTEXT ( 'NONE', 'WORKASPACE' ) );
#37103=CARTESIAN_POINT ( 'NONE',  ( 50.11058929355269953, -7.578863168071589662, 7.455576670931136185 ) ) ;
#37107=ORIENTED_EDGE ( 'NONE', *, *, #30281, .F. ) ;
#37110=FACE_OUTER_BOUND ( 'NONE', #49802, .T. ) ;
#37111=DIRECTION ( 'NONE',  ( 0.8411784753765545464, 0.000000000000000000, 0.5407575913134972101 ) ) ;
#37112=CARTESIAN_POINT ( 'NONE',  ( -36.80807479611529942, 7.357694319819784390, 1.982731392810406668 ) ) ;
#37123=CARTESIAN_POINT ( 'NONE',  ( -7.129058724845069861, -15.30620660340479766, 9.178419661560148768 ) ) ;
#37126=CARTESIAN_POINT ( 'NONE',  ( 1.401228687704787257, -0.7134216605332859285, 9.945241992664895392 ) ) ;
#37136=CARTESIAN_POINT ( 'NONE',  ( -2.735100745861921201, 5.294958516888076616, 6.606856988583542645E-16 ) ) ;
#37138=EDGE_CURVE ( 'NONE', #31922, #31313, #28348, .T. ) ;
#37140=CARTESIAN_POINT ( 'NONE',  ( 8.277096487746778308, -33.14818118907697198, 7.455576670931136185 ) ) ;
#37144=ADVANCED_FACE ( 'NONE', ( #28317 ), #3097, .T. ) ;
#37148=CARTESIAN_POINT ( 'NONE',  ( -1.011271242968693862, 0.7347315653655780432, 10.00000000000000000 ) ) ;
#37154=ORIENTED_EDGE ( 'NONE', *, *, #42405, .T. ) ;
#37155=ORIENTED_EDGE ( 'NONE', *, *, #42341, .F. ) ;
#37176=CARTESIAN_POINT ( 'NONE',  ( 0.3862712429686727678, 1.188820645368945605, 3.333333333333333481 ) ) ;
#37178=CARTESIAN_POINT ( 'NONE',  ( -8.843309649387274263, 14.11631751497152720, -2.870787844569587133 ) ) ;
#37182=B_SPLINE_CURVE_WITH_KNOTS ( 'NONE', 3,
 ( #20497, #48157, #36166, #1012 ),
 .UNSPECIFIED., .F., .F.,
 ( 4, 4 ),
 ( 0.9811748202683102660, 0.9878904167554125593 ),
 .UNSPECIFIED. ) ;
#37197=CARTESIAN_POINT ( 'NONE',  ( -7.216980890441389462, 6.922079660550276792, 0.000000000000000000 ) ) ;
#37208=AXIS2_PLACEMENT_3D ( 'NONE', #6097, #17644, #32810 ) ;
#37224=B_SPLINE_SURFACE_WITH_KNOTS ( 'NONE', 3, 3, ( 
 ( #22295, #14083, #37973, #26397 ),
 ( #25909, #23826, #15613, #7669 ),
 ( #12026, #22798, #7422, #11264 ),
 ( #43051, #38480, #3291, #30767 ) ),
 .UNSPECIFIED., .F., .F., .F.,
 ( 4, 4 ),
 ( 4, 4 ),
 ( 0.000000000000000000, 1.000000000000000000 ),
 ( 0.000000000000000000, 1.000000000000000000 ),
 .UNSPECIFIED. ) ;
#37238=CARTESIAN_POINT ( 'NONE',  ( 8.843309649387377291, -14.11631751497145792, -2.870787844569587133 ) ) ;
#37241=CARTESIAN_POINT ( 'NONE',  ( -45.21167770612412085, -22.65616271077779942, 7.906207997025717304 ) ) ;
#37242=CARTESIAN_POINT ( 'NONE',  ( -32.36066692128246558, 7.813306791043033606, 3.199614146704519602 ) ) ;
#37255=CARTESIAN_POINT ( 'NONE',  ( -7.576114424932982594, 33.14742743729794938, 7.906207997025717304 ) ) ;
#37274=ORIENTED_EDGE ( 'NONE', *, *, #49465, .T. ) ;
#37281=CARTESIAN_POINT ( 'NONE',  ( -1.769963848780949478, 9.842115015280430868, 0.000000000000000000 ) ) ;
#37287=CARTESIAN_POINT ( 'NONE',  ( 3.996390545799824334, -16.57371371864897469, 8.953103998512858652 ) ) ;
#37292=ORIENTED_EDGE ( 'NONE', *, *, #2087, .T. ) ;
#37300=VERTEX_POINT ( 'NONE', #26233 ) ;
#37319=CARTESIAN_POINT ( 'NONE',  ( -9.281355226777547429, 3.722424633806451943, 0.000000000000000000 ) ) ;
#37320=CARTESIAN_POINT ( 'NONE',  ( 0.8603719846014596939, -1.073163306097343783, 9.972175347158279024 ) ) ;
#37321=CARTESIAN_POINT ( 'NONE',  ( 26.20171990995799760, -42.76673505352026439, -8.466730184410787174 ) ) ;
#37325=CARTESIAN_POINT ( 'NONE',  ( 7.129058724844953510, 15.30620660340485095, 9.178419661560148768 ) ) ;
#37328=CARTESIAN_POINT ( 'NONE',  ( 17.23491422248386584, -0.5912720620000816441, 8.727788335465566760 ) ) ;
#37329=ORIENTED_EDGE ( 'NONE', *, *, #16412, .T. ) ;
#37331=CARTESIAN_POINT ( 'NONE',  ( -0.8738110990267208278, -1.684976543153730244, 9.900811091504552408 ) ) ;
#37332=CARTESIAN_POINT ( 'NONE',  ( 31.28234235046230793, 11.28615439405779064, -3.760136334089591248 ) ) ;
#37353=EDGE_LOOP ( 'NONE', ( #13757, #12494, #28960, #10518 ) ) ;
#37360=CARTESIAN_POINT ( 'NONE',  ( -3.888415560953798700, -9.227494953140025657, 3.092310436554650543 ) ) ;
#37361=CARTESIAN_POINT ( 'NONE',  ( -15.62858259096117841, 5.755205073598719245, -9.683996418299976483 ) ) ;
#37372=VECTOR ( 'NONE', #12364, 999.9999999999998863 ) ;
#37375=CARTESIAN_POINT ( 'NONE',  ( 1.448406091252584238, -0.9360325558322883932, 9.928159647716132241 ) ) ;
#37376=CARTESIAN_POINT ( 'NONE',  ( -1.448406091252275818, 0.9360325558308429938, 9.928159647716187308 ) ) ;
#37377=VECTOR ( 'NONE', #5529, 1000.000000000000000 ) ;
#37383=B_SPLINE_CURVE_WITH_KNOTS ( 'NONE', 3,
 ( #32606, #30017, #14348, #25401 ),
 .UNSPECIFIED., .F., .F.,
 ( 4, 4 ),
 ( 0.7998230999345287140, 0.9869080488566185361 ),
 .UNSPECIFIED. ) ;
#37385=CARTESIAN_POINT ( 'NONE',  ( -1.553324196727134954, 1.431239106454489152, 9.890170120223999106 ) ) ;
#37392=UNCERTAINTY_MEASURE_WITH_UNIT (LENGTH_MEASURE( 1.000000000000000082E-05 ), #15317, 'distance_accuracy_value', 'NONE');
#37396=EDGE_LOOP ( 'NONE', ( #9219, #44478, #44290, #15861 ) ) ;
#37400=CARTESIAN_POINT ( 'NONE',  ( 49.89397392339123627, -8.245536726716670373, 7.906207997025717304 ) ) ;
#37401=CARTESIAN_POINT ( 'NONE',  ( -16.71930270649968620, -33.57409379679878469, 8.506357886886739550 ) ) ;
#37405=CARTESIAN_POINT ( 'NONE',  ( 13.92102703536701114, 30.85732372859822803, 8.356839323120299312 ) ) ;
#37415=CARTESIAN_POINT ( 'NONE',  ( 2.052570692346796122, -0.2041439924650269022, 9.889206917020301191 ) ) ;
#37428=CARTESIAN_POINT ( 'NONE',  ( -37.19569680397831490, 4.820783179364701354, 8.100132398494512387 ) ) ;
#37436=CARTESIAN_POINT ( 'NONE',  ( 1.424123654779712922, 0.3625862473308184009, 9.958264684458541183 ) ) ;
#37446=ADVANCED_FACE ( 'NONE', ( #7236 ), #28985, .T. ) ;
#37457=CIRCLE ( 'NONE', #23528, 10.00000000000000000 ) ;
#37469=CARTESIAN_POINT ( 'NONE',  ( 36.08557433729230013, -35.58569447144767395, 7.455576670931136185 ) ) ;
#37472=CARTESIAN_POINT ( 'NONE',  ( 2.945500763482279627, 16.64098165802040086, -9.008049429158100807 ) ) ;
#37479=CARTESIAN_POINT ( 'NONE',  ( 0.3862712429686894766, -1.188820645368940276, -10.00000000000000000 ) ) ;
#37486=CARTESIAN_POINT ( 'NONE',  ( -2.089000987151039102, -7.666878472664052424, 9.432811472610138637 ) ) ;
#37499=DIRECTION ( 'NONE',  ( -0.000000000000000000, -0.000000000000000000, -1.000000000000000000 ) ) ;
#37508=EDGE_CURVE ( 'NONE', #37300, #13105, #22789, .T. ) ;
#37510=EDGE_CURVE ( 'NONE', #339, #47355, #49000, .T. ) ;
#37517=VERTEX_POINT ( 'NONE', #312 ) ;
#37520=CARTESIAN_POINT ( 'NONE',  ( 0.05286079371170563507, -1.230216489825521009, 9.975326647350893694 ) ) ;
#37524=ADVANCED_FACE ( 'NONE', ( #48948 ), #33515, .T. ) ;
#37526=B_SPLINE_SURFACE_WITH_KNOTS ( 'NONE', 3, 3, ( 
 ( #49998, #38278, #18228, #5931 ),
 ( #14901, #26444, #2336, #48981 ),
 ( #49241, #38014, #34171, #37766 ),
 ( #45410, #14644, #45913, #10792 ) ),
 .UNSPECIFIED., .F., .F., .F.,
 ( 4, 4 ),
 ( 4, 4 ),
 ( 0.000000000000000000, 1.000000000000000000 ),
 ( 0.000000000000000000, 1.000000000000000000 ),
 .UNSPECIFIED. ) ;
#37528=CARTESIAN_POINT ( 'NONE',  ( 1.212058190970869198, 0.1697289529807369801, 9.966990782790126957 ) ) ;
#37530=CARTESIAN_POINT ( 'NONE',  ( 8.277096487746778308, -50.00000000000000000, 7.455576670931136185 ) ) ;
#37552=ORIENTED_EDGE ( 'NONE', *, *, #4482, .T. ) ;
#37556=CARTESIAN_POINT ( 'NONE',  ( -1.460157059060481544, 1.483633425177112164, 9.888808121373916293 ) ) ;
#37569=CARTESIAN_POINT ( 'NONE',  ( 1.011271242968694084, -0.7347315653655782652, 10.00000000000000000 ) ) ;
#37570=EDGE_LOOP ( 'NONE', ( #36306, #29537, #14203, #45284 ) ) ;
#37576=DIRECTION ( 'NONE',  ( 0.000000000000000000, 0.000000000000000000, -1.000000000000000000 ) ) ;
#37585=CARTESIAN_POINT ( 'NONE',  ( 2.536646476037169418, 2.794100479408543780, 9.865049507598756762 ) ) ;
#37617=EDGE_CURVE ( 'NONE', #1912, #12326, #6268, .T. ) ;
#37622=CARTESIAN_POINT ( 'NONE',  ( 0.3862712429686978033, -1.188820645368937834, 3.333333333333333481 ) ) ;
#37626=CARTESIAN_POINT ( 'NONE',  ( -46.75893035013464072, -17.89420872045582200, 3.199614146704519602 ) ) ;
#37627=CARTESIAN_POINT ( 'NONE',  ( -6.508636631827791064, -15.75743548351446854, 8.953103998512858652 ) ) ;
#37640=EDGE_LOOP ( 'NONE', ( #35021, #35849, #45011, #48653 ) ) ;
#37654=CARTESIAN_POINT ( 'NONE',  ( -47.88254548617756967, 14.43607691413558669, -3.760136334089591248 ) ) ;
#37657=CARTESIAN_POINT ( 'NONE',  ( -33.57695195286787282, -16.69845195084869616, 8.914903342594564961 ) ) ;
#37662=FACE_OUTER_BOUND ( 'NONE', #5045, .T. ) ;
#37664=CARTESIAN_POINT ( 'NONE',  ( 24.39427009665985224, 44.07992421011656603, 8.807470649214879543 ) ) ;
#37667=B_SPLINE_CURVE_WITH_KNOTS ( 'NONE', 3,
 ( #23277, #15848, #39716, #50697 ),
 .UNSPECIFIED., .F., .F.,
 ( 4, 4 ),
 ( 0.000000000000000000, 0.2562577668812813791 ),
 .UNSPECIFIED. ) ;
#37668=CARTESIAN_POINT ( 'NONE',  ( 0.3862712429686727678, 1.188820645368945605, 10.00000000000000000 ) ) ;
#37687=VERTEX_POINT ( 'NONE', #2555 ) ;
#37703=B_SPLINE_CURVE_WITH_KNOTS ( 'NONE', 3,
 ( #39975, #47356, #12496, #28661 ),
 .UNSPECIFIED., .F., .F.,
 ( 4, 4 ),
 ( 0.0002936521407534369954, 0.0006663369986142379710 ),
 .UNSPECIFIED. ) ;
#37704=CARTESIAN_POINT ( 'NONE',  ( -8.294258456918070621, -5.607426633512162084, 6.185594734181537824 ) ) ;
#37715=CARTESIAN_POINT ( 'NONE',  ( -2.569099690548740877, 50.00000000000000711, 3.199614146704519602 ) ) ;
#37743=CARTESIAN_POINT ( 'NONE',  ( 3.566525152641073504, -1.569997364302916809, 9.741991644047246268 ) ) ;
#37755=CARTESIAN_POINT ( 'NONE',  ( -25.08868538179562435, 27.91927157928049752, 6.057468652304069501 ) ) ;
#37756=ORIENTED_EDGE ( 'NONE', *, *, #36929, .T. ) ;
#37759=CARTESIAN_POINT ( 'NONE',  ( -36.08557433729205144, 35.58569447144795816, 7.455576670931136185 ) ) ;
#37766=CARTESIAN_POINT ( 'NONE',  ( -0.1287570809895602630, -0.3962735484563142396, 10.00000000000000000 ) ) ;
#37780=FACE_OUTER_BOUND ( 'NONE', #20979, .T. ) ;
#37782=EDGE_LOOP ( 'NONE', ( #29553, #8030, #25072, #37893, #21115 ) ) ;
#37784=CARTESIAN_POINT ( 'NONE',  ( 31.28977333267368621, -11.25592690310905652, -2.408242355805840784 ) ) ;
#37785=CARTESIAN_POINT ( 'NONE',  ( 9.281355226777661116, -3.722424633806168615, 0.000000000000000000 ) ) ;
#37787=EDGE_CURVE ( 'NONE', #47273, #12321, #33805, .T. ) ;
#37788=CARTESIAN_POINT ( 'NONE',  ( 0.1265591857323814795, 1.213367045380162823, 9.963925895596176474 ) ) ;
#37791=CARTESIAN_POINT ( 'NONE',  ( 5.320787806771834383, -8.466948512617054945, 0.000000000000000000 ) ) ;
#37806=EDGE_CURVE ( 'NONE', #40331, #32574, #26421, .T. ) ;
#37808=B_SPLINE_CURVE_WITH_KNOTS ( 'NONE', 3,
 ( #30944, #27330, #46530, #11423 ),
 .UNSPECIFIED., .F., .F.,
 ( 4, 4 ),
 ( 0.8097120833243713900, 0.9322955464062561148 ),
 .UNSPECIFIED. ) ;
#37810=CARTESIAN_POINT ( 'NONE',  ( -33.14391172085785797, -37.72293746533095060, -8.016098858316199838 ) ) ;
#37812=CARTESIAN_POINT ( 'NONE',  ( -31.44259251615275019, -38.95901822126145220, -9.367992836599951190 ) ) ;
#37837=EDGE_CURVE ( 'NONE', #6277, #49960, #1362, .T. ) ;
#37860=ORIENTED_EDGE ( 'NONE', *, *, #29637, .T. ) ;
#37861=CARTESIAN_POINT ( 'NONE',  ( -23.79193388295331602, -28.98609808354994044, -9.422646554964178023 ) ) ;
#37865=CARTESIAN_POINT ( 'NONE',  ( 0.3862712429686810944, 1.188820645368943607, 3.333333333333333481 ) ) ;
#37866=CARTESIAN_POINT ( 'NONE',  ( -1.455748852897583268, -0.01196569884525386721, 9.938560165450793349 ) ) ;
#37877=CARTESIAN_POINT ( 'NONE',  ( -23.26005729352344176, -44.90397804740339183, 7.906207997025717304 ) ) ;
#37885=EDGE_CURVE ( 'NONE', #48228, #23523, #33504, .T. ) ;
#37891=ORIENTED_EDGE ( 'NONE', *, *, #40983, .F. ) ;
#37893=ORIENTED_EDGE ( 'NONE', *, *, #12367, .F. ) ;
#37894=EDGE_CURVE ( 'NONE', #12217, #6697, #3144, .T. ) ;
#37899=CARTESIAN_POINT ( 'NONE',  ( 49.46074318306830975, -9.578883844006833570, 8.807470649214879543 ) ) ;
#37901=CARTESIAN_POINT ( 'NONE',  ( -0.09523839817533703844, -1.466467394240187350, 9.958264684458541183 ) ) ;
#37910=CARTESIAN_POINT ( 'NONE',  ( -0.3862712429686895876, 1.188820645368940720, 10.00000000000000000 ) ) ;
#37911=EDGE_CURVE ( 'NONE', #26328, #76, #17792, .T. ) ;
#37922=CARTESIAN_POINT ( 'NONE',  ( -0.1265591857321690383, -1.213367045380180809, 9.963925895596192461 ) ) ;
#37924=CARTESIAN_POINT ( 'NONE',  ( -27.33593271309441519, 41.94268121623345991, -9.367992836599954742 ) ) ;
#37931=CARTESIAN_POINT ( 'NONE',  ( 0.2778388845795309314, -1.251314014313100520, 9.976582533991681601 ) ) ;
#37944=B_SPLINE_SURFACE_WITH_KNOTS ( 'NONE', 3, 3, ( 
 ( #7518, #23153, #38830, #28280 ),
 ( #29034, #40585, #5172, #28782 ),
 ( #40088, #20575, #16229, #12874 ),
 ( #21074, #36759, #12363, #4682 ) ),
 .UNSPECIFIED., .F., .F., .F.,
 ( 4, 4 ),
 ( 4, 4 ),
 ( 0.000000000000000000, 1.000000000000000000 ),
 ( 0.000000000000000000, 1.000000000000000000 ),
 .UNSPECIFIED. ) ;
#37948=EDGE_CURVE ( 'NONE', #12326, #26155, #9252, .T. ) ;
#37953=DIRECTION ( 'NONE',  ( -0.5877852522924625900, -0.8090169943749551118, 0.000000000000000000 ) ) ;
#37965=VERTEX_POINT ( 'NONE', #14492 ) ;
#37973=CARTESIAN_POINT ( 'NONE',  ( -4.763548243873389154, 16.57409059453848599, 8.727788335465566760 ) ) ;
#37982=ORIENTED_EDGE ( 'NONE', *, *, #16414, .T. ) ;
#38000=CARTESIAN_POINT ( 'NONE',  ( -1.011271242968683204, -0.7347315653655928092, 9.972675548442467175 ) ) ;
#38001=ORIENTED_EDGE ( 'NONE', *, *, #44981, .F. ) ;
#38008=B_SPLINE_CURVE_WITH_KNOTS ( 'NONE', 3,
 ( #45743, #45996, #38356, #45244 ),
 .UNSPECIFIED., .F., .F.,
 ( 4, 4 ),
 ( 0.001937412222931627270, 0.003978261222106111578 ),
 .UNSPECIFIED. ) ;
#38011=CARTESIAN_POINT ( 'NONE',  ( -20.21530556545279111, 31.58467066308232063, -9.422646554964174470 ) ) ;
#38014=CARTESIAN_POINT ( 'NONE',  ( -33.86622497129646092, 3.037805405905158462, 7.906207997025717304 ) ) ;
#38021=CARTESIAN_POINT ( 'NONE',  ( 8.277096487746778308, -50.00000000000000000, 7.455576670931136185 ) ) ;
#38026=CARTESIAN_POINT ( 'NONE',  ( 34.95136153415558056, -36.40974830873469870, 8.356839323120299312 ) ) ;
#38041=CARTESIAN_POINT ( 'NONE',  ( -3.087186397306470820, -2.514307945609864259, -2.642742795433417058E-16 ) ) ;
#38045=ORIENTED_EDGE ( 'NONE', *, *, #23979, .F. ) ;
#38047=B_SPLINE_SURFACE_WITH_KNOTS ( 'NONE', 3, 3, ( 
 ( #788, #47683, #8747, #33114 ),
 ( #36725, #20779, #17191, #44365 ),
 ( #12572, #40793, #24402, #36202 ),
 ( #32348, #32861, #40048, #1041 ) ),
 .UNSPECIFIED., .F., .F., .F.,
 ( 4, 4 ),
 ( 4, 4 ),
 ( 0.000000000000000000, 1.000000000000000000 ),
 ( 0.000000000000000000, 1.000000000000000000 ),
 .UNSPECIFIED. ) ;
#38048=CARTESIAN_POINT ( 'NONE',  ( -47.88254548617756967, 14.43607691413558669, -3.760136334089591248 ) ) ;
#38051=ADVANCED_FACE ( 'NONE', ( #27054 ), #11000, .T. ) ;
#38052=B_SPLINE_CURVE_WITH_KNOTS ( 'NONE', 3,
 ( #5594, #16645, #16394, #27950 ),
 .UNSPECIFIED., .F., .F.,
 ( 4, 4 ),
 ( 1.735570302229820823E-18, 2.647279941188451471E-05 ),
 .UNSPECIFIED. ) ;
#38064=CARTESIAN_POINT ( 'NONE',  ( 44.99506233596247995, 23.32283626942318833, 7.455576670931136185 ) ) ;
#38073=CARTESIAN_POINT ( 'NONE',  ( 0.4430829022285069918, 1.527139474549929155, 9.933337522700155020 ) ) ;
#38078=CARTESIAN_POINT ( 'NONE',  ( 4.353119224256710496, 9.002796955358187247, 0.000000000000000000 ) ) ;
#38081=ORIENTED_EDGE ( 'NONE', *, *, #12171, .F. ) ;
#38084=ORIENTED_EDGE ( 'NONE', *, *, #17063, .F. ) ;
#38089=ORIENTED_EDGE ( 'NONE', *, *, #12037, .T. ) ;
#38091=ORIENTED_EDGE ( 'NONE', *, *, #50390, .T. ) ;
#38095=CARTESIAN_POINT ( 'NONE',  ( -0.9599924130074112272, 0.8495346730527952861, 9.948547179989619238 ) ) ;
#38097=DIRECTION ( 'NONE',  ( -0.000000000000000000, -0.000000000000000000, -1.000000000000000000 ) ) ;
#38102=CARTESIAN_POINT ( 'NONE',  ( -47.88254548617756967, 14.43607691413558669, -3.760136334089591248 ) ) ;
#38108=LINE ( 'NONE', #17831, #1524 ) ;
#38117=EDGE_CURVE ( 'NONE', #43972, #32354, #20248, .T. ) ;
#38122=CARTESIAN_POINT ( 'NONE',  ( 12.16428377685533313, 11.73151505502934810, -9.008049429158102583 ) ) ;
#38129=CARTESIAN_POINT ( 'NONE',  ( 1.011271242968677653, 0.7347315653656002477, -3.333333333333333481 ) ) ;
#38130=CARTESIAN_POINT ( 'NONE',  ( -0.7849184246622071814, 1.242376769534369041, 9.958264684458713489 ) ) ;
#38135=CARTESIAN_POINT ( 'NONE',  ( -5.320787806781440921, 8.466948512633457824, -1.544988095791843818E-15 ) ) ;
#38141=DIRECTION ( 'NONE',  ( 0.000000000000000000, 0.000000000000000000, -1.000000000000000000 ) ) ;
#38144=ORIENTED_EDGE ( 'NONE', *, *, #2473, .T. ) ;
#38147=( GEOMETRIC_REPRESENTATION_CONTEXT ( 3 ) GLOBAL_UNCERTAINTY_ASSIGNED_CONTEXT ( ( #50562 ) ) GLOBAL_UNIT_ASSIGNED_CONTEXT ( ( #5960, #22622, #9804 ) ) REPRESENTATION_CONTEXT ( 'NONE', 'WORKASPACE' ) );
#38151=CARTESIAN_POINT ( 'NONE',  ( -17.34922095635781147, -33.24536858281880569, 8.914903342594564961 ) ) ;
#38153=FACE_OUTER_BOUND ( 'NONE', #20006, .T. ) ;
#38160=LINE ( 'NONE', #12833, #20163 ) ;
#38161=CARTESIAN_POINT ( 'NONE',  ( 2.089000987151460986, 7.666878472665119126, 9.432811472610055148 ) ) ;
#38180=VECTOR ( 'NONE', #46605, 1000.000000000000114 ) ;
#38185=CARTESIAN_POINT ( 'NONE',  ( 27.33593271309472073, -41.94268121623323964, -9.367992836599954742 ) ) ;
#38187=ADVANCED_FACE ( 'NONE', ( #24482 ), #25737, .T. ) ;
#38189=CARTESIAN_POINT ( 'NONE',  ( -1.377509002708424468, 0.6027468487255034368, 9.927319414211229542 ) ) ;
#38200=EDGE_CURVE ( 'NONE', #14294, #49029, #17154, .T. ) ;
#38203=ORIENTED_EDGE ( 'NONE', *, *, #6276, .F. ) ;
#38209=CARTESIAN_POINT ( 'NONE',  ( -30.87089393895367095, 12.69923079256638587, -9.367992836599954742 ) ) ;
#38212=PLANE ( 'NONE',  #20683 ) ;
#38222=CARTESIAN_POINT ( 'NONE',  ( -3.345242017215803276, 2.159124855890678596, -2.642742795433417058E-16 ) ) ;
#38226=EDGE_LOOP ( 'NONE', ( #1729, #46365, #48032, #18994, #40950, #48, #18618, #45323, #45801, #50544, #45960, #20595, #46809, #48609, #13446, #32016, #9312, #24367, #35987, #32338, #7370, #44037, #3805, #48568, #6948 ) ) ;
#38240=CARTESIAN_POINT ( 'NONE',  ( 34.38425513258721367, -36.82177522737821107, 8.807470649214879543 ) ) ;
#38251=CARTESIAN_POINT ( 'NONE',  ( -1.401228687704686449, 0.7134216605328093097, 9.945241992664930919 ) ) ;
#38254=EDGE_CURVE ( 'NONE', #38752, #50500, #22694, .T. ) ;
#38274=CARTESIAN_POINT ( 'NONE',  ( 3.087186397306452612, 2.514307945609885131, -2.642742795433417058E-16 ) ) ;
#38278=CARTESIAN_POINT ( 'NONE',  ( -33.43156050989129824, 4.370686678976795747, 8.807470649214879543 ) ) ;
#38279=CARTESIAN_POINT ( 'NONE',  ( -0.7139173712339883515, 1.401061409226810994, 9.927288994922816912 ) ) ;
#38282=B_SPLINE_CURVE_WITH_KNOTS ( 'NONE', 3,
 ( #16482, #335, #39846, #46974 ),
 .UNSPECIFIED., .F., .F.,
 ( 4, 4 ),
 ( 0.8097120833243680593, 0.9322955464062561148 ),
 .UNSPECIFIED. ) ;
#38289=VERTEX_POINT ( 'NONE', #29334 ) ;
#38291=CARTESIAN_POINT ( 'NONE',  ( -1.011271242968683426, -0.7347315653655928092, 10.00000000000000000 ) ) ;
#38292=CARTESIAN_POINT ( 'NONE',  ( 26.18032376592674737, -21.95228666728361233, 7.455576670931136185 ) ) ;
#38295=ORIENTED_EDGE ( 'NONE', *, *, #21373, .F. ) ;
#38296=CARTESIAN_POINT ( 'NONE',  ( -13.35436367797847801, -31.26996044524040741, 7.906207997025717304 ) ) ;
#38298=CARTESIAN_POINT ( 'NONE',  ( 1.011271242968677653, 0.7347315653656002477, 3.333333333333333481 ) ) ;
#38309=ORIENTED_EDGE ( 'NONE', *, *, #46224, .F. ) ;
#38310=CARTESIAN_POINT ( 'NONE',  ( 46.11867747200574996, -19.86470446310233484, -8.016098858316199838 ) ) ;
#38321=ORIENTED_EDGE ( 'NONE', *, *, #6413, .T. ) ;
#38323=CARTESIAN_POINT ( 'NONE',  ( -1.133908876584336367, -0.5183204401656656968, 9.981352469109934233 ) ) ;
#38325=CARTESIAN_POINT ( 'NONE',  ( 48.33712804702526000, 13.03701565032775456, -9.367992836599954742 ) ) ;
#38330=ORIENTED_EDGE ( 'NONE', *, *, #16147, .T. ) ;
#38331=CARTESIAN_POINT ( 'NONE',  ( -5.505322767148756569, 37.09368438467003415, 8.914903342594564961 ) ) ;
#38332=CARTESIAN_POINT ( 'NONE',  ( 0.1425549192113746144, -1.238581250503543618, 9.981352469109934233 ) ) ;
#38344=ORIENTED_EDGE ( 'NONE', *, *, #42799, .F. ) ;
#38349=CARTESIAN_POINT ( 'NONE',  ( -28.96803024440907137, -18.11533787072017176, 7.455576670931136185 ) ) ;
#38355=CARTESIAN_POINT ( 'NONE',  ( -26.18032376592659105, 21.95228666728381128, 7.455576670931136185 ) ) ;
#38356=CARTESIAN_POINT ( 'NONE',  ( 2.892039187330371242, -1.502206308778212929, 9.799352050262459812 ) ) ;
#38357=CARTESIAN_POINT ( 'NONE',  ( -15.62858259096117841, 5.755205073598721910, -9.683996418299976483 ) ) ;
#38364=B_SPLINE_SURFACE_WITH_KNOTS ( 'NONE', 3, 3, ( 
 ( #2684, #7053, #38366, #34511 ),
 ( #50090, #29889, #45509, #22198 ),
 ( #10397, #15003, #46509, #37865 ),
 ( #46259, #11401, #11157, #18321 ) ),
 .UNSPECIFIED., .F., .F., .F.,
 ( 4, 4 ),
 ( 4, 4 ),
 ( 0.000000000000000000, 1.000000000000000000 ),
 ( 0.000000000000000000, 1.000000000000000000 ),
 .UNSPECIFIED. ) ;
#38366=CARTESIAN_POINT ( 'NONE',  ( -14.91630425054805187, 7.943683830272224355, -9.008049429158100807 ) ) ;
#38371=CARTESIAN_POINT ( 'NONE',  ( 31.93002621080262671, 9.285431160462559674, -2.408242355805840784 ) ) ;
#38378=CARTESIAN_POINT ( 'NONE',  ( -1.565984505217804967, 1.491012526244388070, 9.885585981620945262 ) ) ;
#38384=CARTESIAN_POINT ( 'NONE',  ( -0.5705203167777310735, -1.169354363542817854, 9.986087673579140400 ) ) ;
#38390=CARTESIAN_POINT ( 'NONE',  ( -7.576114424932982594, 33.14742743729794938, 7.906207997025717304 ) ) ;
#38393=ORIENTED_EDGE ( 'NONE', *, *, #32612, .F. ) ;
#38400=ORIENTED_EDGE ( 'NONE', *, *, #22690, .F. ) ;
#38402=LINE ( 'NONE', #25831, #43165 ) ;
#38406=VERTEX_POINT ( 'NONE', #20561 ) ;
#38409=CARTESIAN_POINT ( 'NONE',  ( -0.9870575514055066613, -1.980598328282574316, 9.881002359080278907 ) ) ;
#38414=CARTESIAN_POINT ( 'NONE',  ( 31.28234235046230793, 11.28615439405779064, -3.760136334089591248 ) ) ;
#38422=CARTESIAN_POINT ( 'NONE',  ( -2.134700047865557782, -5.564249483241940908, 1.036768327439263615E-15 ) ) ;
#38425=CARTESIAN_POINT ( 'NONE',  ( 48.77035878734821495, 11.70366853303760379, -8.466730184410787174 ) ) ;
#38438=CARTESIAN_POINT ( 'NONE',  ( -0.5391684635142623971, 1.495919383164612926, 9.933337522700158573 ) ) ;
#38445=B_SPLINE_CURVE_WITH_KNOTS ( 'NONE', 3,
 ( #3961, #16275, #11926, #35293 ),
 .UNSPECIFIED., .F., .F.,
 ( 4, 4 ),
 ( 0.9811748202683098219, 0.9878904167554126703 ),
 .UNSPECIFIED. ) ;
#38454=ADVANCED_FACE ( 'NONE', ( #43391, #39569, #24172, #35977, #820, #16466 ), #32117, .T. ) ;
#38458=CARTESIAN_POINT ( 'NONE',  ( -0.4548599190037587725, -1.225298710497772836, 9.945465957785113886 ) ) ;
#38473=CARTESIAN_POINT ( 'NONE',  ( 1.011271242968694084, -0.7347315653655782652, -3.333333333333333481 ) ) ;
#38474=EDGE_CURVE ( 'NONE', #31155, #23256, #35535, .T. ) ;
#38476=CARTESIAN_POINT ( 'NONE',  ( 15.73090589902275482, 29.60029367929053024, 1.847720168420772691 ) ) ;
#38477=B_SPLINE_SURFACE_WITH_KNOTS ( 'NONE', 3, 3, ( 
 ( #48854, #26315, #45526, #22210 ),
 ( #34267, #9898, #22455, #13742 ),
 ( #2209, #45270, #41956, #38129 ),
 ( #6046, #14756, #2944, #18338 ) ),
 .UNSPECIFIED., .F., .F., .F.,
 ( 4, 4 ),
 ( 4, 4 ),
 ( 0.000000000000000000, 1.000000000000000000 ),
 ( 0.000000000000000000, 1.000000000000000000 ),
 .UNSPECIFIED. ) ;
#38479=EDGE_CURVE ( 'NONE', #24866, #14725, #33706, .T. ) ;
#38480=CARTESIAN_POINT ( 'NONE',  ( 2.538055338523177440, 33.28424297489108596, -9.367992836599954742 ) ) ;
#38483=CARTESIAN_POINT ( 'NONE',  ( -8.277096487746778308, 50.00000000000000711, 7.455576670931136185 ) ) ;
#38487=CARTESIAN_POINT ( 'NONE',  ( 8.843309649387377291, -14.11631751497145792, -2.870787844569587133 ) ) ;
#38501=CARTESIAN_POINT ( 'NONE',  ( -29.39982726364978660, -16.78152490921149109, 8.356839323120299312 ) ) ;
#38503=CARTESIAN_POINT ( 'NONE',  ( -44.99506233596264337, -23.32283626942287214, 7.455576670931136185 ) ) ;
#38512=ORIENTED_EDGE ( 'NONE', *, *, #19134, .F. ) ;
#38531=CARTESIAN_POINT ( 'NONE',  ( 0.2050626648100478400, -1.807624707196173519, 9.903764339332001398 ) ) ;
#38533=CARTESIAN_POINT ( 'NONE',  ( 0.4098590526157686598, 3.751478160727024225, 9.865049507598756762 ) ) ;
#38534=CIRCLE ( 'NONE', #33575, 10.00000000000000000 ) ;
#38538=CARTESIAN_POINT ( 'NONE',  ( -1.286508520037554337, -0.4866366830703409141, 9.972175347158394487 ) ) ;
#38560=FACE_OUTER_BOUND ( 'NONE', #22472, .T. ) ;
#38567=CARTESIAN_POINT ( 'NONE',  ( -0.3862712429686889770, 1.188820645368940720, 9.972675548442463622 ) ) ;
#38576=EDGE_CURVE ( 'NONE', #21273, #46833, #44885, .T. ) ;
#38580=CARTESIAN_POINT ( 'NONE',  ( 14.29087950072012170, 9.652079258044652832, 8.727788335465566760 ) ) ;
#38583=EDGE_LOOP ( 'NONE', ( #28299, #49366, #36914, #42809, #10668, #6323, #446, #35114, #21972, #38599, #1280, #13314, #42275, #15024, #22555 ) ) ;
#38589=CARTESIAN_POINT ( 'NONE',  ( 34.76907794179066258, -14.14424844080153498, -5.338708898921614932 ) ) ;
#38598=CARTESIAN_POINT ( 'NONE',  ( 9.281355226777661116, -3.722424633806168615, 0.000000000000000000 ) ) ;
#38599=ORIENTED_EDGE ( 'NONE', *, *, #30941, .F. ) ;
#38601=ORIENTED_EDGE ( 'NONE', *, *, #11521, .F. ) ;
#38605=CARTESIAN_POINT ( 'NONE',  ( 0.1188999517099294939, 1.297929763951737758, 9.961915419665734461 ) ) ;
#38614=CARTESIAN_POINT ( 'NONE',  ( 7.129058724844953510, 15.30620660340485095, 9.178419661560148768 ) ) ;
#38616=VERTEX_POINT ( 'NONE', #11029 ) ;
#38617=CARTESIAN_POINT ( 'NONE',  ( -1.072341519476054827, 1.326978504731037845, 9.912102921405034905 ) ) ;
#38639=CARTESIAN_POINT ( 'NONE',  ( -1.249999999999999778, 0.000000000000000000, -10.00000000000000000 ) ) ;
#38641=ORIENTED_EDGE ( 'NONE', *, *, #42341, .T. ) ;
#38645=VERTEX_POINT ( 'NONE', #42570 ) ;
#38647=B_SPLINE_CURVE_WITH_KNOTS ( 'NONE', 3,
 ( #32693, #33217, #45206, #13437 ),
 .UNSPECIFIED., .F., .F.,
 ( 4, 4 ),
 ( 0.000000000000000000, 0.002368422649471297291 ),
 .UNSPECIFIED. ) ;
#38666=CARTESIAN_POINT ( 'NONE',  ( 27.33593271309472073, -41.94268121623323964, -9.367992836599954742 ) ) ;
#38678=CARTESIAN_POINT ( 'NONE',  ( -0.4166666666666669072, 0.000000000000000000, 10.00000000000000000 ) ) ;
#38679=CARTESIAN_POINT ( 'NONE',  ( -49.67735855322972327, 8.912210285362091255, 8.356839323120299312 ) ) ;
#38687=ORIENTED_EDGE ( 'NONE', *, *, #4500, .T. ) ;
#38692=ORIENTED_EDGE ( 'NONE', *, *, #32612, .T. ) ;
#38699=CARTESIAN_POINT ( 'NONE',  ( -0.3862712429686809279, -1.188820645368943163, -10.00000000000000000 ) ) ;
#38713=EDGE_LOOP ( 'NONE', ( #26211, #3370, #36652 ) ) ;
#38714=EDGE_LOOP ( 'NONE', ( #32970, #24235, #36885, #30738 ) ) ;
#38715=CARTESIAN_POINT ( 'NONE',  ( -1.288422560825909224, 0.1812466941682708832, 9.986087673579197244 ) ) ;
#38720=EDGE_CURVE ( 'NONE', #24051, #39174, #4311, .T. ) ;
#38740=CARTESIAN_POINT ( 'NONE',  ( -7.749480817862350435, -14.85497772329513211, 9.403735324607438884 ) ) ;
#38742=CARTESIAN_POINT ( 'NONE',  ( 0.3862712429686727678, 1.188820645368945605, -10.00000000000000000 ) ) ;
#38743=CARTESIAN_POINT ( 'NONE',  ( 5.923309489234873659, -5.336940131180849534, 8.131516293641283255E-16 ) ) ;
#38752=VERTEX_POINT ( 'NONE', #16152 ) ;
#38760=ORIENTED_EDGE ( 'NONE', *, *, #43705, .T. ) ;
#38764=ORIENTED_EDGE ( 'NONE', *, *, #29658, .T. ) ;
#38771=CARTESIAN_POINT ( 'NONE',  ( -33.26055721649984775, -17.33465289285453181, 8.506357886886743103 ) ) ;
#38782=B_SPLINE_SURFACE_WITH_KNOTS ( 'NONE', 3, 3, ( 
 ( #29555, #6456, #13396, #2359 ),
 ( #9305, #37784, #2598, #24967 ),
 ( #5448, #36782, #29060, #48763 ),
 ( #44679, #41109, #44921, #9559 ) ),
 .UNSPECIFIED., .F., .F., .F.,
 ( 4, 4 ),
 ( 4, 4 ),
 ( 0.000000000000000000, 1.000000000000000000 ),
 ( 0.000000000000000000, 1.000000000000000000 ),
 .UNSPECIFIED. ) ;
#38790=CARTESIAN_POINT ( 'NONE',  ( 17.23491422248386584, -0.5912720620000816441, 8.727788335465566760 ) ) ;
#38793=CARTESIAN_POINT ( 'NONE',  ( 45.42829307628542779, 21.98948915213303579, 8.356839323120299312 ) ) ;
#38807=CARTESIAN_POINT ( 'NONE',  ( -50.11058929355266400, 7.578863168071933387, 7.455576670931136185 ) ) ;
#38808=CARTESIAN_POINT ( 'NONE',  ( 4.376737514451251698, -37.28021197136517628, 1.982731392810406668 ) ) ;
#38829=CARTESIAN_POINT ( 'NONE',  ( -8.813458710706198573, -4.724716452304520864, 0.000000000000000000 ) ) ;
#38830=CARTESIAN_POINT ( 'NONE',  ( 16.52264463346132572, -2.779753662172757878, 9.403735324607438884 ) ) ;
#38836=B_SPLINE_CURVE_WITH_KNOTS ( 'NONE', 3,
 ( #15440, #11338, #31096, #42624 ),
 .UNSPECIFIED., .F., .F.,
 ( 4, 4 ),
 ( 0.000000000000000000, 0.2637263876330694368 ),
 .UNSPECIFIED. ) ;
#38852=CARTESIAN_POINT ( 'NONE',  ( 1.066995270233474624, -33.23888904628638841, -3.760136334089591248 ) ) ;
#38857=CARTESIAN_POINT ( 'NONE',  ( -48.98697415750977058, -11.03699497439218291, -8.016098858316205167 ) ) ;
#38874=CARTESIAN_POINT ( 'NONE',  ( 28.97821631107911600, 35.56709536735927912, -9.367992836599951190 ) ) ;
#38897=CARTESIAN_POINT ( 'NONE',  ( 7.576114424932982594, -33.14742743729794938, 7.906207997025717304 ) ) ;
#38901=CARTESIAN_POINT ( 'NONE',  ( -9.281355226777547429, 3.722424633806451943, 0.000000000000000000 ) ) ;
#38903=ORIENTED_EDGE ( 'NONE', *, *, #9534, .F. ) ;
#38909=ORIENTED_EDGE ( 'NONE', *, *, #38720, .T. ) ;
#38920=ORIENTED_EDGE ( 'NONE', *, *, #24583, .F. ) ;
#38941=CARTESIAN_POINT ( 'NONE',  ( 1.250000000000000222, 0.000000000000000000, 3.333333333333333481 ) ) ;
#38943=ORIENTED_EDGE ( 'NONE', *, *, #20926, .F. ) ;
#38957=CARTESIAN_POINT ( 'NONE',  ( -0.3862712429686889770, 1.188820645368940720, 9.972675548442463622 ) ) ;
#38961=CARTESIAN_POINT ( 'NONE',  ( -0.5113015165352315927, -1.175527691268679398, 9.948547179989621014 ) ) ;
#38983=CARTESIAN_POINT ( 'NONE',  ( -1.337801958641930300, -1.088266084286974689, 9.928159647716134018 ) ) ;
#38990=B_SPLINE_CURVE_WITH_KNOTS ( 'NONE', 3,
 ( #29779, #2567, #3069, #6934 ),
 .UNSPECIFIED., .F., .F.,
 ( 4, 4 ),
 ( 0.000000000000000000, 0.0001252128669263108287 ),
 .UNSPECIFIED. ) ;
#39015=ORIENTED_EDGE ( 'NONE', *, *, #10493, .T. ) ;
#39033=CARTESIAN_POINT ( 'NONE',  ( -25.45361382821521445, 27.58774327458509390, 1.982731392810406668 ) ) ;
#39043=CARTESIAN_POINT ( 'NONE',  ( 0.4152287376636409899, -2.070986276654470881, 9.884520316594377576 ) ) ;
#39049=CARTESIAN_POINT ( 'NONE',  ( 31.94178169330218964, -9.256608784833820991, -3.760136334089591248 ) ) ;
#39053=CARTESIAN_POINT ( 'NONE',  ( 9.260964247899973856, -13.84230907185609460, -9.683996418299976483 ) ) ;
#39054=ORIENTED_EDGE ( 'NONE', *, *, #25591, .F. ) ;
#39065=CARTESIAN_POINT ( 'NONE',  ( -0.3862712429686729343, -1.188820645368946050, -3.333333333333333481 ) ) ;
#39066=CARTESIAN_POINT ( 'NONE',  ( -16.16402646813540755, 4.033894069732547827, -3.546734833711462365 ) ) ;
#39077=CARTESIAN_POINT ( 'NONE',  ( -7.749480817862350435, -14.85497772329513211, 9.403735324607438884 ) ) ;
#39079=CARTESIAN_POINT ( 'NONE',  ( -24.39427009666018265, -44.07992421011638129, 8.807470649214879543 ) ) ;
#39081=CARTESIAN_POINT ( 'NONE',  ( -1.011271242968693862, 0.7347315653655780432, -10.00000000000000000 ) ) ;
#39096=B_SPLINE_CURVE_WITH_KNOTS ( 'NONE', 3,
 ( #38567, #3379, #27258, #45955 ),
 .UNSPECIFIED., .F., .F.,
 ( 4, 4 ),
 ( 0.000000000000000000, 0.0002610106747150458747 ),
 .UNSPECIFIED. ) ;
#39121=ORIENTED_EDGE ( 'NONE', *, *, #27402, .T. ) ;
#39124=CARTESIAN_POINT ( 'NONE',  ( 13.92102703536701114, 30.85732372859822803, 8.356839323120299312 ) ) ;
#39128=ORIENTED_EDGE ( 'NONE', *, *, #42214, .T. ) ;
#39136=CARTESIAN_POINT ( 'NONE',  ( 34.94239438780391538, 13.71128139791418832, 3.209567239418968487 ) ) ;
#39143=CARTESIAN_POINT ( 'NONE',  ( 0.7849184246612691540, -1.242376769536456704, 9.958264684458541183 ) ) ;
#39149=ORIENTED_EDGE ( 'NONE', *, *, #47845, .T. ) ;
#39151=CARTESIAN_POINT ( 'NONE',  ( 0.06526599240121484791, -1.373921316406707449, 9.972175347158280800 ) ) ;
#39152=CARTESIAN_POINT ( 'NONE',  ( 24.47767542868285062, -23.18653802921781448, 8.807470649214879543 ) ) ;
#39160=ORIENTED_EDGE ( 'NONE', *, *, #5765, .F. ) ;
#39162=CARTESIAN_POINT ( 'NONE',  ( -0.4166666666666669072, 0.000000000000000000, 10.00000000000000000 ) ) ;
#39164=CARTESIAN_POINT ( 'NONE',  ( 0.7601424845489945792, -1.297311920616997627, 9.927319414211225990 ) ) ;
#39166=VERTEX_POINT ( 'NONE', #5027 ) ;
#39172=EDGE_CURVE ( 'NONE', #290, #11134, #23284, .T. ) ;
#39174=VERTEX_POINT ( 'NONE', #12975 ) ;
#39175=ADVANCED_FACE ( 'NONE', ( #28635 ), #25304, .T. ) ;
#39176=CYLINDRICAL_SURFACE ( 'NONE', #27441, 10.00000000000000000 ) ;
#39183=CARTESIAN_POINT ( 'NONE',  ( 1.011271242968677653, 0.7347315653656002477, -10.00000000000000000 ) ) ;
#39193=CARTESIAN_POINT ( 'NONE',  ( -33.64889274059387958, 3.704246042440976439, 8.356839323120299312 ) ) ;
#39204=B_SPLINE_SURFACE_WITH_KNOTS ( 'NONE', 3, 3, ( 
 ( #46251, #23457, #42427, #7289 ),
 ( #15256, #49826, #50343, #18821 ),
 ( #38102, #27042, #30395, #30916 ),
 ( #7046, #22684, #38357, #46499 ) ),
 .UNSPECIFIED., .F., .F., .F.,
 ( 4, 4 ),
 ( 4, 4 ),
 ( 0.000000000000000000, 1.000000000000000000 ),
 ( 0.000000000000000000, 1.000000000000000000 ),
 .UNSPECIFIED. ) ;
#39206=ORIENTED_EDGE ( 'NONE', *, *, #42405, .F. ) ;
#39213=CARTESIAN_POINT ( 'NONE',  ( 17.34922095635755568, 33.24536858281893359, 8.914903342594564961 ) ) ;
#39224=ORIENTED_EDGE ( 'NONE', *, *, #35100, .F. ) ;
#39226=CARTESIAN_POINT ( 'NONE',  ( 33.14391172085757375, 37.72293746533119929, -8.016098858316199838 ) ) ;
#39233=CARTESIAN_POINT ( 'NONE',  ( 0.3862712429686894766, -1.188820645368940276, 10.00000000000000000 ) ) ;
#39234=CARTESIAN_POINT ( 'NONE',  ( -3.229232847726260403, 16.57333684275945629, 9.178419661560148768 ) ) ;
#39237=CARTESIAN_POINT ( 'NONE',  ( -1.275927284277175167, 0.1224368140627496299, 9.976582533991679824 ) ) ;
#39238=B_SPLINE_CURVE_WITH_KNOTS ( 'NONE', 3,
 ( #5580, #17879, #33558, #44550 ),
 .UNSPECIFIED., .F., .F.,
 ( 4, 4 ),
 ( 0.000000000000000000, 0.0002610106747335709325 ),
 .UNSPECIFIED. ) ;
#39239=CARTESIAN_POINT ( 'NONE',  ( 45.35314062630785514, -8.244242869018759023, 8.807470649214881320 ) ) ;
#39241=CARTESIAN_POINT ( 'NONE',  ( -9.760995290733800900, 2.173239732351794462, 9.646707543097347681 ) ) ;
#39254=CARTESIAN_POINT ( 'NONE',  ( -0.9983599181300891745, -1.124146016603549070, 9.953784399990620813 ) ) ;
#39263=ORIENTED_EDGE ( 'NONE', *, *, #20553, .T. ) ;
#39287=CARTESIAN_POINT ( 'NONE',  ( -32.43949840348904701, -7.871562655726277669, -9.367992836599951190 ) ) ;
#39292=CARTESIAN_POINT ( 'NONE',  ( 0.3862712429686727678, 1.188820645368945605, -10.00000000000000000 ) ) ;
#39295=ADVANCED_FACE ( 'NONE', ( #10648 ), #36798, .T. ) ;
#39299=PRODUCT_CONTEXT ( 'NONE', #21692, 'mechanical' ) ;
#39305=CARTESIAN_POINT ( 'NONE',  ( 2.418900724918336298, 41.61933801977895087, -9.387872844313825738 ) ) ;
#39314=EDGE_CURVE ( 'NONE', #40295, #24192, #41594, .T. ) ;
#39317=ORIENTED_EDGE ( 'NONE', *, *, #17055, .F. ) ;
#39320=FACE_OUTER_BOUND ( 'NONE', #14895, .T. ) ;
#39321=CARTESIAN_POINT ( 'NONE',  ( -1.011271242968693862, 0.7347315653655780432, -3.333333333333333481 ) ) ;
#39334=CARTESIAN_POINT ( 'NONE',  ( -0.5107275442771143092, -1.175643901748072873, 9.976582533991681601 ) ) ;
#39341=VERTEX_POINT ( 'NONE', #28774 ) ;
#39362=CARTESIAN_POINT ( 'NONE',  ( -14.52758583651993618, -8.922352469211071835, 8.953103998512858652 ) ) ;
#39368=FACE_OUTER_BOUND ( 'NONE', #32720, .T. ) ;
#39378=CARTESIAN_POINT ( 'NONE',  ( 1.249999999999999778, 0.000000000000000000, 10.00000000000000000 ) ) ;
#39389=CARTESIAN_POINT ( 'NONE',  ( -14.52758583651993618, -8.922352469211071835, 8.953103998512858652 ) ) ;
#39406=CARTESIAN_POINT ( 'NONE',  ( 24.39427009665985224, 44.07992421011656603, 8.807470649214879543 ) ) ;
#39413=VERTEX_POINT ( 'NONE', #33149 ) ;
#39419=CARTESIAN_POINT ( 'NONE',  ( 7.576114424932982594, -33.14742743729794938, 7.906207997025717304 ) ) ;
#39426=CARTESIAN_POINT ( 'NONE',  ( 1.011271242968688311, -0.7347315653655855927, -10.00000000000000000 ) ) ;
#39430=CARTESIAN_POINT ( 'NONE',  ( 16.02661358026014327, 4.530191650547718218, -9.683996418299976483 ) ) ;
#39432=ORIENTED_EDGE ( 'NONE', *, *, #37787, .T. ) ;
#39436=CARTESIAN_POINT ( 'NONE',  ( 30.25247992116058526, -39.82368563463805344, -3.760136334089591248 ) ) ;
#39439=CARTESIAN_POINT ( 'NONE',  ( -0.5113015165352315927, -1.175527691268679398, 9.948547179989621014 ) ) ;
#39444=CARTESIAN_POINT ( 'NONE',  ( -16.52264463346130796, 2.779753662172870232, 9.403735324607438884 ) ) ;
#39447=ORIENTED_EDGE ( 'NONE', *, *, #255, .F. ) ;
#39454=DIRECTION ( 'NONE',  ( -1.000000000000000000, 0.000000000000000000, -0.000000000000000000 ) ) ;
#39455=CARTESIAN_POINT ( 'NONE',  ( -3.951902932896436571, -0.4322042056279351008, 3.247138655587367140 ) ) ;
#39470=CARTESIAN_POINT ( 'NONE',  ( 1.655785408456140084, 0.7536129375913136474, 9.903764339332061795 ) ) ;
#39480=ORIENTED_EDGE ( 'NONE', *, *, #16414, .F. ) ;
#39493=CARTESIAN_POINT ( 'NONE',  ( -5.083187235775261215, -8.611690166631138510, 9.646707543097347681 ) ) ;
#39495=CARTESIAN_POINT ( 'NONE',  ( -0.2050626648094178439, 1.807624707194796843, 9.903764339332081335 ) ) ;
#39507=CARTESIAN_POINT ( 'NONE',  ( 4.632259372452904422, -3.749670805219074143, 1.768604793866979108E-15 ) ) ;
#39508=CARTESIAN_POINT ( 'NONE',  ( -33.43156050989129824, 4.370686678976795747, 8.807470649214879543 ) ) ;
#39531=B_SPLINE_CURVE_WITH_KNOTS ( 'NONE', 3,
 ( #8389, #4533, #30987, #46334 ),
 .UNSPECIFIED., .F., .F.,
 ( 4, 4 ),
 ( 0.9895749839358303213, 1.000000000000000000 ),
 .UNSPECIFIED. ) ;
#39548=CARTESIAN_POINT ( 'NONE',  ( 0.3904210042914120771, -2.126747006146346930, 9.882710035074770971 ) ) ;
#39550=ORIENTED_EDGE ( 'NONE', *, *, #13057, .F. ) ;
#39552=CARTESIAN_POINT ( 'NONE',  ( -2.052549611693787135, 0.2039603569406744088, 9.894754715216729224 ) ) ;
#39560=CARTESIAN_POINT ( 'NONE',  ( -12.15085308559838317, 11.68662139125813226, 2.590526750877053086 ) ) ;
#39567=CARTESIAN_POINT ( 'NONE',  ( 2.052549611693792464, -0.2039603569406628347, 9.894754715216725671 ) ) ;
#39569=FACE_BOUND ( 'NONE', #27322, .T. ) ;
#39581=CARTESIAN_POINT ( 'NONE',  ( -4.207128120815918256E-14, 3.058192377181588826E-14, 10.00000000000000000 ) ) ;
#39597=CARTESIAN_POINT ( 'NONE',  ( -8.831420117243776957, -14.12636088103186260, -3.546734833711462365 ) ) ;
#39599=B_SPLINE_CURVE_WITH_KNOTS ( 'NONE', 3,
 ( #7597, #19891, #30961, #42982, #46546, #23231 ),
 .UNSPECIFIED., .F., .F.,
 ( 4, 2, 4 ),
 ( 4.629632144690684174E-17, 0.009882509389272370673, 0.01976501877854469624 ),
 .UNSPECIFIED. ) ;
#39604=ORIENTED_EDGE ( 'NONE', *, *, #17733, .F. ) ;
#39615=CARTESIAN_POINT ( 'NONE',  ( 9.563755223200855582, 2.971660568388050372, 3.215106848023521646 ) ) ;
#39621=CARTESIAN_POINT ( 'NONE',  ( -2.538055338523177440, -33.28424297489108596, -9.367992836599954742 ) ) ;
#39624=ORIENTED_EDGE ( 'NONE', *, *, #36629, .T. ) ;
#39626=B_SPLINE_SURFACE_WITH_KNOTS ( 'NONE', 3, 3, ( 
 ( #14724, #33983, #48820, #45736 ),
 ( #10873, #30386, #26530, #42169 ),
 ( #13710, #362, #39362, #35516 ),
 ( #46244, #38349, #23183, #3421 ) ),
 .UNSPECIFIED., .F., .F., .F.,
 ( 4, 4 ),
 ( 4, 4 ),
 ( 0.000000000000000000, 1.000000000000000000 ),
 ( 0.000000000000000000, 1.000000000000000000 ),
 .UNSPECIFIED. ) ;
#39647=FACE_OUTER_BOUND ( 'NONE', #22569, .T. ) ;
#39653=CARTESIAN_POINT ( 'NONE',  ( -0.8101545402525901496, -3.892041480676482479, 3.247138655587363587 ) ) ;
#39654=CARTESIAN_POINT ( 'NONE',  ( -6.875132362119187768, 50.00000000000000711, 8.356839323120299312 ) ) ;
#39660=CARTESIAN_POINT ( 'NONE',  ( 0.1287570809895604018, 0.3962735484563146282, 10.00000000000000000 ) ) ;
#39668=CARTESIAN_POINT ( 'NONE',  ( 1.011271242968688311, -0.7347315653655855927, 3.333333333333333481 ) ) ;
#39687=CARTESIAN_POINT ( 'NONE',  ( 1.011271242968683648, 0.7347315653655930312, 10.00000000000000000 ) ) ;
#39691=CARTESIAN_POINT ( 'NONE',  ( 1.011271242968683648, 0.7347315653655930312, -3.333333333333333481 ) ) ;
#39701=EDGE_CURVE ( 'NONE', #5897, #23745, #44617, .T. ) ;
#39715=CARTESIAN_POINT ( 'NONE',  ( 2.188678504086826848, -0.3267089737525829540, 9.881002359080282460 ) ) ;
#39716=CARTESIAN_POINT ( 'NONE',  ( -41.18776771165107675, 7.147140551973688360, 8.846626183609803462 ) ) ;
#39728=CARTESIAN_POINT ( 'NONE',  ( 34.38425513258721367, -36.82177522737821107, 8.807470649214879543 ) ) ;
#39754=CARTESIAN_POINT ( 'NONE',  ( 9.999999999999998224, 1.843143693225357538E-15, 8.340239149798797769 ) ) ;
#39758=CARTESIAN_POINT ( 'NONE',  ( 0.000000000000000000, -50.00000000000000000, 0.000000000000000000 ) ) ;
#39761=CARTESIAN_POINT ( 'NONE',  ( 0.3862712429686810944, 1.188820645368943607, 10.00000000000000000 ) ) ;
#39767=CARTESIAN_POINT ( 'NONE',  ( 16.69947034530964913, -2.312583065866261389, 2.590526750877053086 ) ) ;
#39800=CARTESIAN_POINT ( 'NONE',  ( 0.3656201545664388708, -2.182515578491310393, 9.881002359080277131 ) ) ;
#39802=EDGE_CURVE ( 'NONE', #22583, #48305, #50136, .T. ) ;
#39815=CARTESIAN_POINT ( 'NONE',  ( -26.18032376592659105, 21.95228666728381128, 7.455576670931136185 ) ) ;
#39826=ADVANCED_FACE ( 'NONE', ( #33330 ), #18769, .T. ) ;
#39832=CARTESIAN_POINT ( 'NONE',  ( 12.35406723005396046, -11.51001571518080624, 9.178419661560148768 ) ) ;
#39835=CARTESIAN_POINT ( 'NONE',  ( -23.26005729352344176, -44.90397804740339183, 7.906207997025717304 ) ) ;
#39846=CARTESIAN_POINT ( 'NONE',  ( 5.873104089934109595, 0.6060605173725697181, 9.586754400234156037 ) ) ;
#39852=ORIENTED_EDGE ( 'NONE', *, *, #10493, .F. ) ;
#39856=VERTEX_POINT ( 'NONE', #19164 ) ;
#39862=CARTESIAN_POINT ( 'NONE',  ( -18.67411147745623978, -27.51799019669813973, -3.760136334089591248 ) ) ;
#39864=CARTESIAN_POINT ( 'NONE',  ( 10.00000000000000000, 1.224646799147353256E-15, 10.00000000000000000 ) ) ;
#39870=CARTESIAN_POINT ( 'NONE',  ( 4.641001526964561918, 45.74479092860853058, -8.016098858316205167 ) ) ;
#39890=CARTESIAN_POINT ( 'NONE',  ( -9.760995290733800900, 2.173239732351794462, 9.646707543097347681 ) ) ;
#39900=FACE_OUTER_BOUND ( 'NONE', #29721, .T. ) ;
#39908=CARTESIAN_POINT ( 'NONE',  ( 22.69295089195473736, 45.31600496604706052, 7.455576670931136185 ) ) ;
#39913=CARTESIAN_POINT ( 'NONE',  ( 8.277096487746778308, -50.00000000000000000, 7.455576670931136185 ) ) ;
#39914=CARTESIAN_POINT ( 'NONE',  ( 29.18392875402930997, 17.44843138996603216, 7.906207997025717304 ) ) ;
#39915=SHAPE_REPRESENTATION ( 'fan', ( #45486 ), #38147 ) ;
#39917=ORIENTED_EDGE ( 'NONE', *, *, #50528, .T. ) ;
#39927=CARTESIAN_POINT ( 'NONE',  ( 6.174150299305392053, -50.00000000000000000, 8.807470649214879543 ) ) ;
#39929=ORIENTED_EDGE ( 'NONE', *, *, #23673, .F. ) ;
#39930=CARTESIAN_POINT ( 'NONE',  ( -0.3862712429686729343, -1.188820645368946050, 10.00000000000000000 ) ) ;
#39934=CARTESIAN_POINT ( 'NONE',  ( -2.322372356066614074, -2.286285436021753270, 9.799352050262461589 ) ) ;
#39939=CARTESIAN_POINT ( 'NONE',  ( -46.76852358249002606, 17.86468378716741512, -9.367992836599954742 ) ) ;
#39940=CARTESIAN_POINT ( 'NONE',  ( -0.1530804384065780344, 1.323112372394628977, 9.951893257059998277 ) ) ;
#39943=FACE_OUTER_BOUND ( 'NONE', #37570, .T. ) ;
#39950=EDGE_CURVE ( 'NONE', #6697, #43021, #11025, .T. ) ;
#39954=ORIENTED_EDGE ( 'NONE', *, *, #49304, .F. ) ;
#39956=CARTESIAN_POINT ( 'NONE',  ( 26.18032376592674737, -21.95228666728361233, 7.455576670931136185 ) ) ;
#39964=CARTESIAN_POINT ( 'NONE',  ( 0.3862712429686978033, -1.188820645368937834, -10.00000000000000000 ) ) ;
#39965=CARTESIAN_POINT ( 'NONE',  ( 1.962712821592840662, 1.022159834731142691, 9.881002359080275355 ) ) ;
#39975=CARTESIAN_POINT ( 'NONE',  ( 0.3896797354184660667, -1.262193838292004155, 9.943883492372872723 ) ) ;
#39979=CARTESIAN_POINT ( 'NONE',  ( 1.011271242968688311, -0.7347315653655855927, -10.00000000000000000 ) ) ;
#39986=CARTESIAN_POINT ( 'NONE',  ( -0.3896797354171960270, 1.262193838292709147, 9.943883492372847854 ) ) ;
#39990=EDGE_CURVE ( 'NONE', #6697, #11814, #47693, .T. ) ;
#39991=LINE ( 'NONE', #12514, #47064 ) ;
#40017=CARTESIAN_POINT ( 'NONE',  ( -32.00969891772112419, -38.54699130261795403, -8.917361510505369182 ) ) ;
#40019=CARTESIAN_POINT ( 'NONE',  ( -0.8282505383454070724, -1.889063466747028297, 9.894754715216727448 ) ) ;
#40020=ORIENTED_EDGE ( 'NONE', *, *, #35160, .T. ) ;
#40045=B_SPLINE_SURFACE_WITH_KNOTS ( 'NONE', 3, 3, ( 
 ( #40168, #4259, #24274, #5004 ),
 ( #35839, #5258, #36598, #39668 ),
 ( #48060, #20151, #16310, #43498 ),
 ( #47567, #12450, #44242, #39426 ) ),
 .UNSPECIFIED., .F., .F., .F.,
 ( 4, 4 ),
 ( 4, 4 ),
 ( 0.000000000000000000, 1.000000000000000000 ),
 ( 0.000000000000000000, 1.000000000000000000 ),
 .UNSPECIFIED. ) ;
#40048=CARTESIAN_POINT ( 'NONE',  ( -13.59579750444763668, 10.60877755095910935, 8.727788335465566760 ) ) ;
#40062=CARTESIAN_POINT ( 'NONE',  ( -33.16902712922616558, 37.70469005304312304, 1.847720168420772691 ) ) ;
#40067=EDGE_CURVE ( 'NONE', #43972, #17766, #26301, .T. ) ;
#40069=CARTESIAN_POINT ( 'NONE',  ( -0.8433491450857070193, 0.9182416014173486740, 9.981352469109932457 ) ) ;
#40088=CARTESIAN_POINT ( 'NONE',  ( 49.89397392339123627, -8.245536726716670373, 7.906207997025717304 ) ) ;
#40120=CARTESIAN_POINT ( 'NONE',  ( -44.99506233596265048, -23.32283626942287569, 7.455576670931136185 ) ) ;
#40125=CARTESIAN_POINT ( 'NONE',  ( 1.066995270233474624, -33.23888904628638841, -3.760136334089591248 ) ) ;
#40126=EDGE_LOOP ( 'NONE', ( #30476, #44706, #23438 ) ) ;
#40143=CARTESIAN_POINT ( 'NONE',  ( -48.98697415750977768, -11.03699497439218646, -8.016098858316199838 ) ) ;
#40147=CARTESIAN_POINT ( 'NONE',  ( -0.4154044336478688315, 2.070917815000994811, 9.890170120223993777 ) ) ;
#40148=CARTESIAN_POINT ( 'NONE',  ( -0.3862712429686729343, -1.188820645368946050, 10.00000000000000000 ) ) ;
#40149=EDGE_CURVE ( 'NONE', #30248, #18098, #42188, .T. ) ;
#40159=B_SPLINE_CURVE_WITH_KNOTS ( 'NONE', 3,
 ( #31240, #7891, #8141, #7376 ),
 .UNSPECIFIED., .F., .F.,
 ( 4, 4 ),
 ( 0.001152428489661405653, 0.001623376834729593982 ),
 .UNSPECIFIED. ) ;
#40168=CARTESIAN_POINT ( 'NONE',  ( -22.69295089195507487, -45.31600496604688999, 7.455576670931136185 ) ) ;
#40172=ORIENTED_EDGE ( 'NONE', *, *, #33777, .T. ) ;
#40186=CARTESIAN_POINT ( 'NONE',  ( -44.99506233596265048, -23.32283626942287569, 7.455576670931136185 ) ) ;
#40188=CARTESIAN_POINT ( 'NONE',  ( -1.782521105131510186, 0.3635605703594341209, 9.903764339332088440 ) ) ;
#40196=CARTESIAN_POINT ( 'NONE',  ( -24.39427009666018265, -44.07992421011638129, 8.807470649214879543 ) ) ;
#40203=ORIENTED_EDGE ( 'NONE', *, *, #47570, .F. ) ;
#40205=FACE_OUTER_BOUND ( 'NONE', #4100, .T. ) ;
#40217=CARTESIAN_POINT ( 'NONE',  ( -1.080000014127418639, -0.7606467978654640749, 9.943883492372872723 ) ) ;
#40220=CARTESIAN_POINT ( 'NONE',  ( 14.48769039275578407, 30.44468701195595983, 8.807470649214879543 ) ) ;
#40224=CARTESIAN_POINT ( 'NONE',  ( 7.749480817862238524, 14.85497772329518895, 9.403735324607438884 ) ) ;
#40243=CARTESIAN_POINT ( 'NONE',  ( -27.73884755486766096, 25.23502201956265978, 7.697694107796191787 ) ) ;
#40250=DIRECTION ( 'NONE',  ( -0.000000000000000000, 0.000000000000000000, -1.000000000000000000 ) ) ;
#40258=CARTESIAN_POINT ( 'NONE',  ( -32.57680531928949108, -38.13496438397444877, -8.466730184410787174 ) ) ;
#40266=ORIENTED_EDGE ( 'NONE', *, *, #47865, .T. ) ;
#40270=ORIENTED_EDGE ( 'NONE', *, *, #9250, .F. ) ;
#40287=ORIENTED_EDGE ( 'NONE', *, *, #30414, .T. ) ;
#40288=ORIENTED_EDGE ( 'NONE', *, *, #14123, .F. ) ;
#40294=CARTESIAN_POINT ( 'NONE',  ( 5.888214538810389698, 16.20866436362417673, 8.727788335465566760 ) ) ;
#40295=VERTEX_POINT ( 'NONE', #2110 ) ;
#40317=CARTESIAN_POINT ( 'NONE',  ( -0.05286079371165668117, 1.230216489825517234, 9.975326647350888365 ) ) ;
#40331=VERTEX_POINT ( 'NONE', #24958 ) ;
#40340=ORIENTED_EDGE ( 'NONE', *, *, #38200, .T. ) ;
#40341=CARTESIAN_POINT ( 'NONE',  ( -0.2553898474591131396, 1.933866572595240640, 9.896373613412551506 ) ) ;
#40352=B_SPLINE_SURFACE_WITH_KNOTS ( 'NONE', 3, 3, ( 
 ( #5028, #41451, #18336, #9646 ),
 ( #21191, #49101, #40705, #17343 ),
 ( #37626, #29649, #21691, #1952 ),
 ( #2694, #14241, #2206, #22208 ) ),
 .UNSPECIFIED., .F., .F., .F.,
 ( 4, 4 ),
 ( 4, 4 ),
 ( 0.000000000000000000, 1.000000000000000000 ),
 ( 0.000000000000000000, 1.000000000000000000 ),
 .UNSPECIFIED. ) ;
#40353=CARTESIAN_POINT ( 'NONE',  ( 1.249999999999999778, -0.000000000000000000, -10.00000000000000000 ) ) ;
#40354=CARTESIAN_POINT ( 'NONE',  ( -49.46074318306826001, 9.578883844007169301, 8.807470649214879543 ) ) ;
#40367=CARTESIAN_POINT ( 'NONE',  ( -48.33712804702535948, -13.03701565032741527, -9.367992836599954742 ) ) ;
#40370=CARTESIAN_POINT ( 'NONE',  ( -6.875132362119187768, 33.14667368551891258, 8.356839323120299312 ) ) ;
#40371=CARTESIAN_POINT ( 'NONE',  ( 1.377509002708426689, -0.6027468487254984408, 9.927319414211227766 ) ) ;
#40378=CARTESIAN_POINT ( 'NONE',  ( -0.3370904143228927730, -0.2449105217885335917, 10.00000000000000000 ) ) ;
#40379=VERTEX_POINT ( 'NONE', #22105 ) ;
#40397=VERTEX_POINT ( 'NONE', #37530 ) ;
#40398=CARTESIAN_POINT ( 'NONE',  ( 2.961022939495062900, -16.59676755884084187, 2.590526750877053086 ) ) ;
#40400=CARTESIAN_POINT ( 'NONE',  ( -45.64490844644706868, -21.32281559348764333, 8.807470649214879543 ) ) ;
#40405=CARTESIAN_POINT ( 'NONE',  ( 13.35436367797824353, 31.26996044524050333, 7.906207997025717304 ) ) ;
#40409=CARTESIAN_POINT ( 'NONE',  ( 8.032723559237163968, -41.13077784380362090, 7.544061037322996377 ) ) ;
#40414=B_SPLINE_CURVE_WITH_KNOTS ( 'NONE', 3,
 ( #44622, #21302, #1562, #25924 ),
 .UNSPECIFIED., .F., .F.,
 ( 4, 4 ),
 ( 0.0006669682284780709776, 0.0007799402130919361490 ),
 .UNSPECIFIED. ) ;
#40421=EDGE_LOOP ( 'NONE', ( #22834, #48002, #3199 ) ) ;
#40429=CARTESIAN_POINT ( 'NONE',  ( -46.11867747200562206, 19.86470446310265459, -8.016098858316205167 ) ) ;
#40434=ADVANCED_FACE ( 'NONE', ( #45677 ), #44521, .T. ) ;
#40438=CARTESIAN_POINT ( 'NONE',  ( 34.08355720199905647, -2.371364769369109116, 7.455576670931136185 ) ) ;
#40439=CARTESIAN_POINT ( 'NONE',  ( -25.63461350838931807, 43.17876197216396861, -8.016098858316199838 ) ) ;
#40447=CARTESIAN_POINT ( 'NONE',  ( 0.2827943264366570286, -6.852167361307233584, 9.753789706659947711 ) ) ;
#40451=CARTESIAN_POINT ( 'NONE',  ( -13.35436367797847801, -31.26996044524040741, 7.906207997025717304 ) ) ;
#40460=B_SPLINE_SURFACE_WITH_KNOTS ( 'NONE', 3, 3, ( 
 ( #6969, #30080, #19514, #15176 ),
 ( #3107, #26222, #10816, #38298 ),
 ( #41867, #23381, #22867, #50270 ),
 ( #7226, #7490, #39053, #18754 ) ),
 .UNSPECIFIED., .F., .F., .F.,
 ( 4, 4 ),
 ( 4, 4 ),
 ( 0.000000000000000000, 1.000000000000000000 ),
 ( 0.000000000000000000, 1.000000000000000000 ),
 .UNSPECIFIED. ) ;
#40461=ORIENTED_EDGE ( 'NONE', *, *, #45961, .F. ) ;
#40468=ORIENTED_EDGE ( 'NONE', *, *, #4965, .T. ) ;
#40470=CARTESIAN_POINT ( 'NONE',  ( 1.738880908827871830, 0.9455076376092198531, 9.897807938190494426 ) ) ;
#40475=CARTESIAN_POINT ( 'NONE',  ( -12.78770032058971395, -31.68259716188267916, 7.455576670931136185 ) ) ;
#40494=FACE_OUTER_BOUND ( 'NONE', #25189, .T. ) ;
#40497=CARTESIAN_POINT ( 'NONE',  ( 48.98697415750968531, 11.03699497439252752, -8.016098858316199838 ) ) ;
#40503=ADVANCED_FACE ( 'NONE', ( #38 ), #21197, .T. ) ;
#40505=CARTESIAN_POINT ( 'NONE',  ( -0.5109188679997889171, -1.175605252300625514, 9.967237415621765351 ) ) ;
#40513=CARTESIAN_POINT ( 'NONE',  ( 0.3370904143228959926, -0.2449105217885284291, -10.00000000000000000 ) ) ;
#40516=CARTESIAN_POINT ( 'NONE',  ( 1.456734136748010888, -2.915208416223516785, 9.799352050262463365 ) ) ;
#40523=CARTESIAN_POINT ( 'NONE',  ( -23.26005729352344176, -44.90397804740339183, 7.906207997025717304 ) ) ;
#40526=CARTESIAN_POINT ( 'NONE',  ( 1.250000000000000222, 0.000000000000000000, 10.00000000000000000 ) ) ;
#40539=CARTESIAN_POINT ( 'NONE',  ( -1.096405125442160067, -0.6872074048085232700, 9.947020512645400103 ) ) ;
#40544=CARTESIAN_POINT ( 'NONE',  ( 8.831420117243668599, 14.12636088103192655, -3.546734833711462365 ) ) ;
#40558=CARTESIAN_POINT ( 'NONE',  ( -15.45175104485246820, 6.222373774239106758, -2.870787844569587133 ) ) ;
#40559=EDGE_LOOP ( 'NONE', ( #13809, #21035, #33243, #47103 ) ) ;
#40563=CARTESIAN_POINT ( 'NONE',  ( -28.96803024440907137, -18.11533787072017176, 7.455576670931136185 ) ) ;
#40566=CARTESIAN_POINT ( 'NONE',  ( -0.1425549192113998442, 1.238581250503548059, 9.981352469109934233 ) ) ;
#40572=CARTESIAN_POINT ( 'NONE',  ( 6.174150299305392053, -50.00000000000000000, 8.807470649214879543 ) ) ;
#40584=CARTESIAN_POINT ( 'NONE',  ( 0.7606162131530698201, -1.296876929034913140, 9.953784399990620813 ) ) ;
#40585=CARTESIAN_POINT ( 'NONE',  ( 33.64889274059390090, -3.704246042440748621, 8.356839323120299312 ) ) ;
#40587=CARTESIAN_POINT ( 'NONE',  ( 28.96803024440893992, 18.11533787072037072, 7.455576670931136185 ) ) ;
#40589=EDGE_CURVE ( 'NONE', #40610, #17293, #50688, .T. ) ;
#40595=EDGE_CURVE ( 'NONE', #33462, #10853, #11843, .T. ) ;
#40601=ADVANCED_FACE ( 'NONE', ( #5127 ), #38047, .T. ) ;
#40610=VERTEX_POINT ( 'NONE', #47942 ) ;
#40614=FACE_OUTER_BOUND ( 'NONE', #5359, .T. ) ;
#40631=ORIENTED_EDGE ( 'NONE', *, *, #23096, .T. ) ;
#40637=CARTESIAN_POINT ( 'NONE',  ( -0.6667118921986187052, 1.119934874655410972, 9.961915419665738014 ) ) ;
#40644=EDGE_CURVE ( 'NONE', #7897, #50205, #26200, .T. ) ;
#40647=CARTESIAN_POINT ( 'NONE',  ( 23.26005729352310425, 44.90397804740356236, 7.906207997025717304 ) ) ;
#40655=CARTESIAN_POINT ( 'NONE',  ( -5.542614707656985829, -8.340505786370593810, 6.429802539306485265 ) ) ;
#40675=VERTEX_POINT ( 'NONE', #48936 ) ;
#40680=CARTESIAN_POINT ( 'NONE',  ( 49.46074318306830975, -9.578883844006833570, 8.807470649214879543 ) ) ;
#40693=CARTESIAN_POINT ( 'NONE',  ( 16.16402646813543242, -4.033894069732437693, -3.546734833711462365 ) ) ;
#40695=CARTESIAN_POINT ( 'NONE',  ( 37.50000000000000000, 4.592425496802574367E-15, 10.00000000000000000 ) ) ;
#40698=AXIS2_PLACEMENT_3D ( 'NONE', #16377, #43313, #35147 ) ;
#40701=CARTESIAN_POINT ( 'NONE',  ( 0.9390173899407876501, 1.130417317737878458, 9.958264684458711713 ) ) ;
#40705=CARTESIAN_POINT ( 'NONE',  ( -16.15814872688569181, -4.048305257546697788, -2.870787844569587133 ) ) ;
#40712=CARTESIAN_POINT ( 'NONE',  ( -49.67735855322972327, 8.912210285362091255, 8.356839323120299312 ) ) ;
#40728=VERTEX_POINT ( 'NONE', #10250 ) ;
#40736=CARTESIAN_POINT ( 'NONE',  ( 0.2778388845795309314, -1.251314014313100520, 9.976582533991681601 ) ) ;
#40738=B_SPLINE_CURVE_WITH_KNOTS ( 'NONE', 3,
 ( #39241, #733, #4586, #34889 ),
 .UNSPECIFIED., .F., .F.,
 ( 4, 4 ),
 ( 0.000000000000000000, 0.002217981418809652702 ),
 .UNSPECIFIED. ) ;
#40749=FACE_OUTER_BOUND ( 'NONE', #21796, .T. ) ;
#40764=CARTESIAN_POINT ( 'NONE',  ( 18.38319608353691947, -32.68498281710168385, -8.192531242611265085 ) ) ;
#40768=B_SPLINE_SURFACE_WITH_KNOTS ( 'NONE', 3, 3, ( 
 ( #27372, #46061, #7885, #23530 ),
 ( #15328, #30980, #27120, #43005 ),
 ( #38425, #4020, #19667, #14544 ),
 ( #30199, #6857, #10955, #20170 ) ),
 .UNSPECIFIED., .F., .F., .F.,
 ( 4, 4 ),
 ( 4, 4 ),
 ( 0.000000000000000000, 1.000000000000000000 ),
 ( 0.000000000000000000, 1.000000000000000000 ),
 .UNSPECIFIED. ) ;
#40775=CARTESIAN_POINT ( 'NONE',  ( 14.76429217231961566, 8.192625680377691566, 9.178419661560148768 ) ) ;
#40777=CARTESIAN_POINT ( 'NONE',  ( -0.9599924130074112272, 0.8495346730527952861, 9.948547179989619238 ) ) ;
#40779=EDGE_LOOP ( 'NONE', ( #46102, #11795, #31961, #26898, #10472 ) ) ;
#40782=B_SPLINE_CURVE_WITH_KNOTS ( 'NONE', 3,
 ( #29730, #10724, #6374, #34102 ),
 .UNSPECIFIED., .F., .F.,
 ( 4, 4 ),
 ( 3.789440921763008408E-16, 0.009762429737398312102 ),
 .UNSPECIFIED. ) ;
#40788=ORIENTED_EDGE ( 'NONE', *, *, #41286, .T. ) ;
#40790=ADVANCED_FACE ( 'NONE', ( #6646 ), #37224, .T. ) ;
#40793=CARTESIAN_POINT ( 'NONE',  ( -25.61277432017861955, 22.36370378792854297, 7.906207997025717304 ) ) ;
#40794=CARTESIAN_POINT ( 'NONE',  ( 1.250000000000000222, 0.000000000000000000, 3.333333333333333481 ) ) ;
#40795=CARTESIAN_POINT ( 'NONE',  ( 21.61731705588930907, 25.43568671410602278, -9.367992836599954742 ) ) ;
#40807=CARTESIAN_POINT ( 'NONE',  ( 0.3862712429686894766, -1.188820645368940276, 10.00000000000000000 ) ) ;
#40830=CARTESIAN_POINT ( 'NONE',  ( -0.3862712429686977478, 1.188820645368937390, 10.00000000000000000 ) ) ;
#40843=CARTESIAN_POINT ( 'NONE',  ( -48.34672127938071640, 13.00749071703899773, 3.199614146704519602 ) ) ;
#40849=ORIENTED_EDGE ( 'NONE', *, *, #18699, .T. ) ;
#40853=EDGE_CURVE ( 'NONE', #1381, #45083, #24399, .T. ) ;
#40857=CARTESIAN_POINT ( 'NONE',  ( -1.249999999999999778, 0.000000000000000000, -3.333333333333333481 ) ) ;
#40863=CARTESIAN_POINT ( 'NONE',  ( 34.91952936320839740, -13.67027684621004546, -9.422646554964178023 ) ) ;
#40869=B_SPLINE_SURFACE_WITH_KNOTS ( 'NONE', 3, 3, ( 
 ( #46537, #39152, #27336, #3980 ),
 ( #20136, #648, #16047, #22964 ),
 ( #148, #16297, #47042, #11945 ),
 ( #27603, #43232, #19113, #12191 ) ),
 .UNSPECIFIED., .F., .F., .F.,
 ( 4, 4 ),
 ( 4, 4 ),
 ( 0.000000000000000000, 1.000000000000000000 ),
 ( 0.000000000000000000, 1.000000000000000000 ),
 .UNSPECIFIED. ) ;
#40876=CARTESIAN_POINT ( 'NONE',  ( -0.7606162131530730397, 1.296876929034918691, 9.953784399990622589 ) ) ;
#40881=CARTESIAN_POINT ( 'NONE',  ( 1.468624871022813139, 0.3222420739259631572, 9.936141075690079205 ) ) ;
#40883=CARTESIAN_POINT ( 'NONE',  ( 8.640097307817493189, -14.29292567250784174, -9.458680755252684591 ) ) ;
#40887=CARTESIAN_POINT ( 'NONE',  ( 46.11867747200574996, -19.86470446310233484, -8.016098858316205167 ) ) ;
#40889=CARTESIAN_POINT ( 'NONE',  ( -46.75893035013464072, -17.89420872045582200, 3.199614146704519602 ) ) ;
#40892=CARTESIAN_POINT ( 'NONE',  ( 33.86622497129647513, -3.037805405904928868, 7.906207997025717304 ) ) ;
#40895=ORIENTED_EDGE ( 'NONE', *, *, #18294, .F. ) ;
#40896=EDGE_CURVE ( 'NONE', #18198, #33857, #12267, .T. ) ;
#40900=ADVANCED_FACE ( 'NONE', ( #23302 ), #2788, .T. ) ;
#40918=CARTESIAN_POINT ( 'NONE',  ( 44.99506233596247995, 23.32283626942318833, 7.455576670931136185 ) ) ;
#40920=ORIENTED_EDGE ( 'NONE', *, *, #37510, .T. ) ;
#40944=B_SPLINE_CURVE_WITH_KNOTS ( 'NONE', 3,
 ( #2870, #30101, #6994, #34983 ),
 .UNSPECIFIED., .F., .F.,
 ( 4, 4 ),
 ( 0.9890644561682331304, 1.000000000000000000 ),
 .UNSPECIFIED. ) ;
#40945=EDGE_CURVE ( 'NONE', #1639, #28100, #4116, .T. ) ;
#40946=CARTESIAN_POINT ( 'NONE',  ( -1.250000000000000222, 0.000000000000000000, 10.00000000000000000 ) ) ;
#40949=FACE_OUTER_BOUND ( 'NONE', #12141, .T. ) ;
#40950=ORIENTED_EDGE ( 'NONE', *, *, #32103, .F. ) ;
#40951=CARTESIAN_POINT ( 'NONE',  ( -13.92102703536724384, -30.85732372859812500, 8.356839323120299312 ) ) ;
#40954=CARTESIAN_POINT ( 'NONE',  ( 48.33712804702525290, 13.03701565032775456, -9.367992836599951190 ) ) ;
#40957=CARTESIAN_POINT ( 'NONE',  ( -1.578643388466005160, 1.550786058692512182, 9.881002359080275355 ) ) ;
#40966=CARTESIAN_POINT ( 'NONE',  ( 4.763548243873389154, -16.57409059453848599, 8.727788335465566760 ) ) ;
#40967=CARTESIAN_POINT ( 'NONE',  ( -0.7849184246622071814, 1.242376769534369041, 9.958264684458713489 ) ) ;
#40979=ORIENTED_EDGE ( 'NONE', *, *, #17986, .T. ) ;
#40983=EDGE_CURVE ( 'NONE', #5197, #8231, #39991, .T. ) ;
#40986=DIRECTION ( 'NONE',  ( -0.4374820812098816347, -0.3178493372392748872, 0.8411784753765542133 ) ) ;
#40995=CARTESIAN_POINT ( 'NONE',  ( -13.59579750444763668, 10.60877755095910935, 8.727788335465566760 ) ) ;
#41000=ORIENTED_EDGE ( 'NONE', *, *, #42214, .F. ) ;
#41018=ORIENTED_EDGE ( 'NONE', *, *, #130, .T. ) ;
#41021=VERTEX_POINT ( 'NONE', #45301 ) ;
#41027=CARTESIAN_POINT ( 'NONE',  ( 20.21530556545302559, -31.58467066308217497, -9.422646554964174470 ) ) ;
#41038=ORIENTED_EDGE ( 'NONE', *, *, #9656, .T. ) ;
#41040=VERTEX_POINT ( 'NONE', #49389 ) ;
#41041=CARTESIAN_POINT ( 'NONE',  ( 0.000000000000000000, 0.000000000000000000, 0.000000000000000000 ) ) ;
#41047=CARTESIAN_POINT ( 'NONE',  ( -6.174150299305392053, 33.14591993373988998, 8.807470649214879543 ) ) ;
#41052=CARTESIAN_POINT ( 'NONE',  ( -0.9342132981372995859, -1.950058179216137999, 9.882710035074772748 ) ) ;
#41053=CARTESIAN_POINT ( 'NONE',  ( -48.33712804702535948, -13.03701565032741527, -9.367992836599954742 ) ) ;
#41056=FACE_OUTER_BOUND ( 'NONE', #6432, .T. ) ;
#41059=CARTESIAN_POINT ( 'NONE',  ( 0.4401267517947335395, -2.015194695084121079, 9.889206917020302967 ) ) ;
#41064=CARTESIAN_POINT ( 'NONE',  ( -4.339432828817248122, -37.24807810779213213, -8.192531242611266862 ) ) ;
#41067=EDGE_CURVE ( 'NONE', #36298, #44983, #21840, .T. ) ;
#41072=CARTESIAN_POINT ( 'NONE',  ( -3.229232847726260403, 16.57333684275945629, 9.178419661560148768 ) ) ;
#41076=VECTOR ( 'NONE', #25601, 1000.000000000000000 ) ;
#41080=B_SPLINE_CURVE_WITH_KNOTS ( 'NONE', 3,
 ( #27575, #43210, #38874, #26548 ),
 .UNSPECIFIED., .F., .F.,
 ( 4, 4 ),
 ( 0.7491799374948676649, 1.000000000000000000 ),
 .UNSPECIFIED. ) ;
#41082=CARTESIAN_POINT ( 'NONE',  ( -21.20039782019574659, 30.97601161206942066, -2.490396854064190979 ) ) ;
#41089=ORIENTED_EDGE ( 'NONE', *, *, #14123, .T. ) ;
#41105=ORIENTED_EDGE ( 'NONE', *, *, #35058, .T. ) ;
#41108=CARTESIAN_POINT ( 'NONE',  ( -0.9602803029231570253, 0.8490247040095960651, 9.976582533991679824 ) ) ;
#41109=CARTESIAN_POINT ( 'NONE',  ( 33.43156050989131955, -4.370686678976570150, 8.807470649214879543 ) ) ;
#41114=ORIENTED_EDGE ( 'NONE', *, *, #21130, .T. ) ;
#41132=CARTESIAN_POINT ( 'NONE',  ( 0.3862712429686894766, -1.188820645368940276, 10.00000000000000000 ) ) ;
#41136=CARTESIAN_POINT ( 'NONE',  ( 1.011271242968694084, -0.7347315653655782652, -10.00000000000000000 ) ) ;
#41138=DIRECTION ( 'NONE',  ( -1.000000000000000000, 0.000000000000000000, 0.000000000000000000 ) ) ;
#41167=CARTESIAN_POINT ( 'NONE',  ( -0.1265591857321690383, -1.213367045380180809, 9.963925895596192461 ) ) ;
#41176=B_SPLINE_SURFACE_WITH_KNOTS ( 'NONE', 3, 3, ( 
 ( #28941, #48641, #40995, #26094 ),
 ( #21742, #17642, #49403, #36930 ),
 ( #29203, #44552, #44818, #45063 ),
 ( #37924, #18387, #33313, #33560 ) ),
 .UNSPECIFIED., .F., .F., .F.,
 ( 4, 4 ),
 ( 4, 4 ),
 ( 0.000000000000000000, 1.000000000000000000 ),
 ( 0.000000000000000000, 1.000000000000000000 ),
 .UNSPECIFIED. ) ;
#41185=ADVANCED_FACE ( 'NONE', ( #41227 ), #3193, .T. ) ;
#41191=CARTESIAN_POINT ( 'NONE',  ( -1.540662627795934769, 1.371465786296043765, 9.894754715216725671 ) ) ;
#41210=CARTESIAN_POINT ( 'NONE',  ( -1.158497635116737312, 16.61944452314319420, -3.546734833711462365 ) ) ;
#41213=EDGE_CURVE ( 'NONE', #1381, #32520, #7608, .T. ) ;
#41227=FACE_OUTER_BOUND ( 'NONE', #30962, .T. ) ;
#41229=CARTESIAN_POINT ( 'NONE',  ( 2.052549611693792464, -0.2039603569406628347, 9.894754715216725671 ) ) ;
#41230=CARTESIAN_POINT ( 'NONE',  ( 48.98697415750967821, 11.03699497439252220, -8.016098858316205167 ) ) ;
#41241=ADVANCED_FACE ( 'NONE', ( #23517 ), #39176, .F. ) ;
#41258=B_SPLINE_CURVE_WITH_KNOTS ( 'NONE', 3,
 ( #44938, #2860, #21886, #25990 ),
 .UNSPECIFIED., .F., .F.,
 ( 4, 4 ),
 ( 0.000000000000000000, 0.002368422649471284714 ),
 .UNSPECIFIED. ) ;
#41263=CARTESIAN_POINT ( 'NONE',  ( -7.129058724845069861, -15.30620660340479766, 9.178419661560148768 ) ) ;
#41272=B_SPLINE_CURVE_WITH_KNOTS ( 'NONE', 3,
 ( #9604, #48555, #25010, #48049 ),
 .UNSPECIFIED., .F., .F.,
 ( 4, 4 ),
 ( 9.305432711149857983E-16, 0.0004154657329515702127 ),
 .UNSPECIFIED. ) ;
#41277=ADVANCED_FACE ( 'NONE', ( #5265 ), #29401, .T. ) ;
#41278=ORIENTED_EDGE ( 'NONE', *, *, #30414, .F. ) ;
#41286=EDGE_CURVE ( 'NONE', #49869, #24077, #20401, .T. ) ;
#41288=B_SPLINE_SURFACE_WITH_KNOTS ( 'NONE', 3, 3, ( 
 ( #38310, #18768, #19019, #34448 ),
 ( #56, #27503, #34708, #39065 ),
 ( #14935, #11852, #11083, #30590 ),
 ( #26743, #19526, #35214, #13099 ) ),
 .UNSPECIFIED., .F., .F., .F.,
 ( 4, 4 ),
 ( 4, 4 ),
 ( 0.000000000000000000, 1.000000000000000000 ),
 ( 0.000000000000000000, 1.000000000000000000 ),
 .UNSPECIFIED. ) ;
#41290=EDGE_CURVE ( 'NONE', #19053, #42239, #41459, .T. ) ;
#41292=CARTESIAN_POINT ( 'NONE',  ( 1.035950918207909632, 50.00000000000000711, -2.408242355805840784 ) ) ;
#41298=VERTEX_POINT ( 'NONE', #927 ) ;
#41308=AXIS2_PLACEMENT_3D ( 'NONE', #25954, #22594, #30553 ) ;
#41312=ORIENTED_EDGE ( 'NONE', *, *, #47152, .F. ) ;
#41317=CARTESIAN_POINT ( 'NONE',  ( -30.12518629743573584, -14.70074613238887551, 1.847720168420772691 ) ) ;
#41322=B_SPLINE_CURVE_WITH_KNOTS ( 'NONE', 3,
 ( #18736, #33416, #18495, #45919 ),
 .UNSPECIFIED., .F., .F.,
 ( 4, 4 ),
 ( 0.000000000000000000, 0.0001252128669263171442 ),
 .UNSPECIFIED. ) ;
#41325=ORIENTED_EDGE ( 'NONE', *, *, #6572, .T. ) ;
#41340=CARTESIAN_POINT ( 'NONE',  ( 0.03371980368970583369, 1.221991649883343412, 9.987567862361069970 ) ) ;
#41346=ORIENTED_EDGE ( 'NONE', *, *, #42799, .T. ) ;
#41366=CARTESIAN_POINT ( 'NONE',  ( 9.645054515263739248, -2.693981805359395576, 6.429802539306495035 ) ) ;
#41368=CARTESIAN_POINT ( 'NONE',  ( 0.3862712429686815385, 1.188820645368943385, 9.972675548442461846 ) ) ;
#41392=EDGE_CURVE ( 'NONE', #10758, #6309, #43271, .T. ) ;
#41393=CARTESIAN_POINT ( 'NONE',  ( 14.48769039275578407, 30.44468701195595983, 8.807470649214879543 ) ) ;
#41402=CARTESIAN_POINT ( 'NONE',  ( 15.44803555374680393, 6.237487519713364570, -3.546734833711462365 ) ) ;
#41438=CARTESIAN_POINT ( 'NONE',  ( 27.73884755486784570, -25.23502201956245017, 7.697694107796188234 ) ) ;
#41448=CARTESIAN_POINT ( 'NONE',  ( 22.18397680750686263, 25.02304503454544360, -8.917361510505369182 ) ) ;
#41451=CARTESIAN_POINT ( 'NONE',  ( -33.08717642956897009, -5.870837526464928402, -8.016098858316199838 ) ) ;
#41453=CARTESIAN_POINT ( 'NONE',  ( -1.578643388466005160, 1.550786058692512182, 9.881002359080275355 ) ) ;
#41459=B_SPLINE_CURVE_WITH_KNOTS ( 'NONE', 3,
 ( #27873, #9367, #32227, #43503 ),
 .UNSPECIFIED., .F., .F.,
 ( 4, 4 ),
 ( 0.000000000000000000, 2.647279941188464684E-05 ),
 .UNSPECIFIED. ) ;
#41462=CARTESIAN_POINT ( 'NONE',  ( -1.437255894074058515, 3.713052624461494755, 6.606856988583542645E-16 ) ) ;
#41464=CARTESIAN_POINT ( 'NONE',  ( -11.73320209285699889, 11.96063479729179768, 9.403735324607438884 ) ) ;
#41482=CARTESIAN_POINT ( 'NONE',  ( -34.08355720199904226, 2.371364769369340042, 7.455576670931136185 ) ) ;
#41485=EDGE_CURVE ( 'NONE', #1912, #3402, #1665, .T. ) ;
#41493=CARTESIAN_POINT ( 'NONE',  ( 2.569099690548740877, -50.00000000000000711, 3.199614146704519602 ) ) ;
#41500=CARTESIAN_POINT ( 'NONE',  ( -25.63461350838931807, 43.17876197216396861, -8.016098858316199838 ) ) ;
#41506=CARTESIAN_POINT ( 'NONE',  ( -46.11867747200561496, 19.86470446310265103, -8.016098858316205167 ) ) ;
#41522=ORIENTED_EDGE ( 'NONE', *, *, #33986, .F. ) ;
#41525=FACE_OUTER_BOUND ( 'NONE', #33161, .T. ) ;
#41532=LINE ( 'NONE', #14579, #29709 ) ;
#41540=ORIENTED_EDGE ( 'NONE', *, *, #18398, .F. ) ;
#41543=ADVANCED_FACE ( 'NONE', ( #30392 ), #15491, .F. ) ;
#41549=CARTESIAN_POINT ( 'NONE',  ( 1.872530400643593440, -0.3103573527826896106, 9.900811091504552408 ) ) ;
#41559=CARTESIAN_POINT ( 'NONE',  ( -1.011271242968677875, -0.7347315653656004697, 3.333333333333333481 ) ) ;
#41561=CARTESIAN_POINT ( 'NONE',  ( 0.4400426740873927822, -2.015233077865103972, 9.886433018048071730 ) ) ;
#41565=CARTESIAN_POINT ( 'NONE',  ( 6.508636631827673824, 15.75743548351451295, 8.953103998512858652 ) ) ;
#41571=CARTESIAN_POINT ( 'NONE',  ( 3.525518878623022268, -1.771455639577098395, 6.494306196954933164 ) ) ;
#41574=DIRECTION ( 'NONE',  ( -1.000000000000000000, 0.000000000000000000, -0.000000000000000000 ) ) ;
#41576=ADVANCED_FACE ( 'NONE', ( #39368 ), #48184, .T. ) ;
#41583=CARTESIAN_POINT ( 'NONE',  ( 48.98697415750968531, 11.03699497439252752, -8.016098858316199838 ) ) ;
#41588=FACE_OUTER_BOUND ( 'NONE', #8962, .T. ) ;
#41590=EDGE_LOOP ( 'NONE', ( #37077, #18393, #39447, #26490, #10577, #27275, #41114, #3800, #23079, #45530, #34531, #19105, #26207, #40979 ) ) ;
#41594=B_SPLINE_CURVE_WITH_KNOTS ( 'NONE', 3,
 ( #29902, #6310, #10901, #21951 ),
 .UNSPECIFIED., .F., .F.,
 ( 4, 4 ),
 ( 0.7998230999345287140, 0.9869080488566185361 ),
 .UNSPECIFIED. ) ;
#41600=CARTESIAN_POINT ( 'NONE',  ( 1.553101183265239493, 0.2460239823947285576, 9.927288994922816912 ) ) ;
#41603=B_SPLINE_SURFACE_WITH_KNOTS ( 'NONE', 3, 3, ( 
 ( #40196, #2695, #3190, #49844 ),
 ( #2943, #14755, #50104, #45770 ),
 ( #37877, #14242, #37627, #29906 ),
 ( #34523, #46019, #18337, #13989 ) ),
 .UNSPECIFIED., .F., .F., .F.,
 ( 4, 4 ),
 ( 4, 4 ),
 ( 0.000000000000000000, 1.000000000000000000 ),
 ( 0.000000000000000000, 1.000000000000000000 ),
 .UNSPECIFIED. ) ;
#41616=VERTEX_POINT ( 'NONE', #617 ) ;
#41617=B_SPLINE_CURVE_WITH_KNOTS ( 'NONE', 3,
 ( #22313, #10511, #30790, #18704 ),
 .UNSPECIFIED., .F., .F.,
 ( 4, 4 ),
 ( 0.003717759948433960009, 0.009855840375009033635 ),
 .UNSPECIFIED. ) ;
#41618=CARTESIAN_POINT ( 'NONE',  ( 0.2131239213569732782, 1.205185050113728673, 9.966990753365131184 ) ) ;
#41630=CARTESIAN_POINT ( 'NONE',  ( 0.9647733827258516692, 1.276878621148359816, 9.919954374050675483 ) ) ;
#41631=EDGE_CURVE ( 'NONE', #566, #50289, #7207, .T. ) ;
#41645=FACE_OUTER_BOUND ( 'NONE', #16039, .T. ) ;
#41656=VERTEX_POINT ( 'NONE', #48513 ) ;
#41703=CARTESIAN_POINT ( 'NONE',  ( 11.54386348672365692, 12.18274641659816915, -9.233365092205394475 ) ) ;
#41705=CARTESIAN_POINT ( 'NONE',  ( 0.3862712429686894766, -1.188820645368940276, -3.333333333333333481 ) ) ;
#41706=CARTESIAN_POINT ( 'NONE',  ( -15.73090589902298042, -29.60029367929041655, 1.847720168420772691 ) ) ;
#41721=B_SPLINE_CURVE_WITH_KNOTS ( 'NONE', 3,
 ( #7008, #22401, #38073, #42652 ),
 .UNSPECIFIED., .F., .F.,
 ( 4, 4 ),
 ( 0.0006664118838822457149, 0.001081796195657078749 ),
 .UNSPECIFIED. ) ;
#41735=ORIENTED_EDGE ( 'NONE', *, *, #41631, .T. ) ;
#41737=CARTESIAN_POINT ( 'NONE',  ( -37.52258785160506704, -18.42740426802361142, 8.846626183609803462 ) ) ;
#41739=VECTOR ( 'NONE', #37070, 999.9999999999998863 ) ;
#41748=CARTESIAN_POINT ( 'NONE',  ( -2.052581215100349521, 0.2042358160481012597, 9.886433018048073507 ) ) ;
#41769=CARTESIAN_POINT ( 'NONE',  ( -33.01266944765060174, 5.813986777101691317, 1.847720168420772691 ) ) ;
#41770=CARTESIAN_POINT ( 'NONE',  ( 45.21167770612395742, 22.65616271077811206, 7.906207997025717304 ) ) ;
#41781=CARTESIAN_POINT ( 'NONE',  ( 0.9942667885118371407, -0.7728247605419453770, 9.974012008644013605 ) ) ;
#41785=CARTESIAN_POINT ( 'NONE',  ( -1.212058008859267177, -0.1697297676669723421, 9.966990753365127631 ) ) ;
#41811=CARTESIAN_POINT ( 'NONE',  ( -1.011271242968688533, 0.7347315653655859258, 3.333333333333333481 ) ) ;
#41812=B_SPLINE_CURVE_WITH_KNOTS ( 'NONE', 3,
 ( #8128, #4273, #8380, #35591 ),
 .UNSPECIFIED., .F., .F.,
 ( 4, 4 ),
 ( 8.673617379884035472E-19, 0.002466147708923230146 ),
 .UNSPECIFIED. ) ;
#41815=CARTESIAN_POINT ( 'NONE',  ( -6.174150299305392053, 50.00000000000000711, 8.807470649214879543 ) ) ;
#41818=ORIENTED_EDGE ( 'NONE', *, *, #45236, .T. ) ;
#41819=EDGE_CURVE ( 'NONE', #29160, #17906, #50493, .T. ) ;
#41823=CARTESIAN_POINT ( 'NONE',  ( -2.462075149652696027, 16.57295996686994499, 9.403735324607438884 ) ) ;
#41834=CARTESIAN_POINT ( 'NONE',  ( -1.332485441698227469, 1.351730126698055479, 9.900811091504548855 ) ) ;
#41845=EDGE_LOOP ( 'NONE', ( #45291, #197, #47694, #35323 ) ) ;
#41861=EDGE_CURVE ( 'NONE', #2423, #43021, #13808, .T. ) ;
#41864=EDGE_CURVE ( 'NONE', #36524, #31257, #40738, .T. ) ;
#41866=EDGE_CURVE ( 'NONE', #12977, #30605, #23650, .T. ) ;
#41867=CARTESIAN_POINT ( 'NONE',  ( 30.25247992116058526, -39.82368563463805344, -3.760136334089591248 ) ) ;
#41873=CARTESIAN_POINT ( 'NONE',  ( -23.82716369509181575, -44.49195112875988656, 8.356839323120299312 ) ) ;
#41882=EDGE_CURVE ( 'NONE', #47214, #24636, #13188, .T. ) ;
#41891=CARTESIAN_POINT ( 'NONE',  ( 9.260964247899975632, -13.84230907185609460, -9.683996418299976483 ) ) ;
#41924=CARTESIAN_POINT ( 'NONE',  ( -4.207128120815918256E-14, 3.058192377181588826E-14, 10.00000000000000000 ) ) ;
#41927=VERTEX_POINT ( 'NONE', #47889 ) ;
#41947=CARTESIAN_POINT ( 'NONE',  ( -4.207128120815918256E-14, 3.058192377181588826E-14, 10.00000000000000000 ) ) ;
#41955=CARTESIAN_POINT ( 'NONE',  ( 0.2459519479918564622, 1.553112592394157110, 9.927288994922816912 ) ) ;
#41956=CARTESIAN_POINT ( 'NONE',  ( 10.70590866674922204, -12.76446523155706814, -3.546734833711462365 ) ) ;
#41958=B_SPLINE_CURVE_WITH_KNOTS ( 'NONE', 3,
 ( #26866, #42503, #23005, #3497 ),
 .UNSPECIFIED., .F., .F.,
 ( 4, 4 ),
 ( 0.001152428489661398714, 0.001623376834730018555 ),
 .UNSPECIFIED. ) ;
#41965=FACE_OUTER_BOUND ( 'NONE', #19037, .T. ) ;
#41966=PLANE ( 'NONE',  #34783 ) ;
#41972=CARTESIAN_POINT ( 'NONE',  ( -1.222012661920452326, 0.2471648704738776681, 9.981352469109934233 ) ) ;
#41997=EDGE_LOOP ( 'NONE', ( #38001, #23860, #44846, #22434, #12194, #6577, #48427, #23091, #34739, #4846, #8415, #1613, #15906, #38309 ) ) ;
#42014=ORIENTED_EDGE ( 'NONE', *, *, #5204, .T. ) ;
#42024=ORIENTED_EDGE ( 'NONE', *, *, #12993, .T. ) ;
#42029=B_SPLINE_CURVE_WITH_KNOTS ( 'NONE', 3,
 ( #44605, #25910, #9734, #36976 ),
 .UNSPECIFIED., .F., .F.,
 ( 4, 4 ),
 ( 0.000000000000000000, 2.804146970186932266E-05 ),
 .UNSPECIFIED. ) ;
#42039=ORIENTED_EDGE ( 'NONE', *, *, #10646, .F. ) ;
#42042=LINE ( 'NONE', #6899, #45067 ) ;
#42057=CARTESIAN_POINT ( 'NONE',  ( -37.50000000000000000, 0.000000000000000000, 10.00000000000000000 ) ) ;
#42058=CARTESIAN_POINT ( 'NONE',  ( 15.80799809827373004, -29.65358618225706522, -8.016098858316199838 ) ) ;
#42063=CARTESIAN_POINT ( 'NONE',  ( -24.34206871062976063, -28.53454467304741371, -9.011255500499645521 ) ) ;
#42073=ORIENTED_EDGE ( 'NONE', *, *, #30574, .F. ) ;
#42078=DIRECTION ( 'NONE',  ( -0.1671032855531354999, 0.5142910309547730208, -0.8411784753765541023 ) ) ;
#42087=CARTESIAN_POINT ( 'NONE',  ( -0.6215990105957072132, 1.608617984725374983, 9.928159647716134018 ) ) ;
#42096=CARTESIAN_POINT ( 'NONE',  ( 0.3370904143228924954, 0.2449105217885333141, 10.00000000000000000 ) ) ;
#42101=CARTESIAN_POINT ( 'NONE',  ( -1.647520908219852975, 0.4432416309288251810, 9.912102921405043787 ) ) ;
#42102=CARTESIAN_POINT ( 'NONE',  ( -12.97493236725075683, 11.05939663307000664, 8.953103998512858652 ) ) ;
#42120=B_SPLINE_SURFACE_WITH_KNOTS ( 'NONE', 3, 3, ( 
 ( #20540, #20289, #20036, #35959 ),
 ( #15678, #16447, #12579, #27987 ),
 ( #1048, #28500, #8998, #44124 ),
 ( #24655, #35721, #31349, #46940 ) ),
 .UNSPECIFIED., .F., .F., .F.,
 ( 4, 4 ),
 ( 4, 4 ),
 ( 0.000000000000000000, 1.000000000000000000 ),
 ( 0.000000000000000000, 1.000000000000000000 ),
 .UNSPECIFIED. ) ;
#42121=CARTESIAN_POINT ( 'NONE',  ( 1.377636575563020438, -0.6021164824561170414, 9.953784399990622589 ) ) ;
#42137=CARTESIAN_POINT ( 'NONE',  ( 47.22310614333766665, 16.46562252335956344, -3.760136334089591248 ) ) ;
#42162=ADVANCED_FACE ( 'NONE', ( #17637 ), #21621, .T. ) ;
#42169=CARTESIAN_POINT ( 'NONE',  ( -0.1287570809895632329, 0.3962735484563137400, 10.00000000000000000 ) ) ;
#42170=ORIENTED_EDGE ( 'NONE', *, *, #10948, .T. ) ;
#42176=CARTESIAN_POINT ( 'NONE',  ( -0.3370904143228943828, -0.2449105217885308716, 10.00000000000000000 ) ) ;
#42186=CARTESIAN_POINT ( 'NONE',  ( 48.33712804702525290, 13.03701565032775456, -9.367992836599951190 ) ) ;
#42188=B_SPLINE_CURVE_WITH_KNOTS ( 'NONE', 3,
 ( #39164, #50643, #23230, #158 ),
 .UNSPECIFIED., .F., .F.,
 ( 4, 4 ),
 ( 0.001152428489661398280, 0.001623376834729610679 ),
 .UNSPECIFIED. ) ;
#42203=B_SPLINE_CURVE_WITH_KNOTS ( 'NONE', 3,
 ( #41748, #11223, #45575, #26360 ),
 .UNSPECIFIED., .F., .F.,
 ( 4, 4 ),
 ( 0.001937412222931639196, 0.003978261222106112445 ),
 .UNSPECIFIED. ) ;
#42205=EDGE_CURVE ( 'NONE', #45889, #20022, #8924, .T. ) ;
#42206=CARTESIAN_POINT ( 'NONE',  ( 0.8431937073474478073, -1.111389989013496837, 9.955131761384825140 ) ) ;
#42210=VERTEX_POINT ( 'NONE', #46566 ) ;
#42214=EDGE_CURVE ( 'NONE', #17359, #32354, #43811, .T. ) ;
#42215=VERTEX_POINT ( 'NONE', #39439 ) ;
#42216=ORIENTED_EDGE ( 'NONE', *, *, #13339, .T. ) ;
#42218=CARTESIAN_POINT ( 'NONE',  ( 0.4277546898748997295, 1.184419892831248378, 9.974012008644017158 ) ) ;
#42239=VERTEX_POINT ( 'NONE', #23524 ) ;
#42242=( NAMED_UNIT ( * ) PLANE_ANGLE_UNIT ( ) SI_UNIT ( $, .RADIAN. ) );
#42253=B_SPLINE_CURVE_WITH_KNOTS ( 'NONE', 3,
 ( #34386, #18960, #38251, #46396 ),
 .UNSPECIFIED., .F., .F.,
 ( 4, 4 ),
 ( 0.9811748202683390208, 0.9878904167554125593 ),
 .UNSPECIFIED. ) ;
#42258=CARTESIAN_POINT ( 'NONE',  ( 0.4166666666666664631, 0.000000000000000000, 10.00000000000000000 ) ) ;
#42259=CARTESIAN_POINT ( 'NONE',  ( 1.250000000000000222, 0.000000000000000000, 10.00000000000000000 ) ) ;
#42275=ORIENTED_EDGE ( 'NONE', *, *, #31574, .F. ) ;
#42285=ADVANCED_FACE ( 'NONE', ( #20674 ), #2375, .T. ) ;
#42286=CARTESIAN_POINT ( 'NONE',  ( 0.4154044336478738830, -2.070917815000952178, 9.890170120223997330 ) ) ;
#42289=CARTESIAN_POINT ( 'NONE',  ( -34.38161489319221431, 14.98878603239709939, -8.600750091277038933 ) ) ;
#42299=CARTESIAN_POINT ( 'NONE',  ( 10.69268279052430159, 12.77266927778462779, -2.870787844569587133 ) ) ;
#42300=CARTESIAN_POINT ( 'NONE',  ( 27.73884755486784570, -25.23502201956245017, 7.697694107796188234 ) ) ;
#42306=CARTESIAN_POINT ( 'NONE',  ( -7.576114424932982594, 33.14742743729794938, 7.906207997025717304 ) ) ;
#42309=CARTESIAN_POINT ( 'NONE',  ( -1.011271242968677875, -0.7347315653656004697, 3.333333333333333481 ) ) ;
#42310=CARTESIAN_POINT ( 'NONE',  ( 1.011271242968688311, -0.7347315653655855927, -10.00000000000000000 ) ) ;
#42319=FACE_OUTER_BOUND ( 'NONE', #43912, .T. ) ;
#42322=CARTESIAN_POINT ( 'NONE',  ( -7.576114424932982594, 33.14742743729794938, 7.906207997025717304 ) ) ;
#42323=CARTESIAN_POINT ( 'NONE',  ( -0.3910393408547386818, -3.877122853643371947, 9.741991644047244492 ) ) ;
#42341=EDGE_CURVE ( 'NONE', #30921, #12217, #24790, .T. ) ;
#42344=ORIENTED_EDGE ( 'NONE', *, *, #33212, .F. ) ;
#42350=VERTEX_POINT ( 'NONE', #1441 ) ;
#42352=B_SPLINE_CURVE_WITH_KNOTS ( 'NONE', 3,
 ( #35614, #1462, #39455, #43528 ),
 .UNSPECIFIED., .F., .F.,
 ( 4, 4 ),
 ( 3.806817868859629271E-16, 0.009762429722931321996 ),
 .UNSPECIFIED. ) ;
#42357=FACE_BOUND ( 'NONE', #27922, .T. ) ;
#42361=CARTESIAN_POINT ( 'NONE',  ( 50.11058929355270664, -7.578863168071591438, 7.455576670931136185 ) ) ;
#42381=CARTESIAN_POINT ( 'NONE',  ( 24.39427009665985224, 44.07992421011656603, 8.807470649214879543 ) ) ;
#42387=LINE ( 'NONE', #74, #32701 ) ;
#42391=LINE ( 'NONE', #18787, #15223 ) ;
#42396=DIRECTION ( 'NONE',  ( 0.000000000000000000, 0.000000000000000000, -1.000000000000000000 ) ) ;
#42405=EDGE_CURVE ( 'NONE', #43021, #16274, #937, .T. ) ;
#42410=CARTESIAN_POINT ( 'NONE',  ( 4.763548243873389154, -16.57409059453848599, 8.727788335465566760 ) ) ;
#42418=CARTESIAN_POINT ( 'NONE',  ( -1.419290803332700523, -0.2086015876293249582, 9.950105812514305370 ) ) ;
#42427=CARTESIAN_POINT ( 'NONE',  ( -17.23491422248386584, 0.5912720620001978844, 8.727788335465566760 ) ) ;
#42431=CARTESIAN_POINT ( 'NONE',  ( 0.7849184246612691540, -1.242376769536456704, 9.958264684458541183 ) ) ;
#42433=CARTESIAN_POINT ( 'NONE',  ( -30.67467450244469873, 28.55398182363574122, 7.544061037322996377 ) ) ;
#42434=EDGE_CURVE ( 'NONE', #49222, #29784, #16859, .T. ) ;
#42436=B_SPLINE_SURFACE_WITH_KNOTS ( 'NONE', 3, 3, ( 
 ( #18508, #46436, #49515, #34187 ),
 ( #23120, #49763, #30322, #42610 ),
 ( #10814, #26465, #42102, #6968 ),
 ( #22617, #18752, #34436, #46175 ) ),
 .UNSPECIFIED., .F., .F., .F.,
 ( 4, 4 ),
 ( 4, 4 ),
 ( 0.000000000000000000, 1.000000000000000000 ),
 ( 0.000000000000000000, 1.000000000000000000 ),
 .UNSPECIFIED. ) ;
#42446=EDGE_CURVE ( 'NONE', #47543, #48228, #49829, .T. ) ;
#42460=CARTESIAN_POINT ( 'NONE',  ( 0.3862712429686894766, -1.188820645368940276, 10.00000000000000000 ) ) ;
#42461=CARTESIAN_POINT ( 'NONE',  ( -4.763548243873389154, 16.57409059453848599, 8.727788335465566760 ) ) ;
#42492=EDGE_CURVE ( 'NONE', #48360, #15177, #43715, .T. ) ;
#42493=CARTESIAN_POINT ( 'NONE',  ( 14.48769039275578407, 30.44468701195595983, 8.807470649214879543 ) ) ;
#42498=CARTESIAN_POINT ( 'NONE',  ( 31.94178169330218964, -9.256608784833820991, -3.760136334089591248 ) ) ;
#42501=CARTESIAN_POINT ( 'NONE',  ( 13.59579750444771307, -10.60877755095900632, 8.727788335465566760 ) ) ;
#42503=CARTESIAN_POINT ( 'NONE',  ( 1.531049279420177101, 0.4659387722960993683, 9.919954280166514593 ) ) ;
#42506=EDGE_CURVE ( 'NONE', #29795, #31313, #5189, .T. ) ;
#42508=ORIENTED_EDGE ( 'NONE', *, *, #9028, .F. ) ;
#42511=CARTESIAN_POINT ( 'NONE',  ( -0.3443084382165982893, -1.609917862996312676, 9.927568724237803011 ) ) ;
#42513=CARTESIAN_POINT ( 'NONE',  ( -1.011271242968688533, 0.7347315653655859258, -3.333333333333333481 ) ) ;
#42528=ORIENTED_EDGE ( 'NONE', *, *, #48200, .T. ) ;
#42536=EDGE_CURVE ( 'NONE', #38752, #46997, #11286, .T. ) ;
#42543=CARTESIAN_POINT ( 'NONE',  ( 1.782521105131670724, -0.3635605703593869920, 9.903764339332079558 ) ) ;
#42559=CARTESIAN_POINT ( 'NONE',  ( 1.055760676366898521, 37.52140099356444836, -2.490396854064190535 ) ) ;
#42562=CARTESIAN_POINT ( 'NONE',  ( -1.011271242968688533, 0.7347315653655859258, -10.00000000000000000 ) ) ;
#42566=CARTESIAN_POINT ( 'NONE',  ( 31.94178169330218964, -9.256608784833820991, -3.760136334089591248 ) ) ;
#42570=CARTESIAN_POINT ( 'NONE',  ( -46.76852358249001895, 17.86468378716740801, -9.367992836599951190 ) ) ;
#42572=CARTESIAN_POINT ( 'NONE',  ( 33.64889274059390090, -3.704246042440748621, 8.356839323120299312 ) ) ;
#42577=ORIENTED_EDGE ( 'NONE', *, *, #33079, .F. ) ;
#42582=FACE_OUTER_BOUND ( 'NONE', #28330, .T. ) ;
#42602=CARTESIAN_POINT ( 'NONE',  ( -48.77035878734830732, -11.70366853303726273, -8.466730184410787174 ) ) ;
#42609=CARTESIAN_POINT ( 'NONE',  ( 33.01266944765062306, -5.813986777101467496, 1.847720168420772691 ) ) ;
#42610=CARTESIAN_POINT ( 'NONE',  ( 0.3370904143228947158, 0.2449105217885311492, 10.00000000000000000 ) ) ;
#42611=CARTESIAN_POINT ( 'NONE',  ( 0.3862712429686978033, -1.188820645368937834, 10.00000000000000000 ) ) ;
#42624=CARTESIAN_POINT ( 'NONE',  ( 37.27397286063867199, -4.111076158911552092, 7.697694107796188234 ) ) ;
#42629=VECTOR ( 'NONE', #29842, 1000.000000000000227 ) ;
#42633=CARTESIAN_POINT ( 'NONE',  ( 1.011271242968694084, -0.7347315653655782652, 10.00000000000000000 ) ) ;
#42646=FACE_OUTER_BOUND ( 'NONE', #1815, .T. ) ;
#42647=CARTESIAN_POINT ( 'NONE',  ( 27.33593271309472073, -41.94268121623323253, -9.367992836599951190 ) ) ;
#42650=VERTEX_POINT ( 'NONE', #1630 ) ;
#42652=CARTESIAN_POINT ( 'NONE',  ( 0.4426377647354858835, 1.666766018367784596, 9.928159647716132241 ) ) ;
#42654=ORIENTED_EDGE ( 'NONE', *, *, #11243, .T. ) ;
#42660=CARTESIAN_POINT ( 'NONE',  ( -31.44259251615275019, -38.95901822126145220, -9.367992836599954742 ) ) ;
#42662=CARTESIAN_POINT ( 'NONE',  ( 0.3862712429686894766, -1.188820645368940276, 10.00000000000000000 ) ) ;
#42676=B_SPLINE_CURVE_WITH_KNOTS ( 'NONE', 3,
 ( #50705, #31013, #42289, #34351 ),
 .UNSPECIFIED., .F., .F.,
 ( 4, 4 ),
 ( 2.453269466693398698E-18, 0.002466147708923231447 ),
 .UNSPECIFIED. ) ;
#42687=CARTESIAN_POINT ( 'NONE',  ( -2.052549611693787135, 0.2039603569406744088, 9.894754715216729224 ) ) ;
#42705=CARTESIAN_POINT ( 'NONE',  ( 7.576114424932982594, -50.00000000000000711, 7.906207997025717304 ) ) ;
#42731=LINE ( 'NONE', #7611, #14050 ) ;
#42736=CARTESIAN_POINT ( 'NONE',  ( 23.29043492822826167, -24.10797434788167948, 1.847720168420772691 ) ) ;
#42746=CARTESIAN_POINT ( 'NONE',  ( 3.087186397306452612, 2.514307945609885131, -2.642742795433417058E-16 ) ) ;
#42754=CARTESIAN_POINT ( 'NONE',  ( 9.907356528111447957, -1.358045148324435347, 0.000000000000000000 ) ) ;
#42756=CARTESIAN_POINT ( 'NONE',  ( 21.20039782019597396, -30.97601161206925724, -2.490396854064192755 ) ) ;
#42762=EDGE_LOOP ( 'NONE', ( #24195, #50271, #49382, #29295, #22137 ) ) ;
#42768=ORIENTED_EDGE ( 'NONE', *, *, #29267, .F. ) ;
#42775=CARTESIAN_POINT ( 'NONE',  ( 36.76598589393955052, 7.383243274241862331, -8.192531242611266862 ) ) ;
#42782=DIRECTION ( 'NONE',  ( 0.3090169943749447312, 0.9510565162951544194, 0.000000000000000000 ) ) ;
#42795=CARTESIAN_POINT ( 'NONE',  ( -45.21167770612412085, -22.65616271077779942, 7.906207997025717304 ) ) ;
#42799=EDGE_CURVE ( 'NONE', #6581, #35009, #26639, .T. ) ;
#42800=CARTESIAN_POINT ( 'NONE',  ( 0.8433491450857230065, -0.9182416014173362395, 9.981352469109934233 ) ) ;
#42809=ORIENTED_EDGE ( 'NONE', *, *, #22995, .T. ) ;
#42818=CARTESIAN_POINT ( 'NONE',  ( -29.18392875402943432, -17.44843138996582965, 7.906207997025717304 ) ) ;
#42820=CARTESIAN_POINT ( 'NONE',  ( 14.86945752723346637, 7.944783388879009145, 2.590526750877053086 ) ) ;
#42824=ADVANCED_FACE ( 'NONE', ( #2613 ), #37054, .F. ) ;
#42830=EDGE_CURVE ( 'NONE', #19115, #1912, #41258, .T. ) ;
#42836=B_SPLINE_CURVE_WITH_KNOTS ( 'NONE', 3,
 ( #48947, #13835, #10009, #25669 ),
 .UNSPECIFIED., .F., .F.,
 ( 4, 4 ),
 ( 0.001937412222931662181, 0.003978261222109142140 ),
 .UNSPECIFIED. ) ;
#42854=B_SPLINE_SURFACE_WITH_KNOTS ( 'NONE', 3, 3, ( 
 ( #19428, #11732, #7128, #43719 ),
 ( #8588, #897, #30469, #16538 ),
 ( #32191, #3254, #22767, #18906 ),
 ( #34581, #46342, #7385, #5986 ) ),
 .UNSPECIFIED., .F., .F., .F.,
 ( 4, 4 ),
 ( 4, 4 ),
 ( 0.000000000000000000, 1.000000000000000000 ),
 ( 0.000000000000000000, 1.000000000000000000 ),
 .UNSPECIFIED. ) ;
#42856=CARTESIAN_POINT ( 'NONE',  ( 0.9598058911017247619, 1.847159827636295937, 9.888808121373916293 ) ) ;
#42862=FACE_OUTER_BOUND ( 'NONE', #22382, .T. ) ;
#42868=CARTESIAN_POINT ( 'NONE',  ( -9.696760411816217839, -2.443938934554997999, 0.000000000000000000 ) ) ;
#42876=CARTESIAN_POINT ( 'NONE',  ( -16.69947034530963847, 2.312583065866374632, 2.590526750877053086 ) ) ;
#42884=CARTESIAN_POINT ( 'NONE',  ( -1.011271242968688533, 0.7347315653655859258, 10.00000000000000000 ) ) ;
#42887=CARTESIAN_POINT ( 'NONE',  ( -1.011271242968693862, 0.7347315653655780432, -10.00000000000000000 ) ) ;
#42891=EDGE_CURVE ( 'NONE', #30805, #3733, #38836, .T. ) ;
#42922=CARTESIAN_POINT ( 'NONE',  ( 1.249999999999999778, -0.000000000000000000, -10.00000000000000000 ) ) ;
#42923=ORIENTED_EDGE ( 'NONE', *, *, #6431, .F. ) ;
#42935=CARTESIAN_POINT ( 'NONE',  ( 14.48769039275578407, 30.44468701195595983, 8.807470649214879543 ) ) ;
#42938=CARTESIAN_POINT ( 'NONE',  ( 1.249999999999999778, -0.000000000000000000, -3.333333333333333481 ) ) ;
#42948=CARTESIAN_POINT ( 'NONE',  ( 36.44255557191966943, 8.993813888722351990, -5.338708898921616708 ) ) ;
#42955=EDGE_LOOP ( 'NONE', ( #10734, #22923, #20504, #38330 ) ) ;
#42963=CARTESIAN_POINT ( 'NONE',  ( -4.672045878990125800, 33.19353511768168374, 1.847720168420772691 ) ) ;
#42967=CARTESIAN_POINT ( 'NONE',  ( -45.64490844644706158, -21.32281559348763977, 8.807470649214879543 ) ) ;
#42968=CARTESIAN_POINT ( 'NONE',  ( -8.277096487746778308, 33.14818118907697198, 7.455576670931136185 ) ) ;
#42970=FACE_OUTER_BOUND ( 'NONE', #10489, .T. ) ;
#42976=B_SPLINE_CURVE_WITH_KNOTS ( 'NONE', 3,
 ( #43575, #11075, #8445, #45937 ),
 .UNSPECIFIED., .F., .F.,
 ( 4, 4 ),
 ( 0.0009679537044784938989, 0.001281751046851235375 ),
 .UNSPECIFIED. ) ;
#42980=CARTESIAN_POINT ( 'NONE',  ( 6.875132362119187768, -50.00000000000000711, 8.356839323120299312 ) ) ;
#42982=CARTESIAN_POINT ( 'NONE',  ( 21.17460298198255231, 30.99364813079834491, -3.721387749823085400 ) ) ;
#42988=CARTESIAN_POINT ( 'NONE',  ( 2.948105490344985480, 9.555557232197198658, 9.282506307616484875 ) ) ;
#43005=CARTESIAN_POINT ( 'NONE',  ( -0.1287570809895658697, 0.3962735484563123523, -10.00000000000000000 ) ) ;
#43009=CARTESIAN_POINT ( 'NONE',  ( 4.997594231923199182, 3.246827887979424787, -2.642742795433417058E-16 ) ) ;
#43021=VERTEX_POINT ( 'NONE', #14676 ) ;
#43029=CARTESIAN_POINT ( 'NONE',  ( 2.391286777838985245, -5.398370916123746532, 9.586754400234157814 ) ) ;
#43032=ADVANCED_FACE ( 'NONE', ( #46951 ), #41288, .T. ) ;
#43033=CARTESIAN_POINT ( 'NONE',  ( 0.6812130152897633018, 2.552013566577088888, 9.847478321177755234 ) ) ;
#43044=VERTEX_POINT ( 'NONE', #5145 ) ;
#43051=CARTESIAN_POINT ( 'NONE',  ( 2.538055338523177440, 50.00000000000000711, -9.367992836599954742 ) ) ;
#43054=FACE_OUTER_BOUND ( 'NONE', #5624, .T. ) ;
#43057=CARTESIAN_POINT ( 'NONE',  ( -1.011271242968687867, 0.7347315653655861478, 9.972675548442463622 ) ) ;
#43061=CARTESIAN_POINT ( 'NONE',  ( -2.536646476037189846, -2.794100479408525128, 9.865049507598756762 ) ) ;
#43081=CARTESIAN_POINT ( 'NONE',  ( -34.08355720199904226, 2.371364769369340042, 7.455576670931136185 ) ) ;
#43083=AXIS2_PLACEMENT_3D ( 'NONE', #43106, #19757, #46912 ) ;
#43100=ORIENTED_EDGE ( 'NONE', *, *, #12335, .T. ) ;
#43106=CARTESIAN_POINT ( 'NONE',  ( 0.000000000000000000, 0.000000000000000000, 0.000000000000000000 ) ) ;
#43114=CARTESIAN_POINT ( 'NONE',  ( 8.176860274785711979, -5.756644512789521606, 9.282506307616484875 ) ) ;
#43116=CARTESIAN_POINT ( 'NONE',  ( 6.174150299305392053, -33.14591993373988998, 8.807470649214879543 ) ) ;
#43119=CARTESIAN_POINT ( 'NONE',  ( 1.468446590252912465, 0.3226319952343980058, 9.953784399990622589 ) ) ;
#43121=ORIENTED_EDGE ( 'NONE', *, *, #29333, .F. ) ;
#43130=CARTESIAN_POINT ( 'NONE',  ( -22.69295089195507487, -45.31600496604688999, 7.455576670931136185 ) ) ;
#43145=CARTESIAN_POINT ( 'NONE',  ( 2.210477865340801706, 37.43479381012853224, -9.422646554964178023 ) ) ;
#43147=EDGE_CURVE ( 'NONE', #17682, #11134, #24743, .T. ) ;
#43154=EDGE_CURVE ( 'NONE', #46476, #290, #9365, .T. ) ;
#43159=ORIENTED_EDGE ( 'NONE', *, *, #25759, .T. ) ;
#43165=VECTOR ( 'NONE', #3213, 1000.000000000000000 ) ;
#43167=CARTESIAN_POINT ( 'NONE',  ( -8.277096487746778308, 50.00000000000000000, 7.455576670931136185 ) ) ;
#43181=CARTESIAN_POINT ( 'NONE',  ( -0.2099955233291965206, -1.205406147626143509, 9.993783931180535873 ) ) ;
#43184=CARTESIAN_POINT ( 'NONE',  ( -1.962712821592842882, -1.022159834731130257, 9.881002359080275355 ) ) ;
#43192=B_SPLINE_CURVE_WITH_KNOTS ( 'NONE', 3,
 ( #42988, #26845, #11207, #23513 ),
 .UNSPECIFIED., .F., .F.,
 ( 4, 4 ),
 ( 1.404617285391336434E-17, 0.009404495247862658044 ),
 .UNSPECIFIED. ) ;
#43194=CARTESIAN_POINT ( 'NONE',  ( 3.222683565149129237, 0.4845875505058722110, 9.799352050262459812 ) ) ;
#43210=CARTESIAN_POINT ( 'NONE',  ( 26.42016489236587873, 32.24895757977031963, -9.387872844313825738 ) ) ;
#43212=EDGE_CURVE ( 'NONE', #38645, #49869, #29512, .T. ) ;
#43214=CARTESIAN_POINT ( 'NONE',  ( -0.3862712429686809279, -1.188820645368943163, 10.00000000000000000 ) ) ;
#43232=CARTESIAN_POINT ( 'NONE',  ( 26.18032376592674737, -21.95228666728361233, 7.455576670931136185 ) ) ;
#43235=ORIENTED_EDGE ( 'NONE', *, *, #31789, .T. ) ;
#43241=CARTESIAN_POINT ( 'NONE',  ( 6.875132362119187768, -33.14667368551891258, 8.356839323120299312 ) ) ;
#43251=DIRECTION ( 'NONE',  ( -0.000000000000000000, -0.000000000000000000, -1.000000000000000000 ) ) ;
#43252=CARTESIAN_POINT ( 'NONE',  ( -46.76852358249002606, 17.86468378716741512, -9.367992836599951190 ) ) ;
#43260=CARTESIAN_POINT ( 'NONE',  ( 1.011271242968694084, -0.7347315653655782652, 10.00000000000000000 ) ) ;
#43270=CARTESIAN_POINT ( 'NONE',  ( -50.11058929355266400, 7.578863168071933387, 7.455576670931136185 ) ) ;
#43271=B_SPLINE_CURVE_WITH_KNOTS ( 'NONE', 3,
 ( #14476, #26286, #37360, #25521 ),
 .UNSPECIFIED., .F., .F.,
 ( 4, 4 ),
 ( 0.000000000000000000, 0.009404495247862337121 ),
 .UNSPECIFIED. ) ;
#43281=B_SPLINE_SURFACE_WITH_KNOTS ( 'NONE', 3, 3, ( 
 ( #15025, #50374, #26829, #22963 ),
 ( #3457, #15291, #30950, #46536 ),
 ( #27079, #24761, #25009, #8848 ),
 ( #13194, #12689, #28350, #27849 ) ),
 .UNSPECIFIED., .F., .F., .F.,
 ( 4, 4 ),
 ( 4, 4 ),
 ( 0.000000000000000000, 1.000000000000000000 ),
 ( 0.000000000000000000, 1.000000000000000000 ),
 .UNSPECIFIED. ) ;
#43284=CARTESIAN_POINT ( 'NONE',  ( 0.3862712429686978033, -1.188820645368937834, 3.333333333333333481 ) ) ;
#43291=ADVANCED_FACE ( 'NONE', ( #42319 ), #1957, .T. ) ;
#43304=ORIENTED_EDGE ( 'NONE', *, *, #43154, .F. ) ;
#43311=CARTESIAN_POINT ( 'NONE',  ( -1.250000000000000222, 0.000000000000000000, 10.00000000000000000 ) ) ;
#43313=DIRECTION ( 'NONE',  ( 0.000000000000000000, 0.000000000000000000, 1.000000000000000000 ) ) ;
#43315=CARTESIAN_POINT ( 'NONE',  ( 3.231548175622897645, -9.463461120997347820, 9.282506307616472441 ) ) ;
#43316=CARTESIAN_POINT ( 'NONE',  ( -2.774199681320129951, -2.805557802885433993, 6.494306115488113207 ) ) ;
#43323=CARTESIAN_POINT ( 'NONE',  ( 47.55282581475783132, -15.45084971874691604, 0.000000000000000000 ) ) ;
#43328=ORIENTED_EDGE ( 'NONE', *, *, #40945, .F. ) ;
#43334=EDGE_LOOP ( 'NONE', ( #44230, #35456, #11896, #13356, #39015, #32269, #25620, #45424, #3522, #11233, #29664, #50713, #49878, #1233 ) ) ;
#43335=VECTOR ( 'NONE', #42782, 1000.000000000000000 ) ;
#43337=CARTESIAN_POINT ( 'NONE',  ( -1.275927284277175167, 0.1224368140627496299, 9.976582533991679824 ) ) ;
#43338=ORIENTED_EDGE ( 'NONE', *, *, #44797, .F. ) ;
#43350=EDGE_CURVE ( 'NONE', #13694, #26320, #21632, .T. ) ;
#43370=CARTESIAN_POINT ( 'NONE',  ( 14.52758583651987223, 8.922352469211173087, 8.953103998512858652 ) ) ;
#43372=CARTESIAN_POINT ( 'NONE',  ( 28.96803024440893992, 18.11533787072037072, 7.455576670931136185 ) ) ;
#43379=CARTESIAN_POINT ( 'NONE',  ( 2.538055338523173443, 45.80735277814159190, -9.367992836599951190 ) ) ;
#43391=FACE_BOUND ( 'NONE', #31612, .T. ) ;
#43413=ORIENTED_EDGE ( 'NONE', *, *, #11158, .T. ) ;
#43430=CARTESIAN_POINT ( 'NONE',  ( -8.277096487746778308, 50.00000000000000711, 7.455576670931136185 ) ) ;
#43452=CARTESIAN_POINT ( 'NONE',  ( 4.672045878990125800, -50.00000000000000711, 1.847720168420772691 ) ) ;
#43453=CARTESIAN_POINT ( 'NONE',  ( 26.18032376592674737, -21.95228666728361233, 7.455576670931136185 ) ) ;
#43454=ORIENTED_EDGE ( 'NONE', *, *, #7400, .F. ) ;
#43460=CARTESIAN_POINT ( 'NONE',  ( -48.98697415750977768, -11.03699497439218646, -8.016098858316199838 ) ) ;
#43463=ORIENTED_EDGE ( 'NONE', *, *, #15300, .T. ) ;
#43465=CARTESIAN_POINT ( 'NONE',  ( -41.59994237955809382, 5.070535260985659320, 7.544061037322998153 ) ) ;
#43468=CARTESIAN_POINT ( 'NONE',  ( 1.249999999999999778, -0.000000000000000000, -10.00000000000000000 ) ) ;
#43475=CARTESIAN_POINT ( 'NONE',  ( -0.3370904143228978245, 0.2449105217885259589, 10.00000000000000000 ) ) ;
#43483=CARTESIAN_POINT ( 'NONE',  ( -6.875132362119187768, 33.14667368551891258, 8.356839323120299312 ) ) ;
#43494=ORIENTED_EDGE ( 'NONE', *, *, #37948, .T. ) ;
#43497=CARTESIAN_POINT ( 'NONE',  ( 1.962558162476984114, -3.366505435497487042, 9.741991644047251597 ) ) ;
#43498=CARTESIAN_POINT ( 'NONE',  ( 1.011271242968688311, -0.7347315653655855927, -3.333333333333333481 ) ) ;
#43499=ADVANCED_FACE ( 'NONE', ( #30121 ), #46194, .T. ) ;
#43503=CARTESIAN_POINT ( 'NONE',  ( 1.377509002708426689, -0.6027468487254984408, 9.927319414211227766 ) ) ;
#43519=B_SPLINE_CURVE_WITH_KNOTS ( 'NONE', 3,
 ( #49959, #2796, #3050, #45629 ),
 .UNSPECIFIED., .F., .F.,
 ( 4, 4 ),
 ( 0.000000000000000000, 0.0003726855806051465212 ),
 .UNSPECIFIED. ) ;
#43520=DIRECTION ( 'NONE',  ( 0.3090169943749447312, 0.9510565162951544194, 0.000000000000000000 ) ) ;
#43528=CARTESIAN_POINT ( 'NONE',  ( -3.975459390375366997, -0.2195152216756601216, -2.642742795433417058E-16 ) ) ;
#43530=CARTESIAN_POINT ( 'NONE',  ( 0.7455485644579565863, 0.9687920084208806459, 9.987567862361069970 ) ) ;
#43531=B_SPLINE_CURVE_WITH_KNOTS ( 'NONE', 3,
 ( #17874, #13524, #45056, #20727 ),
 .UNSPECIFIED., .F., .F.,
 ( 4, 4 ),
 ( 5.641302087905949829E-05, 0.0003272669002638295692 ),
 .UNSPECIFIED. ) ;
#43553=VERTEX_POINT ( 'NONE', #38598 ) ;
#43573=CARTESIAN_POINT ( 'NONE',  ( 1.540662627795932105, -1.371465786296032441, 9.894754715216729224 ) ) ;
#43575=CARTESIAN_POINT ( 'NONE',  ( -1.655785408455817675, -0.7536129375911022610, 9.903764339332079558 ) ) ;
#43584=CARTESIAN_POINT ( 'NONE',  ( 7.216980890441427654, -6.922079660550236824, 0.000000000000000000 ) ) ;
#43595=CARTESIAN_POINT ( 'NONE',  ( 33.57695195286775913, 16.69845195084893064, 8.914903342594561408 ) ) ;
#43631=FACE_OUTER_BOUND ( 'NONE', #3731, .T. ) ;
#43632=CARTESIAN_POINT ( 'NONE',  ( -2.143303251558873690, 0.2857918750721046286, 9.885585981620941709 ) ) ;
#43671=ADVANCED_FACE ( 'NONE', ( #4193 ), #6902, .T. ) ;
#43685=ORIENTED_EDGE ( 'NONE', *, *, #23321, .F. ) ;
#43694=B_SPLINE_CURVE_WITH_KNOTS ( 'NONE', 3,
 ( #19169, #27911, #43029, #26884 ),
 .UNSPECIFIED., .F., .F.,
 ( 4, 4 ),
 ( 0.8097120833243680593, 0.9322955464062570030 ),
 .UNSPECIFIED. ) ;
#43701=B_SPLINE_SURFACE_WITH_KNOTS ( 'NONE', 3, 3, ( 
 ( #37899, #21712, #33030, #48616 ),
 ( #14006, #25074, #44531, #26073 ),
 ( #37400, #14262, #29926, #33289 ),
 ( #45542, #22224, #9416, #10171 ) ),
 .UNSPECIFIED., .F., .F., .F.,
 ( 4, 4 ),
 ( 4, 4 ),
 ( 0.000000000000000000, 1.000000000000000000 ),
 ( 0.000000000000000000, 1.000000000000000000 ),
 .UNSPECIFIED. ) ;
#43705=EDGE_CURVE ( 'NONE', #10853, #5199, #24203, .T. ) ;
#43715=B_SPLINE_CURVE_WITH_KNOTS ( 'NONE', 3,
 ( #37861, #35036, #11658, #15262 ),
 .UNSPECIFIED., .F., .F.,
 ( 4, 4 ),
 ( 0.7491799374948678869, 1.000000000000000000 ),
 .UNSPECIFIED. ) ;
#43717=ORIENTED_EDGE ( 'NONE', *, *, #27233, .F. ) ;
#43719=CARTESIAN_POINT ( 'NONE',  ( -1.249999999999999778, 0.000000000000000000, -10.00000000000000000 ) ) ;
#43734=CARTESIAN_POINT ( 'NONE',  ( 45.42829307628542779, 21.98948915213303579, 8.356839323120299312 ) ) ;
#43739=ORIENTED_EDGE ( 'NONE', *, *, #28856, .T. ) ;
#43742=ORIENTED_EDGE ( 'NONE', *, *, #46193, .F. ) ;
#43748=LINE ( 'NONE', #39927, #10127 ) ;
#43757=CARTESIAN_POINT ( 'NONE',  ( -1.962712821592842882, -1.022159834731130257, 9.881002359080275355 ) ) ;
#43772=B_SPLINE_CURVE_WITH_KNOTS ( 'NONE', 3,
 ( #40701, #48592, #28137, #29150 ),
 .UNSPECIFIED., .F., .F.,
 ( 4, 4 ),
 ( 0.9890644561682315761, 1.000000000000000000 ),
 .UNSPECIFIED. ) ;
#43775=CARTESIAN_POINT ( 'NONE',  ( 0.3862712429686978033, -1.188820645368937834, -10.00000000000000000 ) ) ;
#43778=CARTESIAN_POINT ( 'NONE',  ( -33.38053581724533814, -17.16548397897120282, 4.835783797351804303 ) ) ;
#43781=CARTESIAN_POINT ( 'NONE',  ( 34.95136153415558056, -36.40974830873469870, 8.356839323120299312 ) ) ;
#43790=EDGE_CURVE ( 'NONE', #47214, #18098, #5080, .T. ) ;
#43802=CARTESIAN_POINT ( 'NONE',  ( 12.35406723005396046, -11.51001571518080624, 9.178419661560148768 ) ) ;
#43805=ORIENTED_EDGE ( 'NONE', *, *, #22988, .T. ) ;
#43807=CARTESIAN_POINT ( 'NONE',  ( 9.221081804193270059, 13.81382350053991104, 3.266473740018926541 ) ) ;
#43811=B_SPLINE_CURVE_WITH_KNOTS ( 'NONE', 3,
 ( #31481, #19144, #4275, #27116 ),
 .UNSPECIFIED., .F., .F.,
 ( 4, 4 ),
 ( 0.8097120833243680593, 0.9322955464061821740 ),
 .UNSPECIFIED. ) ;
#43816=CARTESIAN_POINT ( 'NONE',  ( -0.2773062244624664441, 1.251557370488897813, 9.948547179989621014 ) ) ;
#43818=CARTESIAN_POINT ( 'NONE',  ( -1.377636575563021992, 0.6021164824561227036, 9.953784399990620813 ) ) ;
#43822=CARTESIAN_POINT ( 'NONE',  ( 47.87295225382209907, 14.46560184742433641, -2.408242355805840784 ) ) ;
#43824=EDGE_CURVE ( 'NONE', #2268, #41040, #35112, .T. ) ;
#43826=VECTOR ( 'NONE', #18027, 999.9999999999998863 ) ;
#43838=EDGE_LOOP ( 'NONE', ( #1310, #27767, #33315, #10081, #44638, #49746, #7834, #40287, #35841, #42170, #32633, #41735 ) ) ;
#43860=CARTESIAN_POINT ( 'NONE',  ( -26.76882631152605185, 42.35470813487695807, -8.917361510505369182 ) ) ;
#43864=CARTESIAN_POINT ( 'NONE',  ( 0.6595498452743703277, -16.59563386392009576, 3.266473740018926541 ) ) ;
#43875=CARTESIAN_POINT ( 'NONE',  ( 0.9870575514054733546, 1.980598328282569653, 9.881002359080278907 ) ) ;
#43876=CARTESIAN_POINT ( 'NONE',  ( 0.6215990105956902267, -1.608617984725389860, 9.928159647716132241 ) ) ;
#43903=VERTEX_POINT ( 'NONE', #31080 ) ;
#43910=CARTESIAN_POINT ( 'NONE',  ( -6.619412807845042046, 7.495556955913086128, 9.646707543097347681 ) ) ;
#43912=EDGE_LOOP ( 'NONE', ( #33402, #2562, #45331, #23171 ) ) ;
#43915=CARTESIAN_POINT ( 'NONE',  ( 1.578643388466006714, -1.550786058692517511, 9.881002359080275355 ) ) ;
#43927=VERTEX_POINT ( 'NONE', #25973 ) ;
#43928=B_SPLINE_CURVE_WITH_KNOTS ( 'NONE', 3,
 ( #13373, #5672, #14119, #20819 ),
 .UNSPECIFIED., .F., .F.,
 ( 4, 4 ),
 ( 1.788112030672749005E-18, 0.009404495247862344059 ),
 .UNSPECIFIED. ) ;
#43935=EDGE_LOOP ( 'NONE', ( #6182, #31062, #31918, #10091 ) ) ;
#43936=EDGE_LOOP ( 'NONE', ( #10562, #39480, #4535, #27913 ) ) ;
#43939=CARTESIAN_POINT ( 'NONE',  ( 4.531159320492035292, 41.49457383023836599, -8.080361901872242569 ) ) ;
#43952=CARTESIAN_POINT ( 'NONE',  ( -7.608425291889091113, 36.72004717559254772, 7.697694107796188234 ) ) ;
#43968=CARTESIAN_POINT ( 'NONE',  ( -0.3862712429686895876, 1.188820645368940720, 10.00000000000000000 ) ) ;
#43969=CARTESIAN_POINT ( 'NONE',  ( 16.52264463346132572, -2.779753662172757878, 9.403735324607438884 ) ) ;
#43972=VERTEX_POINT ( 'NONE', #26462 ) ;
#43975=CARTESIAN_POINT ( 'NONE',  ( 33.43156050989131955, -4.370686678976570150, 8.807470649214879543 ) ) ;
#43976=EDGE_CURVE ( 'NONE', #16962, #50249, #6286, .T. ) ;
#43990=EDGE_CURVE ( 'NONE', #36961, #26037, #49661, .T. ) ;
#43992=CARTESIAN_POINT ( 'NONE',  ( -8.843309649387274263, 14.11631751497152720, -2.870787844569587133 ) ) ;
#43994=ORIENTED_EDGE ( 'NONE', *, *, #46886, .F. ) ;
#43995=CARTESIAN_POINT ( 'NONE',  ( -1.250000000000000222, 0.000000000000000000, 3.333333333333333481 ) ) ;
#43998=ORIENTED_EDGE ( 'NONE', *, *, #19919, .T. ) ;
#44001=EDGE_LOOP ( 'NONE', ( #6680, #38045, #25743, #1794 ) ) ;
#44009=B_SPLINE_SURFACE_WITH_KNOTS ( 'NONE', 3, 3, ( 
 ( #9919, #40220, #25578, #9165 ),
 ( #21717, #37405, #28426, #24571 ),
 ( #5055, #16877, #24826, #20715 ),
 ( #36392, #5315, #1235, #32539 ) ),
 .UNSPECIFIED., .F., .F., .F.,
 ( 4, 4 ),
 ( 4, 4 ),
 ( 0.000000000000000000, 1.000000000000000000 ),
 ( 0.000000000000000000, 1.000000000000000000 ),
 .UNSPECIFIED. ) ;
#44010=CARTESIAN_POINT ( 'NONE',  ( -18.69789054174323084, 27.49790346457746182, -2.408242355805840784 ) ) ;
#44025=CARTESIAN_POINT ( 'NONE',  ( 25.04522487443081502, -22.77512090857307925, 8.356839323120299312 ) ) ;
#44030=VERTEX_POINT ( 'NONE', #16679 ) ;
#44031=CARTESIAN_POINT ( 'NONE',  ( 1.275927284277173834, -0.1224368140627448004, 9.976582533991679824 ) ) ;
#44037=ORIENTED_EDGE ( 'NONE', *, *, #16194, .T. ) ;
#44042=B_SPLINE_CURVE_WITH_KNOTS ( 'NONE', 3,
 ( #9283, #2332, #25436, #9527 ),
 .UNSPECIFIED., .F., .F.,
 ( 4, 4 ),
 ( 1.119743386075808773E-15, 0.0004154657329505087246 ),
 .UNSPECIFIED. ) ;
#44043=CARTESIAN_POINT ( 'NONE',  ( 0.6440276692615888310, 16.64212148744554298, -9.683996418299976483 ) ) ;
#44052=ORIENTED_EDGE ( 'NONE', *, *, #8107, .F. ) ;
#44057=CARTESIAN_POINT ( 'NONE',  ( -1.780432407520014415, -1.041450996408466612, 9.894754715216725671 ) ) ;
#44075=ORIENTED_EDGE ( 'NONE', *, *, #11868, .F. ) ;
#44077=FACE_OUTER_BOUND ( 'NONE', #4004, .T. ) ;
#44081=ORIENTED_EDGE ( 'NONE', *, *, #49343, .F. ) ;
#44083=ORIENTED_EDGE ( 'NONE', *, *, #49413, .T. ) ;
#44084=CARTESIAN_POINT ( 'NONE',  ( 16.16402646813543242, -4.033894069732437693, -3.546734833711462365 ) ) ;
#44091=ORIENTED_EDGE ( 'NONE', *, *, #39802, .F. ) ;
#44096=ORIENTED_EDGE ( 'NONE', *, *, #6413, .F. ) ;
#44112=B_SPLINE_SURFACE_WITH_KNOTS ( 'NONE', 3, 3, ( 
 ( #33790, #49379, #14265, #29931 ),
 ( #45546, #19889, #11440, #157 ),
 ( #31207, #19642, #20842, #24706 ),
 ( #4254, #19124, #7862, #40353 ) ),
 .UNSPECIFIED., .F., .F., .F.,
 ( 4, 4 ),
 ( 4, 4 ),
 ( 0.000000000000000000, 1.000000000000000000 ),
 ( 0.000000000000000000, 1.000000000000000000 ),
 .UNSPECIFIED. ) ;
#44115=ADVANCED_FACE ( 'NONE', ( #25397 ), #13820, .T. ) ;
#44116=CARTESIAN_POINT ( 'NONE',  ( 0.7142790906314127053, -1.400791805248631672, 9.945241992664893615 ) ) ;
#44120=ORIENTED_EDGE ( 'NONE', *, *, #43154, .T. ) ;
#44124=CARTESIAN_POINT ( 'NONE',  ( -0.3370904143228943828, -0.2449105217885308716, 10.00000000000000000 ) ) ;
#44125=ORIENTED_EDGE ( 'NONE', *, *, #10927, .F. ) ;
#44133=CARTESIAN_POINT ( 'NONE',  ( -27.33593271309441519, 41.94268121623345991, -9.367992836599954742 ) ) ;
#44135=CARTESIAN_POINT ( 'NONE',  ( -30.21887974406478250, 14.69854701517550666, -8.016098858316199838 ) ) ;
#44143=ORIENTED_EDGE ( 'NONE', *, *, #10266, .F. ) ;
#44153=EDGE_CURVE ( 'NONE', #49290, #19115, #17280, .T. ) ;
#44158=B_SPLINE_CURVE_WITH_KNOTS ( 'NONE', 3,
 ( #22862, #31608, #42101, #7996 ),
 .UNSPECIFIED., .F., .F.,
 ( 4, 4 ),
 ( 0.001152428489661398280, 0.001623376834729528930 ),
 .UNSPECIFIED. ) ;
#44185=CARTESIAN_POINT ( 'NONE',  ( 4.641001526964561030, 50.00000000000000000, -8.016098858316205167 ) ) ;
#44190=CARTESIAN_POINT ( 'NONE',  ( -32.43949840348904701, -7.871562655726274116, -9.367992836599954742 ) ) ;
#44192=CARTESIAN_POINT ( 'NONE',  ( 1.250000000000000222, 0.000000000000000000, 10.00000000000000000 ) ) ;
#44204=B_SPLINE_CURVE_WITH_KNOTS ( 'NONE', 3,
 ( #38135, #17604, #37136, #41462 ),
 .UNSPECIFIED., .F., .F.,
 ( 4, 4 ),
 ( 0.002099423004388898967, 0.008237935836937843731 ),
 .UNSPECIFIED. ) ;
#44205=B_SPLINE_CURVE_WITH_KNOTS ( 'NONE', 3,
 ( #42746, #43009, #7625, #35097 ),
 .UNSPECIFIED., .F., .F.,
 ( 4, 4 ),
 ( 0.002645289245949297274, 0.008783374267191987328 ),
 .UNSPECIFIED. ) ;
#44212=CARTESIAN_POINT ( 'NONE',  ( 1.901953004002553405, 1.028591558669216255, 9.885585981620943485 ) ) ;
#44218=CARTESIAN_POINT ( 'NONE',  ( -0.3862712429686895876, 1.188820645368940720, -10.00000000000000000 ) ) ;
#44223=CARTESIAN_POINT ( 'NONE',  ( 12.78770032058947237, 31.68259716188277864, 7.455576670931136185 ) ) ;
#44230=ORIENTED_EDGE ( 'NONE', *, *, #47719, .F. ) ;
#44231=VERTEX_POINT ( 'NONE', #11004 ) ;
#44242=CARTESIAN_POINT ( 'NONE',  ( -10.30302290646040575, -13.08520913973572419, -9.683996418299976483 ) ) ;
#44244=CARTESIAN_POINT ( 'NONE',  ( 0.1287570809895660084, -0.3962735484563127408, 10.00000000000000000 ) ) ;
#44248=CARTESIAN_POINT ( 'NONE',  ( -0.3862712429686809279, -1.188820645368943163, -10.00000000000000000 ) ) ;
#44249=ORIENTED_EDGE ( 'NONE', *, *, #42434, .F. ) ;
#44256=CARTESIAN_POINT ( 'NONE',  ( -16.16402646813540755, 4.033894069732547827, -3.546734833711462365 ) ) ;
#44258=B_SPLINE_CURVE_WITH_KNOTS ( 'NONE', 3,
 ( #29656, #26322, #2458, #13748 ),
 .UNSPECIFIED., .F., .F.,
 ( 4, 4 ),
 ( 1.734723475976807094E-18, 8.326314925919050278E-06 ),
 .UNSPECIFIED. ) ;
#44259=CARTESIAN_POINT ( 'NONE',  ( -2.948105490345101387, -9.555557232197246620, 9.282506307616472441 ) ) ;
#44260=LINE ( 'NONE', #40695, #37377 ) ;
#44267=CARTESIAN_POINT ( 'NONE',  ( -14.48769039275601145, -30.44468701195584970, 8.807470649214879543 ) ) ;
#44277=CARTESIAN_POINT ( 'NONE',  ( -16.99749102614300966, 1.320765928724422222, 8.953103998512858652 ) ) ;
#44282=ORIENTED_EDGE ( 'NONE', *, *, #25495, .T. ) ;
#44290=ORIENTED_EDGE ( 'NONE', *, *, #17405, .F. ) ;
#44296=ORIENTED_EDGE ( 'NONE', *, *, #31938, .T. ) ;
#44301=EDGE_CURVE ( 'NONE', #41021, #42350, #35661, .T. ) ;
#44314=VECTOR ( 'NONE', #43520, 1000.000000000000000 ) ;
#44319=CARTESIAN_POINT ( 'NONE',  ( 2.538055338523173443, 50.00000000000000000, -9.367992836599951190 ) ) ;
#44323=ADVANCED_FACE ( 'NONE', ( #43054 ), #13411, .T. ) ;
#44341=ORIENTED_EDGE ( 'NONE', *, *, #21185, .F. ) ;
#44344=EDGE_LOOP ( 'NONE', ( #13553, #22794, #2773, #3416 ) ) ;
#44353=EDGE_CURVE ( 'NONE', #8231, #5904, #12269, .T. ) ;
#44365=CARTESIAN_POINT ( 'NONE',  ( 0.3370904143228947158, 0.2449105217885311492, 10.00000000000000000 ) ) ;
#44367=CARTESIAN_POINT ( 'NONE',  ( 10.30302290646030627, 13.08520913973580058, -9.683996418299976483 ) ) ;
#44380=CARTESIAN_POINT ( 'NONE',  ( -20.40054609052957701, 26.26366202847989229, -3.760136334089591248 ) ) ;
#44381=CARTESIAN_POINT ( 'NONE',  ( 0.3862712429686810944, 1.188820645368943607, 3.333333333333333481 ) ) ;
#44384=CARTESIAN_POINT ( 'NONE',  ( -14.29087950072019098, -9.652079258044555132, 8.727788335465566760 ) ) ;
#44388=ORIENTED_EDGE ( 'NONE', *, *, #12059, .F. ) ;
#44391=ORIENTED_EDGE ( 'NONE', *, *, #32914, .F. ) ;
#44408=AXIS2_PLACEMENT_3D ( 'NONE', #11384, #10876, #50073 ) ;
#44421=B_SPLINE_SURFACE_WITH_KNOTS ( 'NONE', 3, 3, ( 
 ( #13740, #25806, #45524, #9396 ),
 ( #21952, #6044, #10406, #6311 ),
 ( #25297, #26057, #1703, #41705 ),
 ( #44773, #6553, #49603, #14500 ) ),
 .UNSPECIFIED., .F., .F., .F.,
 ( 4, 4 ),
 ( 4, 4 ),
 ( 0.000000000000000000, 1.000000000000000000 ),
 ( 0.000000000000000000, 1.000000000000000000 ),
 .UNSPECIFIED. ) ;
#44430=CARTESIAN_POINT ( 'NONE',  ( 4.339432828817248122, 37.24807810779213213, -8.192531242611266862 ) ) ;
#44435=CARTESIAN_POINT ( 'NONE',  ( -14.29087950072019098, -9.652079258044555132, 8.727788335465566760 ) ) ;
#44437=CARTESIAN_POINT ( 'NONE',  ( -3.996390545799824334, 16.57371371864897469, 8.953103998512858652 ) ) ;
#44446=CARTESIAN_POINT ( 'NONE',  ( -0.1469336902871204442, -1.496274467947957376, 9.953784399990622589 ) ) ;
#44463=CARTESIAN_POINT ( 'NONE',  ( -1.011271242968693862, 0.7347315653655780432, 10.00000000000000000 ) ) ;
#44465=CARTESIAN_POINT ( 'NONE',  ( -0.1287570809895576818, -0.3962735484563154609, 10.00000000000000000 ) ) ;
#44478=ORIENTED_EDGE ( 'NONE', *, *, #17055, .T. ) ;
#44479=ORIENTED_EDGE ( 'NONE', *, *, #50556, .F. ) ;
#44483=CARTESIAN_POINT ( 'NONE',  ( -27.33593271309441519, 41.94268121623345280, -9.367992836599951190 ) ) ;
#44493=CARTESIAN_POINT ( 'NONE',  ( 33.86622497129647513, -3.037805405904928868, 7.906207997025717304 ) ) ;
#44496=DIRECTION ( 'NONE',  ( 0.000000000000000000, 0.000000000000000000, 1.000000000000000000 ) ) ;
#44501=CARTESIAN_POINT ( 'NONE',  ( -0.3862712429686809279, -1.188820645368943163, -3.333333333333333481 ) ) ;
#44509=CARTESIAN_POINT ( 'NONE',  ( -1.377509002708424468, 0.6027468487255034368, 9.927319414211229542 ) ) ;
#44510=DIRECTION ( 'NONE',  ( -1.000000000000000000, 0.000000000000000000, 0.000000000000000000 ) ) ;
#44521=B_SPLINE_SURFACE_WITH_KNOTS ( 'NONE', 3, 3, ( 
 ( #6704, #45924, #22350, #10549 ),
 ( #38026, #26214, #2841, #18501 ),
 ( #34181, #14656, #30316, #42096 ),
 ( #22610, #38292, #3100, #14914 ) ),
 .UNSPECIFIED., .F., .F., .F.,
 ( 4, 4 ),
 ( 4, 4 ),
 ( 0.000000000000000000, 1.000000000000000000 ),
 ( 0.000000000000000000, 1.000000000000000000 ),
 .UNSPECIFIED. ) ;
#44530=CARTESIAN_POINT ( 'NONE',  ( 2.538055338523177440, 50.00000000000000711, -9.367992836599954742 ) ) ;
#44531=CARTESIAN_POINT ( 'NONE',  ( 16.76006782980217125, -2.050259795448531541, 9.178419661560148768 ) ) ;
#44532=CARTESIAN_POINT ( 'NONE',  ( -1.256098972485658383, -0.9750543259410950903, 9.933337059263825708 ) ) ;
#44546=CARTESIAN_POINT ( 'NONE',  ( 36.76598589393955052, 7.383243274241862331, -8.192531242611266862 ) ) ;
#44550=CARTESIAN_POINT ( 'NONE',  ( 0.8155877869298099325, 0.9072449372238458043, 9.963925895597341764 ) ) ;
#44552=CARTESIAN_POINT ( 'NONE',  ( -20.40054609052957701, 26.26366202847989229, -3.760136334089591248 ) ) ;
#44555=CARTESIAN_POINT ( 'NONE',  ( -24.47767542868268364, 23.18653802921800278, 8.807470649214879543 ) ) ;
#44582=CARTESIAN_POINT ( 'NONE',  ( 0.1287570809895660084, -0.3962735484563127408, 10.00000000000000000 ) ) ;
#44585=CARTESIAN_POINT ( 'NONE',  ( -0.9601844228325777664, 0.8491947203466829741, 9.967237415621765351 ) ) ;
#44586=EDGE_CURVE ( 'NONE', #40675, #49396, #14809, .T. ) ;
#44602=ORIENTED_EDGE ( 'NONE', *, *, #31640, .F. ) ;
#44603=EDGE_CURVE ( 'NONE', #50662, #29288, #24005, .T. ) ;
#44604=CARTESIAN_POINT ( 'NONE',  ( -1.186340292695371668, 0.3298841998003470555, 9.975326647350893694 ) ) ;
#44605=CARTESIAN_POINT ( 'NONE',  ( 1.275927284277173834, -0.1224368140627448004, 9.976582533991679824 ) ) ;
#44607=EDGE_CURVE ( 'NONE', #1676, #37965, #1036, .T. ) ;
#44617=B_SPLINE_CURVE_WITH_KNOTS ( 'NONE', 3,
 ( #43595, #4362, #35428, #20000 ),
 .UNSPECIFIED., .F., .F.,
 ( 4, 4 ),
 ( 0.000000000000000000, 0.002458791966311105019 ),
 .UNSPECIFIED. ) ;
#44622=CARTESIAN_POINT ( 'NONE',  ( 1.275994128725544741, -0.1230186051320594776, 9.948547179989619238 ) ) ;
#44626=CARTESIAN_POINT ( 'NONE',  ( 0.3862712429686894766, -1.188820645368940276, -10.00000000000000000 ) ) ;
#44630=VERTEX_POINT ( 'NONE', #7037 ) ;
#44632=EDGE_CURVE ( 'NONE', #76, #3380, #17174, .T. ) ;
#44638=ORIENTED_EDGE ( 'NONE', *, *, #41290, .T. ) ;
#44646=EDGE_LOOP ( 'NONE', ( #43454, #17372, #34084, #26629, #6533 ) ) ;
#44659=CARTESIAN_POINT ( 'NONE',  ( 32.57170742938662755, 18.58316106410423174, 7.697694107796188234 ) ) ;
#44663=DIRECTION ( 'NONE',  ( -1.000000000000000000, 0.000000000000000000, 0.000000000000000000 ) ) ;
#44671=AXIS2_PLACEMENT_3D ( 'NONE', #25490, #21906, #41138 ) ;
#44674=ORIENTED_EDGE ( 'NONE', *, *, #20465, .T. ) ;
#44679=CARTESIAN_POINT ( 'NONE',  ( 49.46074318306830975, -9.578883844006833570, 8.807470649214879543 ) ) ;
#44683=CARTESIAN_POINT ( 'NONE',  ( -4.763548243873389154, 16.57409059453848599, 8.727788335465566760 ) ) ;
#44685=B_SPLINE_CURVE_WITH_KNOTS ( 'NONE', 3,
 ( #20869, #23966, #47532, #1134 ),
 .UNSPECIFIED., .F., .F.,
 ( 4, 4 ),
 ( 0.7491799374948679979, 1.000000000000000000 ),
 .UNSPECIFIED. ) ;
#44689=CARTESIAN_POINT ( 'NONE',  ( 2.491056982571220768, -9.716321351877633461, 9.390253821402618328 ) ) ;
#44696=ORIENTED_EDGE ( 'NONE', *, *, #26594, .F. ) ;
#44699=CARTESIAN_POINT ( 'NONE',  ( -0.3862712429686895876, 1.188820645368940720, 3.333333333333333481 ) ) ;
#44706=ORIENTED_EDGE ( 'NONE', *, *, #23029, .F. ) ;
#44710=ORIENTED_EDGE ( 'NONE', *, *, #17733, .T. ) ;
#44713=CARTESIAN_POINT ( 'NONE',  ( -0.6679403265625625252, 1.504705676290988725, 9.936700280135882579 ) ) ;
#44715=CARTESIAN_POINT ( 'NONE',  ( -0.3862712429686895876, 1.188820645368940720, 3.333333333333333481 ) ) ;
#44716=CARTESIAN_POINT ( 'NONE',  ( -7.608425291889091113, 36.72004717559254772, 7.697694107796188234 ) ) ;
#44720=CARTESIAN_POINT ( 'NONE',  ( -1.411185367335151541, -16.64174154430383012, -9.458680755252684591 ) ) ;
#44721=CARTESIAN_POINT ( 'NONE',  ( -0.3862712429686977478, 1.188820645368937390, 3.333333333333333481 ) ) ;
#44726=DIRECTION ( 'NONE',  ( 0.000000000000000000, 0.000000000000000000, -1.000000000000000000 ) ) ;
#44730=CIRCLE ( 'NONE', #40698, 10.00000000000000000 ) ;
#44760=CARTESIAN_POINT ( 'NONE',  ( -1.011271242968683426, -0.7347315653655928092, 10.00000000000000000 ) ) ;
#44761=CARTESIAN_POINT ( 'NONE',  ( 47.88254548617766204, -14.43607691413525984, -3.760136334089591248 ) ) ;
#44773=CARTESIAN_POINT ( 'NONE',  ( -48.33712804702535948, -13.03701565032741527, -9.367992836599954742 ) ) ;
#44775=CARTESIAN_POINT ( 'NONE',  ( 6.174150299305392053, -45.68101107938186800, 8.807470649214879543 ) ) ;
#44780=CARTESIAN_POINT ( 'NONE',  ( -34.08355720199904226, 2.371364769369340042, 7.455576670931136185 ) ) ;
#44781=B_SPLINE_CURVE_WITH_KNOTS ( 'NONE', 3,
 ( #13967, #2431, #29881, #25275 ),
 .UNSPECIFIED., .F., .F.,
 ( 4, 4 ),
 ( 2.680765238357722860E-17, 0.0004072981213157027118 ),
 .UNSPECIFIED. ) ;
#44790=B_SPLINE_CURVE_WITH_KNOTS ( 'NONE', 3,
 ( #43952, #48268, #24475, #36290, #20864, #4955 ),
 .UNSPECIFIED., .F., .F.,
 ( 4, 2, 4 ),
 ( 4.635316164197443437E-17, 0.009882509389272372408, 0.01976501877854469624 ),
 .UNSPECIFIED. ) ;
#44791=CARTESIAN_POINT ( 'NONE',  ( -1.249999999999999778, 0.000000000000000000, 3.333333333333333481 ) ) ;
#44793=CARTESIAN_POINT ( 'NONE',  ( -5.888214538810513154, -16.20866436362413410, 8.727788335465566760 ) ) ;
#44794=ORIENTED_EDGE ( 'NONE', *, *, #7758, .F. ) ;
#44797=EDGE_CURVE ( 'NONE', #43553, #40295, #14717, .T. ) ;
#44804=DIRECTION ( 'NONE',  ( 0.6805276818820472640, -0.4944323023721970412, 0.5407575913134972101 ) ) ;
#44818=CARTESIAN_POINT ( 'NONE',  ( -10.70590866674912967, 12.76446523155714985, -3.546734833711462365 ) ) ;
#44820=CARTESIAN_POINT ( 'NONE',  ( 1.011271242968683648, 0.7347315653655930312, 10.00000000000000000 ) ) ;
#44846=ORIENTED_EDGE ( 'NONE', *, *, #41866, .F. ) ;
#44853=ORIENTED_EDGE ( 'NONE', *, *, #23673, .T. ) ;
#44856=CARTESIAN_POINT ( 'NONE',  ( -7.608425291889091113, 36.72004717559254772, 7.697694107796188234 ) ) ;
#44859=CARTESIAN_POINT ( 'NONE',  ( 1.142975459103954705, 16.61830776097024653, -2.870787844569587133 ) ) ;
#44868=CARTESIAN_POINT ( 'NONE',  ( -31.28234235046239320, -11.28615439405757392, -3.760136334089591248 ) ) ;
#44873=CARTESIAN_POINT ( 'NONE',  ( -30.25247992116029394, 39.82368563463828792, -3.760136334089591248 ) ) ;
#44877=CARTESIAN_POINT ( 'NONE',  ( 14.48769039275578407, 30.44468701195595983, 8.807470649214879543 ) ) ;
#44883=B_SPLINE_CURVE_WITH_KNOTS ( 'NONE', 3,
 ( #9045, #24196, #20332, #24700 ),
 .UNSPECIFIED., .F., .F.,
 ( 4, 4 ),
 ( 0.0001349653321192963314, 0.009897389366564843943 ),
 .UNSPECIFIED. ) ;
#44884=ORIENTED_EDGE ( 'NONE', *, *, #36055, .T. ) ;
#44885=LINE ( 'NONE', #36747, #1039 ) ;
#44892=VERTEX_POINT ( 'NONE', #29558 ) ;
#44913=CARTESIAN_POINT ( 'NONE',  ( 1.228394325311184421, -1.341866297401743235, 9.903764339332088440 ) ) ;
#44916=ADVANCED_FACE ( 'NONE', ( #13399 ), #6050, .T. ) ;
#44921=CARTESIAN_POINT ( 'NONE',  ( 16.52264463346132572, -2.779753662172757878, 9.403735324607438884 ) ) ;
#44938=CARTESIAN_POINT ( 'NONE',  ( -0.9494396179258391966, 9.954826186926261755, 9.646707543097345905 ) ) ;
#44941=CARTESIAN_POINT ( 'NONE',  ( -45.64490844644706868, -21.32281559348764333, 8.807470649214879543 ) ) ;
#44947=LINE ( 'NONE', #41132, #43826 ) ;
#44952=ADVANCED_FACE ( 'NONE', ( #23121 ), #40460, .T. ) ;
#44955=CARTESIAN_POINT ( 'NONE',  ( 30.87089393895375267, -12.69923079256617093, -9.367992836599951190 ) ) ;
#44956=CARTESIAN_POINT ( 'NONE',  ( 1.011271242968694084, -0.7347315653655782652, 3.333333333333333481 ) ) ;
#44963=ORIENTED_EDGE ( 'NONE', *, *, #32628, .F. ) ;
#44981=EDGE_CURVE ( 'NONE', #8966, #22583, #22077, .T. ) ;
#44983=VERTEX_POINT ( 'NONE', #7741 ) ;
#44992=CARTESIAN_POINT ( 'NONE',  ( 7.576114424932982594, -50.00000000000000711, 7.906207997025717304 ) ) ;
#45000=ADVANCED_FACE ( 'NONE', ( #3360 ), #26142, .T. ) ;
#45001=VECTOR ( 'NONE', #46637, 1000.000000000000000 ) ;
#45003=CARTESIAN_POINT ( 'NONE',  ( -37.27397286063865778, 4.111076158911805223, 7.697694107796192675 ) ) ;
#45005=CARTESIAN_POINT ( 'NONE',  ( -1.320835335343009787, 0.01943189458965158267, 9.943883492372876276 ) ) ;
#45011=ORIENTED_EDGE ( 'NONE', *, *, #19327, .T. ) ;
#45025=CARTESIAN_POINT ( 'NONE',  ( -17.23491422248386584, 0.5912720620001978844, 8.727788335465566760 ) ) ;
#45026=ADVANCED_FACE ( 'NONE', ( #4390 ), #42120, .T. ) ;
#45039=CARTESIAN_POINT ( 'NONE',  ( -8.277096487746778308, 33.14818118907697198, 7.455576670931136185 ) ) ;
#45040=CARTESIAN_POINT ( 'NONE',  ( 34.91952936320839740, -13.67027684621004546, -9.422646554964178023 ) ) ;
#45056=CARTESIAN_POINT ( 'NONE',  ( -0.6803378293975504976, -1.026336841997344429, 9.975326647350891918 ) ) ;
#45057=CARTESIAN_POINT ( 'NONE',  ( 36.76598589393955052, 7.383243274241862331, -8.192531242611266862 ) ) ;
#45060=CARTESIAN_POINT ( 'NONE',  ( 0.9983599181300923942, 1.124146016603553733, 9.953784399990620813 ) ) ;
#45063=CARTESIAN_POINT ( 'NONE',  ( -1.011271242968683426, -0.7347315653655928092, -3.333333333333333481 ) ) ;
#45067=VECTOR ( 'NONE', #33353, 1000.000000000000000 ) ;
#45083=VERTEX_POINT ( 'NONE', #5638 ) ;
#45114=B_SPLINE_CURVE_WITH_KNOTS ( 'NONE', 3,
 ( #21910, #25756, #6498, #30364 ),
 .UNSPECIFIED., .F., .F.,
 ( 4, 4 ),
 ( 0.000000000000000000, 0.2545280377015988194 ),
 .UNSPECIFIED. ) ;
#45119=EDGE_CURVE ( 'NONE', #8942, #27159, #109, .T. ) ;
#45124=CARTESIAN_POINT ( 'NONE',  ( -0.3910393408547386818, -3.877122853643371947, 9.741991644047244492 ) ) ;
#45125=CARTESIAN_POINT ( 'NONE',  ( -0.3862712429686895876, 1.188820645368940720, 10.00000000000000000 ) ) ;
#45131=CARTESIAN_POINT ( 'NONE',  ( 1.250000000000000222, 0.000000000000000000, 10.00000000000000000 ) ) ;
#45136=EDGE_LOOP ( 'NONE', ( #12247, #38144, #14621, #44674 ) ) ;
#45145=VERTEX_POINT ( 'NONE', #21047 ) ;
#45171=ORIENTED_EDGE ( 'NONE', *, *, #33473, .T. ) ;
#45176=CARTESIAN_POINT ( 'NONE',  ( -1.249999999999999778, 0.000000000000000000, 10.00000000000000000 ) ) ;
#45183=CARTESIAN_POINT ( 'NONE',  ( -4.763548243873389154, 16.57409059453848599, 8.727788335465566760 ) ) ;
#45185=CARTESIAN_POINT ( 'NONE',  ( -1.011271242968688533, 0.7347315653655859258, 10.00000000000000000 ) ) ;
#45191=CARTESIAN_POINT ( 'NONE',  ( -1.578643388466005160, 1.550786058692512182, 9.881002359080275355 ) ) ;
#45195=EDGE_LOOP ( 'NONE', ( #7434, #41089, #42508 ) ) ;
#45199=CARTESIAN_POINT ( 'NONE',  ( -1.655785408455817675, -0.7536129375911022610, 9.903764339332079558 ) ) ;
#45204=CARTESIAN_POINT ( 'NONE',  ( -0.6215990105957072132, 1.608617984725374983, 9.928159647716134018 ) ) ;
#45206=CARTESIAN_POINT ( 'NONE',  ( 3.695802964311526218, 9.324875653452767921, 9.390253821402620105 ) ) ;
#45217=CARTESIAN_POINT ( 'NONE',  ( 3.245329132135053474, 7.282608432884214444, -6.098637220230962441E-16 ) ) ;
#45218=CARTESIAN_POINT ( 'NONE',  ( -17.67745476136668614, -37.99701471135970365, 7.544061037322996377 ) ) ;
#45224=ADVANCED_FACE ( 'NONE', ( #10001 ), #17924, .T. ) ;
#45230=ORIENTED_EDGE ( 'NONE', *, *, #13768, .F. ) ;
#45236=EDGE_CURVE ( 'NONE', #47355, #16274, #25175, .T. ) ;
#45237=EDGE_CURVE ( 'NONE', #50500, #12617, #43519, .T. ) ;
#45241=ORIENTED_EDGE ( 'NONE', *, *, #31182, .F. ) ;
#45244=CARTESIAN_POINT ( 'NONE',  ( 3.566525152641073504, -1.569997364302916809, 9.741991644047246268 ) ) ;
#45254=B_SPLINE_SURFACE_WITH_KNOTS ( 'NONE', 3, 3, ( 
 ( #26253, #25234, #41891, #22386 ),
 ( #21633, #2871, #40883, #17536 ),
 ( #37321, #49787, #33209, #2146 ),
 ( #17791, #5728, #30352, #49032 ) ),
 .UNSPECIFIED., .F., .F., .F.,
 ( 4, 4 ),
 ( 4, 4 ),
 ( 0.000000000000000000, 1.000000000000000000 ),
 ( 0.000000000000000000, 1.000000000000000000 ),
 .UNSPECIFIED. ) ;
#45256=CARTESIAN_POINT ( 'NONE',  ( -35.51958307830761896, 12.13749199045067684, -6.568693074176341185 ) ) ;
#45269=CARTESIAN_POINT ( 'NONE',  ( 0.4426377647354858835, 1.666766018367784596, 9.928159647716132241 ) ) ;
#45270=CARTESIAN_POINT ( 'NONE',  ( 20.40054609052976531, -26.26366202847973597, -3.760136334089591248 ) ) ;
#45278=ADVANCED_FACE ( 'NONE', ( #18695 ), #22459, .T. ) ;
#45284=ORIENTED_EDGE ( 'NONE', *, *, #32022, .F. ) ;
#45289=CARTESIAN_POINT ( 'NONE',  ( 36.02002318912989409, -10.56068015588340181, -3.721387749823056090 ) ) ;
#45291=ORIENTED_EDGE ( 'NONE', *, *, #19405, .F. ) ;
#45298=CARTESIAN_POINT ( 'NONE',  ( -46.76852358249002606, 17.86468378716741512, -9.367992836599954742 ) ) ;
#45301=CARTESIAN_POINT ( 'NONE',  ( 1.782521105131670724, -0.3635605703593869920, 9.903764339332079558 ) ) ;
#45313=CARTESIAN_POINT ( 'NONE',  ( 1.250000000000000222, 0.000000000000000000, 10.00000000000000000 ) ) ;
#45323=ORIENTED_EDGE ( 'NONE', *, *, #20553, .F. ) ;
#45331=ORIENTED_EDGE ( 'NONE', *, *, #40644, .T. ) ;
#45346=ORIENTED_EDGE ( 'NONE', *, *, #4500, .F. ) ;
#45359=B_SPLINE_SURFACE_WITH_KNOTS ( 'NONE', 3, 3, ( 
 ( #45379, #5903, #2303, #29509 ),
 ( #10267, #36992, #9747, #18196 ),
 ( #44873, #44380, #49212, #14360 ),
 ( #5647, #13345, #21551, #2554 ) ),
 .UNSPECIFIED., .F., .F., .F.,
 ( 4, 4 ),
 ( 4, 4 ),
 ( 0.000000000000000000, 1.000000000000000000 ),
 ( 0.000000000000000000, 1.000000000000000000 ),
 .UNSPECIFIED. ) ;
#45370=CARTESIAN_POINT ( 'NONE',  ( 44.34968358615004291, 11.74141640735454928, -9.367992836599951190 ) ) ;
#45371=EDGE_CURVE ( 'NONE', #23745, #9096, #45907, .T. ) ;
#45377=CARTESIAN_POINT ( 'NONE',  ( 1.280882217648804167, -0.5301415400443709736, 9.960033073700794048 ) ) ;
#45379=CARTESIAN_POINT ( 'NONE',  ( -36.08557433729205144, 35.58569447144795816, 7.455576670931136185 ) ) ;
#45400=CARTESIAN_POINT ( 'NONE',  ( -1.540662627795934769, 1.371465786296043765, 9.894754715216725671 ) ) ;
#45407=CARTESIAN_POINT ( 'NONE',  ( 1.424123654779712922, 0.3625862473308184009, 9.958264684458541183 ) ) ;
#45410=CARTESIAN_POINT ( 'NONE',  ( -50.11058929355266400, 7.578863168071933387, 7.455576670931136185 ) ) ;
#45415=VERTEX_POINT ( 'NONE', #43315 ) ;
#45419=CARTESIAN_POINT ( 'NONE',  ( 6.619412807845094449, -7.495556955913033725, 9.646707543097347681 ) ) ;
#45424=ORIENTED_EDGE ( 'NONE', *, *, #43790, .T. ) ;
#45437=CARTESIAN_POINT ( 'NONE',  ( 0.3370904143228959926, -0.2449105217885284291, 10.00000000000000000 ) ) ;
#45442=ORIENTED_EDGE ( 'NONE', *, *, #42536, .F. ) ;
#45443=EDGE_CURVE ( 'NONE', #16274, #11814, #39238, .T. ) ;
#45448=CARTESIAN_POINT ( 'NONE',  ( -0.6108107228405769140, 1.056024183042602482, 9.963925895596188909 ) ) ;
#45459=CARTESIAN_POINT ( 'NONE',  ( 15.39115647749017590, -6.484697992489784291, -9.458680755252684591 ) ) ;
#45462=DIRECTION ( 'NONE',  ( -0.000000000000000000, -0.000000000000000000, -1.000000000000000000 ) ) ;
#45467=CARTESIAN_POINT ( 'NONE',  ( -5.930385588435886923, 41.38048276556310157, 8.846626183609801686 ) ) ;
#45468=CARTESIAN_POINT ( 'NONE',  ( 16.02661358026014327, 4.530191650547718218, -9.683996418299976483 ) ) ;
#45485=B_SPLINE_CURVE_WITH_KNOTS ( 'NONE', 3,
 ( #32765, #47609, #24064, #36380 ),
 .UNSPECIFIED., .F., .F.,
 ( 4, 4 ),
 ( 0.0001535465953326492635, 0.0005837444810832899313 ),
 .UNSPECIFIED. ) ;
#45486=AXIS2_PLACEMENT_3D ( 'NONE', #31923, #7813, #35026 ) ;
#45490=CARTESIAN_POINT ( 'NONE',  ( -1.104345476778524349, -0.6507740520594079703, 9.967237415621761798 ) ) ;
#45509=CARTESIAN_POINT ( 'NONE',  ( -15.45175104485246820, 6.222373774239106758, -2.870787844569587133 ) ) ;
#45510=B_SPLINE_CURVE_WITH_KNOTS ( 'NONE', 3,
 ( #41229, #6084, #37415, #29684 ),
 .UNSPECIFIED., .F., .F.,
 ( 4, 4 ),
 ( 3.471140604459641645E-18, 8.326314924909149835E-06 ),
 .UNSPECIFIED. ) ;
#45515=CARTESIAN_POINT ( 'NONE',  ( -0.5107275442771143092, -1.175643901748072873, 9.976582533991681601 ) ) ;
#45516=CARTESIAN_POINT ( 'NONE',  ( 7.576114424932982594, -50.00000000000000711, 7.906207997025717304 ) ) ;
#45517=EDGE_CURVE ( 'NONE', #19482, #6581, #688, .T. ) ;
#45524=CARTESIAN_POINT ( 'NONE',  ( -14.29087950072019098, -9.652079258044555132, 8.727788335465566760 ) ) ;
#45526=CARTESIAN_POINT ( 'NONE',  ( 13.59579750444771307, -10.60877755095900632, 8.727788335465566760 ) ) ;
#45527=ORIENTED_EDGE ( 'NONE', *, *, #29276, .T. ) ;
#45530=ORIENTED_EDGE ( 'NONE', *, *, #11868, .T. ) ;
#45536=CARTESIAN_POINT ( 'NONE',  ( 7.576114424932982594, -33.14742743729794938, 7.906207997025717304 ) ) ;
#45542=CARTESIAN_POINT ( 'NONE',  ( 50.11058929355270664, -7.578863168071591438, 7.455576670931136185 ) ) ;
#45543=CARTESIAN_POINT ( 'NONE',  ( 22.69295089195473736, 45.31600496604706052, 7.455576670931136185 ) ) ;
#45546=CARTESIAN_POINT ( 'NONE',  ( 4.672045878990125800, -50.00000000000000711, 1.847720168420772691 ) ) ;
#45553=CARTESIAN_POINT ( 'NONE',  ( -15.62858259096117841, 5.755205073598721910, -9.683996418299976483 ) ) ;
#45575=CARTESIAN_POINT ( 'NONE',  ( -3.222683565149130569, -0.4845875505058497290, 9.799352050262461589 ) ) ;
#45578=CARTESIAN_POINT ( 'NONE',  ( -44.99506233596265048, -23.32283626942287569, 7.455576670931136185 ) ) ;
#45601=CARTESIAN_POINT ( 'NONE',  ( 15.00099850811936264, 7.462898891544210933, 9.403735324607438884 ) ) ;
#45607=CARTESIAN_POINT ( 'NONE',  ( -1.011271242968677875, -0.7347315653656004697, 10.00000000000000000 ) ) ;
#45629=CARTESIAN_POINT ( 'NONE',  ( -0.3896797354171960270, 1.262193838292709147, 9.943883492372847854 ) ) ;
#45635=VERTEX_POINT ( 'NONE', #37922 ) ;
#45636=DIRECTION ( 'NONE',  ( -0.1671032855531317807, -0.5142910309547739089, 0.8411784753765542133 ) ) ;
#45638=CARTESIAN_POINT ( 'NONE',  ( 5.888214538810389698, 16.20866436362417673, 8.727788335465566760 ) ) ;
#45639=CARTESIAN_POINT ( 'NONE',  ( 0.3862712429686727678, 1.188820645368945605, 10.00000000000000000 ) ) ;
#45643=ORIENTED_EDGE ( 'NONE', *, *, #24583, .T. ) ;
#45644=FACE_OUTER_BOUND ( 'NONE', #49984, .T. ) ;
#45646=VERTEX_POINT ( 'NONE', #50147 ) ;
#45660=B_SPLINE_CURVE_WITH_KNOTS ( 'NONE', 3,
 ( #40566, #40317, #21823, #21059 ),
 .UNSPECIFIED., .F., .F.,
 ( 4, 4 ),
 ( 1.084202172485504627E-18, 0.0002708531562908071634 ),
 .UNSPECIFIED. ) ;
#45665=EDGE_CURVE ( 'NONE', #25205, #37687, #15962, .T. ) ;
#45668=CARTESIAN_POINT ( 'NONE',  ( -0.8282505383454070724, -1.889063466747028297, 9.894754715216727448 ) ) ;
#45674=B_SPLINE_SURFACE_WITH_KNOTS ( 'NONE', 3, 3, ( 
 ( #7068, #6312, #6805, #10407 ),
 ( #26058, #41706, #22209, #19368 ),
 ( #34793, #47032, #15279, #16284 ),
 ( #7838, #15766, #8087, #27325 ) ),
 .UNSPECIFIED., .F., .F., .F.,
 ( 4, 4 ),
 ( 4, 4 ),
 ( 0.000000000000000000, 1.000000000000000000 ),
 ( 0.000000000000000000, 1.000000000000000000 ),
 .UNSPECIFIED. ) ;
#45677=FACE_OUTER_BOUND ( 'NONE', #6999, .T. ) ;
#45678=CARTESIAN_POINT ( 'NONE',  ( -8.813458710706198573, -4.724716452304520864, 0.000000000000000000 ) ) ;
#45712=DIRECTION ( 'NONE',  ( -0.000000000000000000, -0.000000000000000000, -1.000000000000000000 ) ) ;
#45715=CARTESIAN_POINT ( 'NONE',  ( -6.174150299305392053, 45.68101107938186800, 8.807470649214879543 ) ) ;
#45736=CARTESIAN_POINT ( 'NONE',  ( -0.3862712429686895876, 1.188820645368940720, 10.00000000000000000 ) ) ;
#45743=CARTESIAN_POINT ( 'NONE',  ( 1.540526284687965264, -1.371707213411490267, 9.886433018048071730 ) ) ;
#45744=DIRECTION ( 'NONE',  ( -0.9510565162951500895, -0.3090169943749582759, 0.000000000000000000 ) ) ;
#45764=B_SPLINE_CURVE_WITH_KNOTS ( 'NONE', 3,
 ( #29834, #14940, #30593, #14679 ),
 .UNSPECIFIED., .F., .F.,
 ( 4, 4 ),
 ( 0.9890644561682323532, 1.000000000000000000 ),
 .UNSPECIFIED. ) ;
#45770=CARTESIAN_POINT ( 'NONE',  ( -0.3370904143228963812, 0.2449105217885287067, 10.00000000000000000 ) ) ;
#45774=B_SPLINE_SURFACE_WITH_KNOTS ( 'NONE', 3, 3, ( 
 ( #15085, #6370, #7140, #29984 ),
 ( #6623, #41769, #22278, #34592 ),
 ( #10981, #22017, #18164, #33844 ),
 ( #2767, #38209, #22779, #38699 ) ),
 .UNSPECIFIED., .F., .F., .F.,
 ( 4, 4 ),
 ( 4, 4 ),
 ( 0.000000000000000000, 1.000000000000000000 ),
 ( 0.000000000000000000, 1.000000000000000000 ),
 .UNSPECIFIED. ) ;
#45776=CARTESIAN_POINT ( 'NONE',  ( -0.7547693905867810527, -1.149888081716692545, 9.972175347158279024 ) ) ;
#45801=ORIENTED_EDGE ( 'NONE', *, *, #9505, .F. ) ;
#45804=CARTESIAN_POINT ( 'NONE',  ( -4.641001526964560142, -33.28196331604080171, -8.016098858316199838 ) ) ;
#45806=CARTESIAN_POINT ( 'NONE',  ( 24.47767542868285062, -23.18653802921781448, 8.807470649214879543 ) ) ;
#45812=ORIENTED_EDGE ( 'NONE', *, *, #10516, .T. ) ;
#45813=CARTESIAN_POINT ( 'NONE',  ( 1.011271242968677653, 0.7347315653656002477, -3.333333333333333481 ) ) ;
#45814=CARTESIAN_POINT ( 'NONE',  ( -45.64490844644706868, -21.32281559348764333, 8.807470649214879543 ) ) ;
#45843=ADVANCED_FACE ( 'NONE', ( #37110 ), #30677, .T. ) ;
#45853=CARTESIAN_POINT ( 'NONE',  ( 18.67411147745603373, 27.51799019669827473, -3.760136334089591248 ) ) ;
#45856=AXIS2_PLACEMENT_3D ( 'NONE', #9589, #32961, #48540 ) ;
#45858=DIRECTION ( 'NONE',  ( 0.4374820812098816902, 0.3178493372392748872, -0.8411784753765541023 ) ) ;
#45860=CARTESIAN_POINT ( 'NONE',  ( 1.962539651752403413, -0.2571568065648505708, 9.897807938190497978 ) ) ;
#45862=DIRECTION ( 'NONE',  ( -0.000000000000000000, -0.000000000000000000, -1.000000000000000000 ) ) ;
#45884=CARTESIAN_POINT ( 'NONE',  ( 30.87089393895375267, -12.69923079256617449, -9.367992836599954742 ) ) ;
#45885=CARTESIAN_POINT ( 'NONE',  ( 1.377636575563020438, -0.6021164824561170414, 9.953784399990622589 ) ) ;
#45889=VERTEX_POINT ( 'NONE', #5527 ) ;
#45907=B_SPLINE_CURVE_WITH_KNOTS ( 'NONE', 3,
 ( #4587, #23578, #27937, #31797, #12523, #27682 ),
 .UNSPECIFIED., .F., .F.,
 ( 4, 2, 4 ),
 ( 4.171459933175973117E-17, 0.009882509389272368938, 0.01976501877854469277 ),
 .UNSPECIFIED. ) ;
#45909=CARTESIAN_POINT ( 'NONE',  ( 0.5107275442771160856, 1.175643901748075537, 9.976582533991678048 ) ) ;
#45913=CARTESIAN_POINT ( 'NONE',  ( -17.23491422248386584, 0.5912720620001978844, 8.727788335465566760 ) ) ;
#45919=CARTESIAN_POINT ( 'NONE',  ( 0.2778388845795309314, -1.251314014313100520, 9.976582533991681601 ) ) ;
#45924=CARTESIAN_POINT ( 'NONE',  ( 24.47767542868285062, -23.18653802921781448, 8.807470649214879543 ) ) ;
#45937=CARTESIAN_POINT ( 'NONE',  ( -1.780432407520014415, -1.041450996408466612, 9.894754715216725671 ) ) ;
#45942=CARTESIAN_POINT ( 'NONE',  ( 0.4612311909458165493, -1.380801828344328186, 9.938560165450807560 ) ) ;
#45944=CARTESIAN_POINT ( 'NONE',  ( 5.888214538810389698, 16.20866436362417673, 8.727788335465566760 ) ) ;
#45949=CARTESIAN_POINT ( 'NONE',  ( 0.8433491450857230065, -0.9182416014173362395, 9.981352469109934233 ) ) ;
#45955=CARTESIAN_POINT ( 'NONE',  ( -0.6108107228405769140, 1.056024183042602482, 9.963925895596188909 ) ) ;
#45960=ORIENTED_EDGE ( 'NONE', *, *, #41485, .F. ) ;
#45961=EDGE_CURVE ( 'NONE', #37083, #44030, #19030, .T. ) ;
#45962=CARTESIAN_POINT ( 'NONE',  ( -1.193089574352124149, -0.2545860991493743564, 9.963925895596188909 ) ) ;
#45979=ORIENTED_EDGE ( 'NONE', *, *, #41861, .F. ) ;
#45983=CARTESIAN_POINT ( 'NONE',  ( -2.538055338523177440, -33.28424297489108596, -9.367992836599954742 ) ) ;
#45996=CARTESIAN_POINT ( 'NONE',  ( 2.216591765713427975, -1.436486588195951430, 9.847478953136990398 ) ) ;
#45997=CARTESIAN_POINT ( 'NONE',  ( 1.011271242968694084, -0.7347315653655782652, 10.00000000000000000 ) ) ;
#46003=ORIENTED_EDGE ( 'NONE', *, *, #50041, .T. ) ;
#46007=EDGE_CURVE ( 'NONE', #50249, #34526, #28238, .T. ) ;
#46014=EDGE_CURVE ( 'NONE', #44030, #43044, #4958, .T. ) ;
#46018=CARTESIAN_POINT ( 'NONE',  ( 10.70590866674922204, -12.76446523155706814, -3.546734833711462365 ) ) ;
#46019=CARTESIAN_POINT ( 'NONE',  ( -12.78770032058971395, -31.68259716188267916, 7.455576670931136185 ) ) ;
#46024=CARTESIAN_POINT ( 'NONE',  ( -8.277096487746778308, 50.00000000000000711, 7.455576670931136185 ) ) ;
#46026=CARTESIAN_POINT ( 'NONE',  ( -0.09523839817533703844, -1.466467394240187350, 9.958264684458541183 ) ) ;
#46027=CARTESIAN_POINT ( 'NONE',  ( 0.4692401618441018885, 1.180027720800731039, 9.975314328424618182 ) ) ;
#46037=CARTESIAN_POINT ( 'NONE',  ( -1.540662627795934769, 1.371465786296043765, 9.894754715216725671 ) ) ;
#46049=CARTESIAN_POINT ( 'NONE',  ( 47.22310614333766665, 16.46562252335956344, -3.760136334089591248 ) ) ;
#46060=CARTESIAN_POINT ( 'NONE',  ( 1.133908876584335257, 0.5183204401656757998, 9.981352469109932457 ) ) ;
#46061=CARTESIAN_POINT ( 'NONE',  ( 32.43949840348898306, 7.871562655726503266, -9.367992836599951190 ) ) ;
#46066=CARTESIAN_POINT ( 'NONE',  ( 2.462075149652696027, -16.57295996686994499, 9.403735324607438884 ) ) ;
#46068=CARTESIAN_POINT ( 'NONE',  ( 2.945500763482279627, 16.64098165802040086, -9.008049429158100807 ) ) ;
#46069=CARTESIAN_POINT ( 'NONE',  ( 0.2773062244624638351, -1.251557370488896481, 9.948547179989619238 ) ) ;
#46081=B_SPLINE_SURFACE_WITH_KNOTS ( 'NONE', 3, 3, ( 
 ( #47078, #18894, #46068, #23782 ),
 ( #19152, #4284, #50671, #19918 ),
 ( #11468, #7373, #35604, #38941 ),
 ( #16082, #10959, #26614, #42259 ) ),
 .UNSPECIFIED., .F., .F., .F.,
 ( 4, 4 ),
 ( 4, 4 ),
 ( 0.000000000000000000, 1.000000000000000000 ),
 ( 0.000000000000000000, 1.000000000000000000 ),
 .UNSPECIFIED. ) ;
#46090=CARTESIAN_POINT ( 'NONE',  ( 0.3656201545664388708, -2.182515578491310393, 9.881002359080277131 ) ) ;
#46091=ORIENTED_EDGE ( 'NONE', *, *, #38576, .T. ) ;
#46102=ORIENTED_EDGE ( 'NONE', *, *, #40644, .F. ) ;
#46111=CARTESIAN_POINT ( 'NONE',  ( -6.174150299305392053, 33.14591993373988998, 8.807470649214879543 ) ) ;
#46115=CARTESIAN_POINT ( 'NONE',  ( 18.69789054174343690, -27.49790346457731616, -2.408242355805840784 ) ) ;
#46127=CARTESIAN_POINT ( 'NONE',  ( -4.763548243873389154, 16.57409059453848599, 8.727788335465566760 ) ) ;
#46142=B_SPLINE_CURVE_WITH_KNOTS ( 'NONE', 3,
 ( #30425, #46027, #42218, #22718 ),
 .UNSPECIFIED., .F., .F.,
 ( 4, 4 ),
 ( 0.000000000000000000, 0.0001252128669263239205 ),
 .UNSPECIFIED. ) ;
#46151=ORIENTED_EDGE ( 'NONE', *, *, #33212, .T. ) ;
#46153=ORIENTED_EDGE ( 'NONE', *, *, #19040, .T. ) ;
#46154=CARTESIAN_POINT ( 'NONE',  ( 1.173396789973004228, 0.3425192899591110729, 9.969517326150317160 ) ) ;
#46161=CARTESIAN_POINT ( 'NONE',  ( 41.53730588968647197, 19.98817461849979793, 8.807470649214879543 ) ) ;
#46164=CARTESIAN_POINT ( 'NONE',  ( -0.2827943264366573617, 6.852167361307234472, 9.753789706659947711 ) ) ;
#46170=CARTESIAN_POINT ( 'NONE',  ( 0.9390173899407876501, 1.130417317737878458, 9.958264684458711713 ) ) ;
#46171=AXIS2_PLACEMENT_3D ( 'NONE', #12071, #31584, #16413 ) ;
#46175=CARTESIAN_POINT ( 'NONE',  ( -1.011271242968683426, -0.7347315653655928092, 10.00000000000000000 ) ) ;
#46178=ORIENTED_EDGE ( 'NONE', *, *, #39172, .F. ) ;
#46186=EDGE_CURVE ( 'NONE', #35077, #31351, #40414, .T. ) ;
#46193=EDGE_CURVE ( 'NONE', #26846, #36961, #19581, .T. ) ;
#46194=B_SPLINE_SURFACE_WITH_KNOTS ( 'NONE', 3, 3, ( 
 ( #46237, #30898, #42410, #10865 ),
 ( #34489, #7028, #26526, #14975 ),
 ( #35014, #38852, #18557, #46484 ),
 ( #50580, #45983, #50066, #42922 ) ),
 .UNSPECIFIED., .F., .F., .F.,
 ( 4, 4 ),
 ( 4, 4 ),
 ( 0.000000000000000000, 1.000000000000000000 ),
 ( 0.000000000000000000, 1.000000000000000000 ),
 .UNSPECIFIED. ) ;
#46195=CARTESIAN_POINT ( 'NONE',  ( 1.270843316669197254, -0.6654759734677784255, 9.950105812514292936 ) ) ;
#46212=ADVANCED_FACE ( 'NONE', ( #29257 ), #45359, .T. ) ;
#46220=ADVANCED_FACE ( 'NONE', ( #48458 ), #49022, .T. ) ;
#46224=EDGE_CURVE ( 'NONE', #22583, #12326, #42836, .T. ) ;
#46230=ORIENTED_EDGE ( 'NONE', *, *, #29770, .F. ) ;
#46237=CARTESIAN_POINT ( 'NONE',  ( 8.277096487746778308, -50.00000000000000711, 7.455576670931136185 ) ) ;
#46244=CARTESIAN_POINT ( 'NONE',  ( -44.99506233596265048, -23.32283626942287569, 7.455576670931136185 ) ) ;
#46249=CARTESIAN_POINT ( 'NONE',  ( -11.73320209285699889, 11.96063479729179768, 9.403735324607438884 ) ) ;
#46251=CARTESIAN_POINT ( 'NONE',  ( -50.11058929355266400, 7.578863168071933387, 7.455576670931136185 ) ) ;
#46258=CARTESIAN_POINT ( 'NONE',  ( -2.097937730060984052, 0.2450639578955122744, 9.884520316594375799 ) ) ;
#46259=CARTESIAN_POINT ( 'NONE',  ( -49.46074318306826001, 9.578883844007169301, 8.807470649214879543 ) ) ;
#46262=CARTESIAN_POINT ( 'NONE',  ( -44.99506233596265048, -23.32283626942287569, 7.455576670931136185 ) ) ;
#46277=CARTESIAN_POINT ( 'NONE',  ( 6.174150299305392053, -33.14591993373988998, 8.807470649214879543 ) ) ;
#46294=EDGE_CURVE ( 'NONE', #50289, #3893, #3679, .T. ) ;
#46309=B_SPLINE_CURVE_WITH_KNOTS ( 'NONE', 3,
 ( #11023, #29515, #18202, #49218 ),
 .UNSPECIFIED., .F., .F.,
 ( 4, 4 ),
 ( 0.01005345353272254355, 0.01006177981554775419 ),
 .UNSPECIFIED. ) ;
#46317=CARTESIAN_POINT ( 'NONE',  ( 6.174150299305392053, -33.14591993373988998, 8.807470649214879543 ) ) ;
#46332=CARTESIAN_POINT ( 'NONE',  ( 1.011271242968688311, -0.7347315653655855927, 10.00000000000000000 ) ) ;
#46334=CARTESIAN_POINT ( 'NONE',  ( -1.011271242968683426, -0.7347315653655928092, 10.00000000000000000 ) ) ;
#46342=CARTESIAN_POINT ( 'NONE',  ( 4.641001526964561918, 33.28196331604080171, -8.016098858316205167 ) ) ;
#46343=CARTESIAN_POINT ( 'NONE',  ( -0.1265591857321690383, -1.213367045380180809, 9.963925895596192461 ) ) ;
#46344=CARTESIAN_POINT ( 'NONE',  ( 25.08868538179583396, -27.91927157928032699, 6.057468652304065060 ) ) ;
#46346=CARTESIAN_POINT ( 'NONE',  ( -30.22736451279196856, -39.84193304692609416, -2.408242355805840784 ) ) ;
#46361=EDGE_CURVE ( 'NONE', #2701, #36062, #25682, .T. ) ;
#46365=ORIENTED_EDGE ( 'NONE', *, *, #22040, .T. ) ;
#46366=CARTESIAN_POINT ( 'NONE',  ( -8.569579719062554446, -5.179646911086122962, 3.092310436554649655 ) ) ;
#46371=ORIENTED_EDGE ( 'NONE', *, *, #47630, .F. ) ;
#46378=CARTESIAN_POINT ( 'NONE',  ( -0.4692401618441021660, -1.180027720800729041, 9.975314328424614629 ) ) ;
#46381=CARTESIAN_POINT ( 'NONE',  ( -1.249999999999999778, 0.000000000000000000, 10.00000000000000000 ) ) ;
#46386=CARTESIAN_POINT ( 'NONE',  ( -18.67411147745623978, -27.51799019669813973, -3.760136334089591248 ) ) ;
#46390=B_SPLINE_CURVE_WITH_KNOTS ( 'NONE', 3,
 ( #49734, #41834, #21844, #45400 ),
 .UNSPECIFIED., .F., .F.,
 ( 4, 4 ),
 ( 0.0009679537044786268220, 0.001281751046851330568 ),
 .UNSPECIFIED. ) ;
#46394=CARTESIAN_POINT ( 'NONE',  ( 1.184758822850214388, -0.8459872530593102180, 9.938560165450805783 ) ) ;
#46396=CARTESIAN_POINT ( 'NONE',  ( -1.377636575563021992, 0.6021164824561227036, 9.953784399990620813 ) ) ;
#46402=CARTESIAN_POINT ( 'NONE',  ( -0.3862712429686729343, -1.188820645368946050, 10.00000000000000000 ) ) ;
#46406=B_SPLINE_CURVE_WITH_KNOTS ( 'NONE', 3,
 ( #45003, #29634, #37112, #20933, #45256, #9131 ),
 .UNSPECIFIED., .F., .F.,
 ( 4, 2, 4 ),
 ( 4.943961906533900219E-17, 0.009882509389272372408, 0.01976501877854469624 ),
 .UNSPECIFIED. ) ;
#46411=VERTEX_POINT ( 'NONE', #12280 ) ;
#46415=CARTESIAN_POINT ( 'NONE',  ( -1.011271242968683426, -0.7347315653655928092, -10.00000000000000000 ) ) ;
#46421=PLANE ( 'NONE',  #30518 ) ;
#46435=CARTESIAN_POINT ( 'NONE',  ( 34.08355720199905647, -2.371364769369109116, 7.455576670931136185 ) ) ;
#46436=CARTESIAN_POINT ( 'NONE',  ( -24.47767542868268364, 23.18653802921800278, 8.807470649214879543 ) ) ;
#46438=ORIENTED_EDGE ( 'NONE', *, *, #16412, .F. ) ;
#46445=CARTESIAN_POINT ( 'NONE',  ( 7.359817328027030925, 15.16751262232805431, 2.590526750877053086 ) ) ;
#46456=CARTESIAN_POINT ( 'NONE',  ( -7.749480817862350435, -14.85497772329513211, 9.403735324607438884 ) ) ;
#46476=VERTEX_POINT ( 'NONE', #20485 ) ;
#46480=CARTESIAN_POINT ( 'NONE',  ( 0.3862712429686894766, -1.188820645368940276, -10.00000000000000000 ) ) ;
#46484=CARTESIAN_POINT ( 'NONE',  ( 1.249999999999999778, -0.000000000000000000, -3.333333333333333481 ) ) ;
#46499=CARTESIAN_POINT ( 'NONE',  ( -0.3862712429686809279, -1.188820645368943163, -10.00000000000000000 ) ) ;
#46506=CARTESIAN_POINT ( 'NONE',  ( -2.188678504086925880, 0.3267089737526900350, 9.881002359080270026 ) ) ;
#46507=B_SPLINE_SURFACE_WITH_KNOTS ( 'NONE', 3, 3, ( 
 ( #23874, #36193, #23615, #15662 ),
 ( #19498, #46922, #35186, #542 ),
 ( #35441, #12563, #43864, #4631 ),
 ( #31331, #43116, #11825, #4121 ) ),
 .UNSPECIFIED., .F., .F., .F.,
 ( 4, 4 ),
 ( 4, 4 ),
 ( 0.000000000000000000, 1.000000000000000000 ),
 ( 0.000000000000000000, 1.000000000000000000 ),
 .UNSPECIFIED. ) ;
#46509=CARTESIAN_POINT ( 'NONE',  ( -15.98719783915689163, 4.501063718205989161, 3.266473740018926541 ) ) ;
#46530=CARTESIAN_POINT ( 'NONE',  ( 4.395207584381303434, 3.942437227415936718, 9.586754400234161366 ) ) ;
#46531=CARTESIAN_POINT ( 'NONE',  ( 3.229232847726260403, -16.57333684275945629, 9.178419661560148768 ) ) ;
#46534=ADVANCED_FACE ( 'NONE', ( #16903 ), #17524, .T. ) ;
#46536=CARTESIAN_POINT ( 'NONE',  ( 0.1287570809895660084, -0.3962735484563127408, 10.00000000000000000 ) ) ;
#46537=CARTESIAN_POINT ( 'NONE',  ( 34.38425513258721367, -36.82177522737821107, 8.807470649214879543 ) ) ;
#46546=CARTESIAN_POINT ( 'NONE',  ( 22.51959565330788493, 30.03043964857266346, -6.568693074176341185 ) ) ;
#46557=( NAMED_UNIT ( * ) SI_UNIT ( $, .STERADIAN. ) SOLID_ANGLE_UNIT ( ) );
#46564=CARTESIAN_POINT ( 'NONE',  ( 9.260964247899973856, -13.84230907185609460, -9.683996418299976483 ) ) ;
#46566=CARTESIAN_POINT ( 'NONE',  ( 34.08406891383362591, -15.63733501198463038, -8.192531242611266862 ) ) ;
#46572=EDGE_CURVE ( 'NONE', #50186, #9851, #24915, .T. ) ;
#46574=CARTESIAN_POINT ( 'NONE',  ( 1.011271242968677653, 0.7347315653656002477, 3.333333333333333481 ) ) ;
#46585=CARTESIAN_POINT ( 'NONE',  ( -0.9942667885118393611, 0.7728247605419426014, 9.974012008644018934 ) ) ;
#46591=CARTESIAN_POINT ( 'NONE',  ( -0.2778388845795317086, 1.251314014313103851, 9.976582533991678048 ) ) ;
#46605=DIRECTION ( 'NONE',  ( 0.5407575913134976542, 0.000000000000000000, -0.8411784753765542133 ) ) ;
#46608=CARTESIAN_POINT ( 'NONE',  ( -9.907356528110963012, 1.358045148327947427, 0.000000000000000000 ) ) ;
#46617=CARTESIAN_POINT ( 'NONE',  ( -34.38425513258694366, 36.82177522737846687, 8.807470649214879543 ) ) ;
#46619=CARTESIAN_POINT ( 'NONE',  ( 0.3334286742302847717, 1.332255019526881412, 9.946805383069621698 ) ) ;
#46621=CARTESIAN_POINT ( 'NONE',  ( 9.998889670239195837, 0.1490146381531976816, 9.282506307616472441 ) ) ;
#46625=EDGE_LOOP ( 'NONE', ( #1520, #30122, #45346, #46738 ) ) ;
#46634=ORIENTED_EDGE ( 'NONE', *, *, #42492, .T. ) ;
#46637=DIRECTION ( 'NONE',  ( 0.8090169943749465631, 0.5877852522924742473, 0.000000000000000000 ) ) ;
#46639=FACE_OUTER_BOUND ( 'NONE', #19494, .T. ) ;
#46662=CARTESIAN_POINT ( 'NONE',  ( -36.08557433729205144, 35.58569447144795816, 7.455576670931136185 ) ) ;
#46663=CARTESIAN_POINT ( 'NONE',  ( -1.424123654778022274, -0.3625862473323341328, 9.958264684458713489 ) ) ;
#46688=CARTESIAN_POINT ( 'NONE',  ( -6.508636631827791064, -15.75743548351446854, 8.953103998512858652 ) ) ;
#46699=CARTESIAN_POINT ( 'NONE',  ( 34.66007756064423972, -14.33302383662588930, -9.011255500499645521 ) ) ;
#46702=EDGE_LOOP ( 'NONE', ( #4463, #15474, #48460, #10501, #14082 ) ) ;
#46704=ORIENTED_EDGE ( 'NONE', *, *, #45665, .T. ) ;
#46711=CARTESIAN_POINT ( 'NONE',  ( 25.60949810002064098, 43.19700938445193827, 1.847720168420772691 ) ) ;
#46731=CARTESIAN_POINT ( 'NONE',  ( -0.03371980368972005843, -1.221991649883341413, 9.987567862361071747 ) ) ;
#46738=ORIENTED_EDGE ( 'NONE', *, *, #48845, .T. ) ;
#46742=CARTESIAN_POINT ( 'NONE',  ( -36.76598589393961447, -7.383243274241610088, -8.192531242611266862 ) ) ;
#46754=CARTESIAN_POINT ( 'NONE',  ( 1.249999999999999778, 0.000000000000000000, 10.00000000000000000 ) ) ;
#46759=CARTESIAN_POINT ( 'NONE',  ( -0.3862712429686895876, 1.188820645368940720, -10.00000000000000000 ) ) ;
#46763=EDGE_CURVE ( 'NONE', #37083, #4452, #42203, .T. ) ;
#46779=CARTESIAN_POINT ( 'NONE',  ( -1.066995270233474624, 50.00000000000000711, -3.760136334089591248 ) ) ;
#46784=CARTESIAN_POINT ( 'NONE',  ( -7.576114424932982594, 50.00000000000000711, 7.906207997025717304 ) ) ;
#46785=CARTESIAN_POINT ( 'NONE',  ( -8.277096487746778308, 33.14818118907697198, 7.455576670931136185 ) ) ;
#46789=ORIENTED_EDGE ( 'NONE', *, *, #38254, .T. ) ;
#46798=CARTESIAN_POINT ( 'NONE',  ( 1.170973275723889095, 0.8656725377797501730, 9.938543673150057600 ) ) ;
#46800=CARTESIAN_POINT ( 'NONE',  ( -1.184758822850544568, 0.8459872530594374496, 9.938560165450795125 ) ) ;
#46805=CARTESIAN_POINT ( 'NONE',  ( 1.780619886013945052, 1.041246721325614466, 9.886433018048068178 ) ) ;
#46809=ORIENTED_EDGE ( 'NONE', *, *, #44153, .F. ) ;
#46810=ORIENTED_EDGE ( 'NONE', *, *, #11158, .F. ) ;
#46823=CARTESIAN_POINT ( 'NONE',  ( 16.16402646813543242, -4.033894069732437693, -3.546734833711462365 ) ) ;
#46825=B_SPLINE_CURVE_WITH_KNOTS ( 'NONE', 3,
 ( #29990, #15850, #43033, #23030 ),
 .UNSPECIFIED., .F., .F.,
 ( 4, 4 ),
 ( 8.824766327896537836E-19, 0.002040833422559265500 ),
 .UNSPECIFIED. ) ;
#46833=VERTEX_POINT ( 'NONE', #44483 ) ;
#46852=EDGE_CURVE ( 'NONE', #49565, #49290, #11597, .T. ) ;
#46858=ORIENTED_EDGE ( 'NONE', *, *, #27218, .T. ) ;
#46860=CARTESIAN_POINT ( 'NONE',  ( 0.3370904143228924954, 0.2449105217885333141, 10.00000000000000000 ) ) ;
#46862=ORIENTED_EDGE ( 'NONE', *, *, #34991, .F. ) ;
#46872=CARTESIAN_POINT ( 'NONE',  ( -48.98697415750977058, -11.03699497439218291, -8.016098858316205167 ) ) ;
#46886=EDGE_CURVE ( 'NONE', #1823, #42650, #40944, .T. ) ;
#46889=CARTESIAN_POINT ( 'NONE',  ( -34.08406891383351933, 15.63733501198486309, -8.192531242611266862 ) ) ;
#46894=CARTESIAN_POINT ( 'NONE',  ( -16.52264463346130796, 2.779753662172870232, 9.403735324607438884 ) ) ;
#46912=DIRECTION ( 'NONE',  ( -1.000000000000000000, 0.000000000000000000, -0.000000000000000000 ) ) ;
#46922=CARTESIAN_POINT ( 'NONE',  ( -1.035950918207909632, -33.23661552194049307, -2.408242355805840784 ) ) ;
#46928=B_SPLINE_SURFACE_WITH_KNOTS ( 'NONE', 3, 3, ( 
 ( #39728, #4564, #20213, #4799 ),
 ( #712, #16362, #43802, #27157 ),
 ( #23291, #35131, #50709, #46860 ),
 ( #11757, #7923, #23561, #219 ) ),
 .UNSPECIFIED., .F., .F., .F.,
 ( 4, 4 ),
 ( 4, 4 ),
 ( 0.000000000000000000, 1.000000000000000000 ),
 ( 0.000000000000000000, 1.000000000000000000 ),
 .UNSPECIFIED. ) ;
#46937=CARTESIAN_POINT ( 'NONE',  ( -23.82716369509181575, -44.49195112875988656, 8.356839323120299312 ) ) ;
#46938=CARTESIAN_POINT ( 'NONE',  ( -2.052581215100349521, 0.2042358160481012597, 9.886433018048073507 ) ) ;
#46940=CARTESIAN_POINT ( 'NONE',  ( -1.011271242968683426, -0.7347315653655928092, 10.00000000000000000 ) ) ;
#46951=FACE_OUTER_BOUND ( 'NONE', #9968, .T. ) ;
#46974=CARTESIAN_POINT ( 'NONE',  ( 3.808200756227633654, 0.8261963378076531139, 9.741991644047248045 ) ) ;
#46990=CARTESIAN_POINT ( 'NONE',  ( 0.3862712429686894766, -1.188820645368940276, -3.333333333333333481 ) ) ;
#46997=VERTEX_POINT ( 'NONE', #31374 ) ;
#47004=ORIENTED_EDGE ( 'NONE', *, *, #5259, .F. ) ;
#47012=CARTESIAN_POINT ( 'NONE',  ( 1.066995270233474624, -33.23888904628638841, -3.760136334089591248 ) ) ;
#47013=CARTESIAN_POINT ( 'NONE',  ( 4.672045878990125800, -33.19353511768168374, 1.847720168420772691 ) ) ;
#47020=B_SPLINE_CURVE_WITH_KNOTS ( 'NONE', 3,
 ( #23800, #16600, #32260, #12748 ),
 .UNSPECIFIED., .F., .F.,
 ( 4, 4 ),
 ( 0.000000000000000000, 0.001246897409371907316 ),
 .UNSPECIFIED. ) ;
#47031=B_SPLINE_CURVE_WITH_KNOTS ( 'NONE', 3,
 ( #37791, #14420, #30085, #29824 ),
 .UNSPECIFIED., .F., .F.,
 ( 4, 4 ),
 ( 4.818759382071585759E-16, 0.009782300387714815831 ),
 .UNSPECIFIED. ) ;
#47032=CARTESIAN_POINT ( 'NONE',  ( -18.67411147745623978, -27.51799019669813973, -3.760136334089591248 ) ) ;
#47042=CARTESIAN_POINT ( 'NONE',  ( 12.97493236725083676, -11.05939663306990717, 8.953103998512858652 ) ) ;
#47049=CARTESIAN_POINT ( 'NONE',  ( -33.86622497129646092, 3.037805405905158462, 7.906207997025717304 ) ) ;
#47064=VECTOR ( 'NONE', #32793, 1000.000000000000000 ) ;
#47074=ADVANCED_FACE ( 'NONE', ( #28011 ), #6474, .T. ) ;
#47078=CARTESIAN_POINT ( 'NONE',  ( 4.641001526964560142, 50.00000000000000711, -8.016098858316199838 ) ) ;
#47080=LINE ( 'NONE', #27639, #24679 ) ;
#47090=CARTESIAN_POINT ( 'NONE',  ( 19.81499429539178436, -31.87968861126187647, -5.338708898921614932 ) ) ;
#47091=ORIENTED_EDGE ( 'NONE', *, *, #4524, .F. ) ;
#47095=CARTESIAN_POINT ( 'NONE',  ( 31.93002621080262671, 9.285431160462559674, -2.408242355805840784 ) ) ;
#47103=ORIENTED_EDGE ( 'NONE', *, *, #16718, .T. ) ;
#47116=ORIENTED_EDGE ( 'NONE', *, *, #4189, .T. ) ;
#47117=CARTESIAN_POINT ( 'NONE',  ( 20.37409433807990666, 26.28007012093483397, -2.408242355805840784 ) ) ;
#47126=CARTESIAN_POINT ( 'NONE',  ( -15.00099850811941948, -7.462898891544107016, 9.403735324607438884 ) ) ;
#47128=CARTESIAN_POINT ( 'NONE',  ( -1.114871695981121125, 0.4953159757245923500, 9.963925895596188909 ) ) ;
#47129=CARTESIAN_POINT ( 'NONE',  ( 8.277096487746778308, -33.14818118907697198, 7.455576670931136185 ) ) ;
#47140=CARTESIAN_POINT ( 'NONE',  ( 9.907356528111447957, -1.358045148324435347, 0.000000000000000000 ) ) ;
#47152=EDGE_CURVE ( 'NONE', #2282, #8731, #17035, .T. ) ;
#47170=CARTESIAN_POINT ( 'NONE',  ( -10.70590866674912967, 12.76446523155714985, -3.546734833711462365 ) ) ;
#47171=CARTESIAN_POINT ( 'NONE',  ( -1.197382828408634081, 0.5140992728904327791, 9.961922210043265835 ) ) ;
#47172=CARTESIAN_POINT ( 'NONE',  ( 50.11058929355269953, -7.578863168071589662, 7.455576670931136185 ) ) ;
#47182=ORIENTED_EDGE ( 'NONE', *, *, #24898, .T. ) ;
#47186=CARTESIAN_POINT ( 'NONE',  ( 0.9300423221600994106, 1.714483250866464914, 9.896382706792429929 ) ) ;
#47188=CARTESIAN_POINT ( 'NONE',  ( 0.000000000000000000, 0.000000000000000000, 0.000000000000000000 ) ) ;
#47194=CARTESIAN_POINT ( 'NONE',  ( 14.29087950072012170, 9.652079258044652832, 8.727788335465566760 ) ) ;
#47202=CARTESIAN_POINT ( 'NONE',  ( -0.8285222815141961572, -1.889008401827320771, 9.886433018048073507 ) ) ;
#47203=CARTESIAN_POINT ( 'NONE',  ( -23.29043492822808759, 24.10797434788186067, 1.847720168420772691 ) ) ;
#47214=VERTEX_POINT ( 'NONE', #29274 ) ;
#47218=DIRECTION ( 'NONE',  ( 0.000000000000000000, 0.000000000000000000, 1.000000000000000000 ) ) ;
#47232=CARTESIAN_POINT ( 'NONE',  ( -0.8283411193296142949, -1.889045124114520080, 9.891980816076525684 ) ) ;
#47239=CARTESIAN_POINT ( 'NONE',  ( -25.40454589245989325, -27.58367357691681931, -8.192531242611266862 ) ) ;
#47240=ORIENTED_EDGE ( 'NONE', *, *, #13644, .F. ) ;
#47249=CARTESIAN_POINT ( 'NONE',  ( -20.72411365307686637, 36.23316402738157649, -8.080361901872242569 ) ) ;
#47250=CARTESIAN_POINT ( 'NONE',  ( -1.249999999999999778, 0.000000000000000000, 10.00000000000000000 ) ) ;
#47258=EDGE_LOOP ( 'NONE', ( #16750, #35529, #36332, #28806 ) ) ;
#47273=VERTEX_POINT ( 'NONE', #38000 ) ;
#47278=B_SPLINE_CURVE_WITH_KNOTS ( 'NONE', 3,
 ( #38857, #50070, #15486, #46742 ),
 .UNSPECIFIED., .F., .F.,
 ( 4, 4 ),
 ( 0.000000000000000000, 0.2545280377015985418 ),
 .UNSPECIFIED. ) ;
#47302=CARTESIAN_POINT ( 'NONE',  ( -1.249999999999999778, 0.000000000000000000, 10.00000000000000000 ) ) ;
#47308=CARTESIAN_POINT ( 'NONE',  ( 25.63461350838963071, -43.17876197216376255, -8.016098858316205167 ) ) ;
#47315=CARTESIAN_POINT ( 'NONE',  ( 2.569099690548740877, -33.19126772784019153, 3.199614146704519602 ) ) ;
#47317=CARTESIAN_POINT ( 'NONE',  ( 8.277096487746778308, -50.00000000000000000, 7.455576670931136185 ) ) ;
#47326=CARTESIAN_POINT ( 'NONE',  ( -2.538055338523173443, -45.80735277814159190, -9.367992836599951190 ) ) ;
#47340=ORIENTED_EDGE ( 'NONE', *, *, #49699, .T. ) ;
#47347=B_SPLINE_SURFACE_WITH_KNOTS ( 'NONE', 3, 3, ( 
 ( #21141, #25496, #33962, #36824 ),
 ( #49301, #25005, #25758, #44721 ),
 ( #32968, #37332, #41402, #6263 ),
 ( #2160, #5493, #45468, #29352 ) ),
 .UNSPECIFIED., .F., .F., .F.,
 ( 4, 4 ),
 ( 4, 4 ),
 ( 0.000000000000000000, 1.000000000000000000 ),
 ( 0.000000000000000000, 1.000000000000000000 ),
 .UNSPECIFIED. ) ;
#47355=VERTEX_POINT ( 'NONE', #14112 ) ;
#47356=CARTESIAN_POINT ( 'NONE',  ( 0.5133303889071102466, -1.273801409042637944, 9.946805383069644790 ) ) ;
#47372=CARTESIAN_POINT ( 'NONE',  ( -1.011271242968683426, -0.7347315653655928092, 10.00000000000000000 ) ) ;
#47374=CARTESIAN_POINT ( 'NONE',  ( -14.29087950072019098, -9.652079258044555132, 8.727788335465566760 ) ) ;
#47377=CARTESIAN_POINT ( 'NONE',  ( 6.875132362119187768, -50.00000000000000711, 8.356839323120299312 ) ) ;
#47380=CARTESIAN_POINT ( 'NONE',  ( 1.553324196727133621, -1.431239106454483379, 9.890170120223999106 ) ) ;
#47390=CARTESIAN_POINT ( 'NONE',  ( -16.76006782980216059, 2.050259795448645228, 9.178419661560148768 ) ) ;
#47403=CARTESIAN_POINT ( 'NONE',  ( 0.6677345994475253343, -1.504830332935386483, 9.927568724237806563 ) ) ;
#47406=EDGE_LOOP ( 'NONE', ( #26533, #89, #352 ) ) ;
#47425=CARTESIAN_POINT ( 'NONE',  ( 7.896046458374581967, -6.155518428822127852, 6.185594734181547594 ) ) ;
#47443=ORIENTED_EDGE ( 'NONE', *, *, #30705, .F. ) ;
#47446=EDGE_CURVE ( 'NONE', #22094, #13764, #15231, .T. ) ;
#47464=EDGE_CURVE ( 'NONE', #30248, #40610, #33589, .T. ) ;
#47472=B_SPLINE_CURVE_WITH_KNOTS ( 'NONE', 3,
 ( #25292, #28632, #12732, #9392 ),
 .UNSPECIFIED., .F., .F.,
 ( 4, 4 ),
 ( 1.734723475976807094E-18, 8.326314924666556211E-06 ),
 .UNSPECIFIED. ) ;
#47480=CARTESIAN_POINT ( 'NONE',  ( 0.8433491450857230065, -0.9182416014173362395, 9.981352469109934233 ) ) ;
#47500=ORIENTED_EDGE ( 'NONE', *, *, #16510, .F. ) ;
#47506=VERTEX_POINT ( 'NONE', #24860 ) ;
#47518=CARTESIAN_POINT ( 'NONE',  ( -15.44803555374685189, -6.237487519713257100, -3.546734833711462365 ) ) ;
#47527=CARTESIAN_POINT ( 'NONE',  ( 25.61277432017878297, -22.36370378792834757, 7.906207997025717304 ) ) ;
#47532=CARTESIAN_POINT ( 'NONE',  ( -44.34968358615014239, -11.74141640735424019, -9.367992836599951190 ) ) ;
#47543=VERTEX_POINT ( 'NONE', #21011 ) ;
#47544=ORIENTED_EDGE ( 'NONE', *, *, #18808, .F. ) ;
#47556=ORIENTED_EDGE ( 'NONE', *, *, #19040, .F. ) ;
#47558=B_SPLINE_CURVE_WITH_KNOTS ( 'NONE', 3,
 ( #28665, #25319, #47616, #12502 ),
 .UNSPECIFIED., .F., .F.,
 ( 4, 4 ),
 ( 0.0009679537044798808103, 0.001281751046851268335 ),
 .UNSPECIFIED. ) ;
#47559=CARTESIAN_POINT ( 'NONE',  ( -16.76006782980216059, 2.050259795448645228, 9.178419661560148768 ) ) ;
#47567=CARTESIAN_POINT ( 'NONE',  ( -31.44259251615275019, -38.95901822126145220, -9.367992836599954742 ) ) ;
#47570=EDGE_CURVE ( 'NONE', #20193, #27159, #28037, .T. ) ;
#47572=B_SPLINE_CURVE_WITH_KNOTS ( 'NONE', 3,
 ( #37319, #1888, #17027, #36303 ),
 .UNSPECIFIED., .F., .F.,
 ( 4, 4 ),
 ( 0.0008678710649527057426, 0.007006382029922212512 ),
 .UNSPECIFIED. ) ;
#47599=FACE_OUTER_BOUND ( 'NONE', #43334, .T. ) ;
#47609=CARTESIAN_POINT ( 'NONE',  ( -1.305659100530649264, 0.2632760600738136558, 9.951893257059998277 ) ) ;
#47616=CARTESIAN_POINT ( 'NONE',  ( 0.3618874479333703542, -1.945951947734774645, 9.897807938190485544 ) ) ;
#47630=EDGE_CURVE ( 'NONE', #20716, #21514, #5939, .T. ) ;
#47634=CARTESIAN_POINT ( 'NONE',  ( 1.962712821592840662, 1.022159834731142691, 9.881002359080275355 ) ) ;
#47642=CARTESIAN_POINT ( 'NONE',  ( -0.8155877869437639927, -0.9072449372115535260, 9.963925895596188909 ) ) ;
#47647=CARTESIAN_POINT ( 'NONE',  ( 28.96803024440893992, 18.11533787072037072, 7.455576670931136185 ) ) ;
#47649=CARTESIAN_POINT ( 'NONE',  ( -0.9989200098981521059, -1.123829893718962802, 9.927319414211225990 ) ) ;
#47667=CARTESIAN_POINT ( 'NONE',  ( -24.87155650802101903, 38.55075836233108788, -9.367992836599951190 ) ) ;
#47669=CARTESIAN_POINT ( 'NONE',  ( -0.3370904143228943828, -0.2449105217885308716, -10.00000000000000000 ) ) ;
#47675=MECHANICAL_DESIGN_GEOMETRIC_PRESENTATION_REPRESENTATION('',(#35443),#37090);
#47680=ORIENTED_EDGE ( 'NONE', *, *, #29595, .F. ) ;
#47683=CARTESIAN_POINT ( 'NONE',  ( -24.47767542868268364, 23.18653802921800278, 8.807470649214879543 ) ) ;
#47691=CARTESIAN_POINT ( 'NONE',  ( 45.21167770612395742, 22.65616271077811206, 7.906207997025717304 ) ) ;
#47693=B_SPLINE_CURVE_WITH_KNOTS ( 'NONE', 3,
 ( #7904, #24313, #31252, #11736 ),
 .UNSPECIFIED., .F., .F.,
 ( 4, 4 ),
 ( 3.066586833366748373E-19, 0.0002708531562719474124 ),
 .UNSPECIFIED. ) ;
#47694=ORIENTED_EDGE ( 'NONE', *, *, #41286, .F. ) ;
#47699=CARTESIAN_POINT ( 'NONE',  ( -0.4400426740873942810, 2.015233077865125733, 9.886433018048068178 ) ) ;
#47712=CARTESIAN_POINT ( 'NONE',  ( 0.000000000000000000, 0.000000000000000000, 10.00000000000000000 ) ) ;
#47719=EDGE_CURVE ( 'NONE', #1381, #45635, #9675, .T. ) ;
#47736=CARTESIAN_POINT ( 'NONE',  ( -0.3656201545664206076, 2.182515578491385000, 9.881002359080270026 ) ) ;
#47741=CARTESIAN_POINT ( 'NONE',  ( 0.2050626648100478400, -1.807624707196173519, 9.903764339332001398 ) ) ;
#47744=CARTESIAN_POINT ( 'NONE',  ( -4.672045878990125800, 33.19353511768168374, 1.847720168420772691 ) ) ;
#47747=ADVANCED_FACE ( 'NONE', ( #3781 ), #11480, .F. ) ;
#47757=B_SPLINE_CURVE_WITH_KNOTS ( 'NONE', 3,
 ( #33559, #26093, #6596, #30196, #48890, #6855 ),
 .UNSPECIFIED., .F., .F.,
 ( 4, 2, 4 ),
 ( 2.453269466693398698E-18, 0.009877169331704828414, 0.01975433866340965683 ),
 .UNSPECIFIED. ) ;
#47759=CARTESIAN_POINT ( 'NONE',  ( -14.86945752723352498, -7.944783388878907004, 2.590526750877053086 ) ) ;
#47768=VERTEX_POINT ( 'NONE', #23012 ) ;
#47769=B_SPLINE_CURVE_WITH_KNOTS ( 'NONE', 3,
 ( #31950, #4980, #32452, #27594 ),
 .UNSPECIFIED., .F., .F.,
 ( 4, 4 ),
 ( 0.002217981418793440844, 0.002368422649471284280 ),
 .UNSPECIFIED. ) ;
#47771=B_SPLINE_SURFACE_WITH_KNOTS ( 'NONE', 3, 3, ( 
 ( #45814, #2248, #29448, #14549 ),
 ( #49660, #6605, #17886, #5850 ),
 ( #10701, #21493, #10207, #33564 ),
 ( #45578, #33317, #30462, #33819 ) ),
 .UNSPECIFIED., .F., .F., .F.,
 ( 4, 4 ),
 ( 4, 4 ),
 ( 0.000000000000000000, 1.000000000000000000 ),
 ( 0.000000000000000000, 1.000000000000000000 ),
 .UNSPECIFIED. ) ;
#47780=CARTESIAN_POINT ( 'NONE',  ( -45.88383801556796016, 6.205508426777106123, 7.455576670931137073 ) ) ;
#47789=CARTESIAN_POINT ( 'NONE',  ( -47.87295225382221275, -14.46560184742400423, -2.408242355805840784 ) ) ;
#47791=CARTESIAN_POINT ( 'NONE',  ( 49.46074318306830975, -9.578883844006833570, 8.807470649214879543 ) ) ;
#47798=CARTESIAN_POINT ( 'NONE',  ( -0.3862712429686729343, -1.188820645368946050, -3.333333333333333481 ) ) ;
#47804=CARTESIAN_POINT ( 'NONE',  ( 14.29087950072012170, 9.652079258044652832, 8.727788335465566760 ) ) ;
#47821=ORIENTED_EDGE ( 'NONE', *, *, #11419, .T. ) ;
#47824=CARTESIAN_POINT ( 'NONE',  ( -1.655785408455817675, -0.7536129375911022610, 9.903764339332079558 ) ) ;
#47833=CARTESIAN_POINT ( 'NONE',  ( -15.80799809827351154, 29.65358618225718956, -8.016098858316199838 ) ) ;
#47835=CARTESIAN_POINT ( 'NONE',  ( -0.1291457462285138802, -10.01396534242280545, 3.215106848023631336 ) ) ;
#47838=CARTESIAN_POINT ( 'NONE',  ( -0.4098590526157695479, -3.751478160727021116, 9.865049507598754985 ) ) ;
#47842=CARTESIAN_POINT ( 'NONE',  ( 18.79997501618727895, 32.48828710620309579, 6.057468652304064172 ) ) ;
#47845=EDGE_CURVE ( 'NONE', #1676, #39341, #32006, .T. ) ;
#47856=CARTESIAN_POINT ( 'NONE',  ( 16.15814872688565984, 4.048305257546810587, -2.870787844569587133 ) ) ;
#47857=EDGE_CURVE ( 'NONE', #13694, #19053, #20672, .T. ) ;
#47859=ADVANCED_FACE ( 'NONE', ( #47599 ), #49449, .T. ) ;
#47865=EDGE_CURVE ( 'NONE', #13851, #16979, #31693, .T. ) ;
#47872=EDGE_LOOP ( 'NONE', ( #48581, #16875, #43805, #44282 ) ) ;
#47879=CARTESIAN_POINT ( 'NONE',  ( -1.841192853132492813, -1.035021892307830482, 9.890170120223997330 ) ) ;
#47889=CARTESIAN_POINT ( 'NONE',  ( -1.019713130072858798, -3.848720492505054658, 6.098637220230962441E-17 ) ) ;
#47891=CARTESIAN_POINT ( 'NONE',  ( 0.3862712429686978033, -1.188820645368937834, -3.333333333333333481 ) ) ;
#47892=EDGE_CURVE ( 'NONE', #20200, #18355, #36113, .T. ) ;
#47897=DIRECTION ( 'NONE',  ( -0.000000000000000000, 0.000000000000000000, -1.000000000000000000 ) ) ;
#47932=ORIENTED_EDGE ( 'NONE', *, *, #33791, .F. ) ;
#47941=CARTESIAN_POINT ( 'NONE',  ( -31.94178169330213279, 9.256608784834037706, -3.760136334089591248 ) ) ;
#47942=CARTESIAN_POINT ( 'NONE',  ( 0.6215990105956902267, -1.608617984725389860, 9.928159647716132241 ) ) ;
#47945=ORIENTED_EDGE ( 'NONE', *, *, #28369, .F. ) ;
#47959=CARTESIAN_POINT ( 'NONE',  ( 8.831420117243668599, 14.12636088103192655, -3.546734833711462365 ) ) ;
#47961=CARTESIAN_POINT ( 'NONE',  ( 21.85563210430597181, 40.58578877481934910, 8.807470649214879543 ) ) ;
#47973=CARTESIAN_POINT ( 'NONE',  ( -9.174209336589896679, -3.979181203266159095, 9.646707543097347681 ) ) ;
#47981=CARTESIAN_POINT ( 'NONE',  ( 1.186340292695366783, -0.3298841998003522735, 9.975326647350891918 ) ) ;
#48002=ORIENTED_EDGE ( 'NONE', *, *, #41882, .F. ) ;
#48015=CARTESIAN_POINT ( 'NONE',  ( -2.462075149652696027, 16.57295996686994499, 9.403735324607438884 ) ) ;
#48020=CARTESIAN_POINT ( 'NONE',  ( 35.51846793572394034, -35.99772139009119343, 7.906207997025717304 ) ) ;
#48021=ORIENTED_EDGE ( 'NONE', *, *, #41819, .F. ) ;
#48028=B_SPLINE_CURVE_WITH_KNOTS ( 'NONE', 3,
 ( #11107, #15213, #26758, #39334 ),
 .UNSPECIFIED., .F., .F.,
 ( 4, 4 ),
 ( 0.7998230999345287140, 0.9869080488566185361 ),
 .UNSPECIFIED. ) ;
#48031=CARTESIAN_POINT ( 'NONE',  ( 1.436574951976903991, -1.361596091069418701, 9.897807938190499755 ) ) ;
#48032=ORIENTED_EDGE ( 'NONE', *, *, #27289, .T. ) ;
#48036=CARTESIAN_POINT ( 'NONE',  ( 23.31729631074197329, 24.19776167542427814, -8.016098858316199838 ) ) ;
#48049=CARTESIAN_POINT ( 'NONE',  ( 1.320835335343329753, -0.01943189459118491516, 9.943883492372847854 ) ) ;
#48057=CARTESIAN_POINT ( 'NONE',  ( -34.38425513258695077, 36.82177522737848108, 8.807470649214879543 ) ) ;
#48060=CARTESIAN_POINT ( 'NONE',  ( -28.52604530808686079, -41.07801380285659576, -3.760136334089591248 ) ) ;
#48064=ADVANCED_FACE ( 'NONE', ( #33512 ), #38477, .T. ) ;
#48075=ORIENTED_EDGE ( 'NONE', *, *, #19907, .F. ) ;
#48080=B_SPLINE_SURFACE_WITH_KNOTS ( 'NONE', 3, 3, ( 
 ( #4355, #19220, #26687, #46402 ),
 ( #3573, #42572, #15899, #7450 ),
 ( #23077, #23593, #19992, #23336 ),
 ( #35677, #14883, #30534, #30797 ) ),
 .UNSPECIFIED., .F., .F., .F.,
 ( 4, 4 ),
 ( 4, 4 ),
 ( 0.000000000000000000, 1.000000000000000000 ),
 ( 0.000000000000000000, 1.000000000000000000 ),
 .UNSPECIFIED. ) ;
#48086=EDGE_CURVE ( 'NONE', #13210, #47506, #516, .T. ) ;
#48087=CARTESIAN_POINT ( 'NONE',  ( 33.08717642956892746, 5.870837526465160217, -8.016098858316199838 ) ) ;
#48089=EDGE_LOOP ( 'NONE', ( #41278, #47544, #18230 ) ) ;
#48095=ORIENTED_EDGE ( 'NONE', *, *, #16718, .F. ) ;
#48096=CARTESIAN_POINT ( 'NONE',  ( -4.641001526964561918, -45.74479092860853058, -8.016098858316205167 ) ) ;
#48102=B_SPLINE_CURVE_WITH_KNOTS ( 'NONE', 3,
 ( #23011, #35106, #24493, #42754 ),
 .UNSPECIFIED., .F., .F.,
 ( 4, 4 ),
 ( 0.003479523240173989628, 0.009617604115990840280 ),
 .UNSPECIFIED. ) ;
#48104=CARTESIAN_POINT ( 'NONE',  ( 1.035950918207909632, 33.23661552194049307, -2.408242355805840784 ) ) ;
#48113=VERTEX_POINT ( 'NONE', #12128 ) ;
#48116=CARTESIAN_POINT ( 'NONE',  ( 1.011271242968688311, -0.7347315653655855927, 10.00000000000000000 ) ) ;
#48130=CARTESIAN_POINT ( 'NONE',  ( -0.3147652639076214398, 1.255102005797271936, 9.947020512645419643 ) ) ;
#48146=CARTESIAN_POINT ( 'NONE',  ( -0.7831114705608903659, -7.934214658316839142, -3.496552006265751800E-15 ) ) ;
#48156=ORIENTED_EDGE ( 'NONE', *, *, #26070, .T. ) ;
#48157=CARTESIAN_POINT ( 'NONE',  ( -1.224655226406675013, -1.100228625579989572, 9.936700280135884356 ) ) ;
#48161=VERTEX_POINT ( 'NONE', #4916 ) ;
#48164=VERTEX_POINT ( 'NONE', #19550 ) ;
#48168=CARTESIAN_POINT ( 'NONE',  ( -13.35436367797847801, -31.26996044524040741, 7.906207997025717304 ) ) ;
#48184=B_SPLINE_SURFACE_WITH_KNOTS ( 'NONE', 3, 3, ( 
 ( #40120, #20098, #44435, #12646 ),
 ( #866, #36283, #47759, #16256 ),
 ( #28556, #27808, #47518, #36026 ),
 ( #40367, #44190, #23953, #1119 ) ),
 .UNSPECIFIED., .F., .F., .F.,
 ( 4, 4 ),
 ( 4, 4 ),
 ( 0.000000000000000000, 1.000000000000000000 ),
 ( 0.000000000000000000, 1.000000000000000000 ),
 .UNSPECIFIED. ) ;
#48185=EDGE_LOOP ( 'NONE', ( #28551, #9065, #32980, #13631 ) ) ;
#48188=CARTESIAN_POINT ( 'NONE',  ( -1.011271242968693862, 0.7347315653655780432, -3.333333333333333481 ) ) ;
#48190=B_SPLINE_CURVE_WITH_KNOTS ( 'NONE', 3,
 ( #16978, #48475, #9522, #20316 ),
 .UNSPECIFIED., .F., .F.,
 ( 4, 4 ),
 ( 0.7491799374948681089, 1.000000000000000000 ),
 .UNSPECIFIED. ) ;
#48194=CARTESIAN_POINT ( 'NONE',  ( -0.8813680857948604785, -1.919528421257472139, 9.884520316594375799 ) ) ;
#48195=B_SPLINE_CURVE_WITH_KNOTS ( 'NONE', 3,
 ( #18538, #49295, #22151, #10093 ),
 .UNSPECIFIED., .F., .F.,
 ( 4, 4 ),
 ( 0.0004299334430849502051, 0.0007706806524480078798 ),
 .UNSPECIFIED. ) ;
#48200=EDGE_CURVE ( 'NONE', #45415, #12448, #43928, .T. ) ;
#48209=ORIENTED_EDGE ( 'NONE', *, *, #29333, .T. ) ;
#48222=CARTESIAN_POINT ( 'NONE',  ( 25.04522487443081502, -22.77512090857307925, 8.356839323120299312 ) ) ;
#48223=ORIENTED_EDGE ( 'NONE', *, *, #48867, .T. ) ;
#48228=VERTEX_POINT ( 'NONE', #36502 ) ;
#48229=CARTESIAN_POINT ( 'NONE',  ( 0.8155877869298099325, 0.9072449372238458043, 9.963925895597341764 ) ) ;
#48230=CARTESIAN_POINT ( 'NONE',  ( 1.150625731496811355, -0.4126014017553309987, 9.969517326150313608 ) ) ;
#48256=CARTESIAN_POINT ( 'NONE',  ( -0.04754753503590647412, 0.8311582663284536876, 9.985686052694765280 ) ) ;
#48264=CARTESIAN_POINT ( 'NONE',  ( -7.576114424932982594, 50.00000000000000711, 7.906207997025717304 ) ) ;
#48265=CARTESIAN_POINT ( 'NONE',  ( 1.401094519807298155, -0.7138523880601698179, 9.927288994922820464 ) ) ;
#48268=CARTESIAN_POINT ( 'NONE',  ( -6.010192544690008631, 37.05120237258827132, 4.835783797351798974 ) ) ;
#48271=EDGE_CURVE ( 'NONE', #36396, #32219, #34143, .T. ) ;
#48288=CARTESIAN_POINT ( 'NONE',  ( 22.69295089195473736, 45.31600496604706052, 7.455576670931136185 ) ) ;
#48290=CARTESIAN_POINT ( 'NONE',  ( -0.3862712429686895876, 1.188820645368940720, -3.333333333333333481 ) ) ;
#48294=CARTESIAN_POINT ( 'NONE',  ( -5.990542248694146643, -8.025558178072376592, 3.215106848023455921 ) ) ;
#48296=EDGE_CURVE ( 'NONE', #11814, #16962, #33497, .T. ) ;
#48302=CARTESIAN_POINT ( 'NONE',  ( 14.52758583651987223, 8.922352469211173087, 8.953103998512858652 ) ) ;
#48305=VERTEX_POINT ( 'NONE', #25692 ) ;
#48322=CARTESIAN_POINT ( 'NONE',  ( 16.52264463346132572, -2.779753662172757878, 9.403735324607438884 ) ) ;
#48327=CARTESIAN_POINT ( 'NONE',  ( -0.2050626648094178439, 1.807624707194796843, 9.903764339332081335 ) ) ;
#48331=EDGE_CURVE ( 'NONE', #17293, #30248, #11495, .T. ) ;
#48343=EDGE_LOOP ( 'NONE', ( #9198, #32378, #3768, #50134 ) ) ;
#48344=CARTESIAN_POINT ( 'NONE',  ( -22.69295089195507487, -45.31600496604688999, 7.455576670931136185 ) ) ;
#48357=CARTESIAN_POINT ( 'NONE',  ( 1.250000000000000222, 0.000000000000000000, -3.333333333333333481 ) ) ;
#48360=VERTEX_POINT ( 'NONE', #11559 ) ;
#48367=CARTESIAN_POINT ( 'NONE',  ( -0.8285222815141961572, -1.889008401827320771, 9.886433018048073507 ) ) ;
#48369=CARTESIAN_POINT ( 'NONE',  ( -15.73090589902298042, -29.60029367929041655, 1.847720168420772691 ) ) ;
#48370=ORIENTED_EDGE ( 'NONE', *, *, #15235, .F. ) ;
#48387=CARTESIAN_POINT ( 'NONE',  ( 8.843309649387377291, -14.11631751497145792, -2.870787844569587133 ) ) ;
#48407=CARTESIAN_POINT ( 'NONE',  ( -10.92344319659207663, -12.63397777816690315, -9.458680755252684591 ) ) ;
#48426=CARTESIAN_POINT ( 'NONE',  ( 1.011271242968683648, 0.7347315653655930312, -10.00000000000000000 ) ) ;
#48427=ORIENTED_EDGE ( 'NONE', *, *, #43976, .F. ) ;
#48438=ORIENTED_EDGE ( 'NONE', *, *, #25288, .F. ) ;
#48443=B_SPLINE_CURVE_WITH_KNOTS ( 'NONE', 3,
 ( #7395, #23021, #20957, #28648 ),
 .UNSPECIFIED., .F., .F.,
 ( 4, 4 ),
 ( 6.459821870315384563E-06, 0.0003472038099299140732 ),
 .UNSPECIFIED. ) ;
#48458=FACE_OUTER_BOUND ( 'NONE', #8151, .T. ) ;
#48459=CARTESIAN_POINT ( 'NONE',  ( -15.98719783915689163, 4.501063718205989161, 3.266473740018926541 ) ) ;
#48460=ORIENTED_EDGE ( 'NONE', *, *, #50402, .T. ) ;
#48468=CARTESIAN_POINT ( 'NONE',  ( 0.1530804384059059886, -1.323112372395012448, 9.951893257060014264 ) ) ;
#48475=CARTESIAN_POINT ( 'NONE',  ( 22.50630130403698459, -35.09254592550291818, -9.387872844313825738 ) ) ;
#48513=CARTESIAN_POINT ( 'NONE',  ( -1.780619886013952602, -1.041246721325602920, 9.886433018048069954 ) ) ;
#48528=CARTESIAN_POINT ( 'NONE',  ( -0.7601424845489993531, 1.297311920617006065, 9.927319414211224213 ) ) ;
#48529=B_SPLINE_CURVE_WITH_KNOTS ( 'NONE', 3,
 ( #30958, #16743, #3470, #1356 ),
 .UNSPECIFIED., .F., .F.,
 ( 4, 4 ),
 ( 5.033378918613206543E-16, 0.009782300387714822770 ),
 .UNSPECIFIED. ) ;
#48534=CARTESIAN_POINT ( 'NONE',  ( 1.962712821592840662, 1.022159834731142691, 9.881002359080275355 ) ) ;
#48540=DIRECTION ( 'NONE',  ( -1.000000000000000000, 0.000000000000000000, -0.000000000000000000 ) ) ;
#48548=CARTESIAN_POINT ( 'NONE',  ( -0.6440276692615867216, -16.64212148744554298, -9.683996418299976483 ) ) ;
#48555=CARTESIAN_POINT ( 'NONE',  ( 1.589327968330908281, 0.05051906867692627923, 9.933337059263775970 ) ) ;
#48561=ORIENTED_EDGE ( 'NONE', *, *, #20893, .F. ) ;
#48568=ORIENTED_EDGE ( 'NONE', *, *, #50528, .F. ) ;
#48571=CARTESIAN_POINT ( 'NONE',  ( 1.540662627795932105, -1.371465786296032441, 9.894754715216729224 ) ) ;
#48573=VERTEX_POINT ( 'NONE', #24130 ) ;
#48581=ORIENTED_EDGE ( 'NONE', *, *, #15235, .T. ) ;
#48585=CARTESIAN_POINT ( 'NONE',  ( 26.64049824243135234, -26.44234984024210178, 4.835783797351800750 ) ) ;
#48592=CARTESIAN_POINT ( 'NONE',  ( 0.7547693905852842500, 1.149888081716854638, 9.972175347158394487 ) ) ;
#48600=CARTESIAN_POINT ( 'NONE',  ( -0.3370904143228927730, -0.2449105217885335917, 10.00000000000000000 ) ) ;
#48605=B_SPLINE_SURFACE_WITH_KNOTS ( 'NONE', 3, 3, ( 
 ( #23310, #16375, #490, #43311 ),
 ( #47377, #25273, #4582, #21167 ),
 ( #44992, #12032, #4330, #9370 ),
 ( #15876, #47129, #8437, #23832 ) ),
 .UNSPECIFIED., .F., .F., .F.,
 ( 4, 4 ),
 ( 4, 4 ),
 ( 0.000000000000000000, 1.000000000000000000 ),
 ( 0.000000000000000000, 1.000000000000000000 ),
 .UNSPECIFIED. ) ;
#48609=ORIENTED_EDGE ( 'NONE', *, *, #11626, .T. ) ;
#48613=EDGE_LOOP ( 'NONE', ( #40895, #27061, #39149, #14436 ) ) ;
#48616=CARTESIAN_POINT ( 'NONE',  ( -0.3862712429686729343, -1.188820645368946050, 10.00000000000000000 ) ) ;
#48625=EDGE_LOOP ( 'NONE', ( #21808, #37274, #31403 ) ) ;
#48626=EDGE_LOOP ( 'NONE', ( #21348, #44794, #7135, #40266 ) ) ;
#48631=CARTESIAN_POINT ( 'NONE',  ( -1.011271242968683426, -0.7347315653655928092, -10.00000000000000000 ) ) ;
#48640=CARTESIAN_POINT ( 'NONE',  ( 0.3862712429686978033, -1.188820645368937834, 3.333333333333333481 ) ) ;
#48641=CARTESIAN_POINT ( 'NONE',  ( -26.18032376592659105, 21.95228666728381128, 7.455576670931136185 ) ) ;
#48651=CARTESIAN_POINT ( 'NONE',  ( -2.920962725444330221, -37.39284056564468983, -9.011255500499645521 ) ) ;
#48653=ORIENTED_EDGE ( 'NONE', *, *, #1354, .T. ) ;
#48654=CARTESIAN_POINT ( 'NONE',  ( 17.23491422248386584, -0.5912720620000816441, 8.727788335465566760 ) ) ;
#48659=CARTESIAN_POINT ( 'NONE',  ( -0.4400426740873942810, 2.015233077865125733, 9.886433018048068178 ) ) ;
#48663=LINE ( 'NONE', #43167, #23825 ) ;
#48689=CARTESIAN_POINT ( 'NONE',  ( 0.6679403265625496466, -1.504705676290996941, 9.936700280135882579 ) ) ;
#48691=CARTESIAN_POINT ( 'NONE',  ( -0.4183366619398694031, 10.00548002840395867, 6.429680520823656487 ) ) ;
#48695=CARTESIAN_POINT ( 'NONE',  ( 48.33712804702525290, 13.03701565032775456, -9.367992836599951190 ) ) ;
#48704=ADVANCED_FACE ( 'NONE', ( #28965 ), #12983, .T. ) ;
#48705=CARTESIAN_POINT ( 'NONE',  ( 0.4402948852767718524, -2.015117899693914527, 9.894754715216725671 ) ) ;
#48706=CARTESIAN_POINT ( 'NONE',  ( -46.11867747200562917, 19.86470446310265103, -8.016098858316199838 ) ) ;
#48719=FACE_OUTER_BOUND ( 'NONE', #37084, .T. ) ;
#48736=CARTESIAN_POINT ( 'NONE',  ( 0.3370904143228947158, 0.2449105217885311492, 10.00000000000000000 ) ) ;
#48738=CARTESIAN_POINT ( 'NONE',  ( -9.174209336589896679, -3.979181203266159095, 9.646707543097347681 ) ) ;
#48745=ORIENTED_EDGE ( 'NONE', *, *, #20548, .F. ) ;
#48746=CARTESIAN_POINT ( 'NONE',  ( -25.40454589245989325, -27.58367357691681931, -8.192531242611266862 ) ) ;
#48748=CARTESIAN_POINT ( 'NONE',  ( -22.69295089195507131, -45.31600496604688999, 7.455576670931136185 ) ) ;
#48756=CARTESIAN_POINT ( 'NONE',  ( 1.578643388466006714, -1.550786058692517511, 9.881002359080275355 ) ) ;
#48762=CARTESIAN_POINT ( 'NONE',  ( 0.3965308786431460675, 0.1288406926356965576, 9.992737339167973687 ) ) ;
#48763=CARTESIAN_POINT ( 'NONE',  ( -0.3862712429686729343, -1.188820645368946050, 3.333333333333333481 ) ) ;
#48767=CARTESIAN_POINT ( 'NONE',  ( -1.249999999999999778, 0.000000000000000000, -10.00000000000000000 ) ) ;
#48776=ADVANCED_FACE ( 'NONE', ( #41525 ), #45774, .T. ) ;
#48800=VECTOR ( 'NONE', #6584, 1000.000000000000000 ) ;
#48802=CARTESIAN_POINT ( 'NONE',  ( 18.38319608353691947, -32.68498281710168385, -8.192531242611265085 ) ) ;
#48805=CARTESIAN_POINT ( 'NONE',  ( -3.940019464150765760, -33.28272320232423453, -8.466730184410787174 ) ) ;
#48811=ORIENTED_EDGE ( 'NONE', *, *, #31504, .F. ) ;
#48816=CARTESIAN_POINT ( 'NONE',  ( 0.7831114743371334619, 7.934214588790045042, -2.805373121306242723E-15 ) ) ;
#48820=CARTESIAN_POINT ( 'NONE',  ( -15.00099850811941948, -7.462898891544107016, 9.403735324607438884 ) ) ;
#48822=ORIENTED_EDGE ( 'NONE', *, *, #38720, .F. ) ;
#48837=CARTESIAN_POINT ( 'NONE',  ( 0.3862712429686727678, 1.188820645368945605, -10.00000000000000000 ) ) ;
#48845=EDGE_CURVE ( 'NONE', #24077, #8523, #37667, .T. ) ;
#48847=CARTESIAN_POINT ( 'NONE',  ( -10.00000000000000000, 0.000000000000000000, 10.00000000000000000 ) ) ;
#48854=CARTESIAN_POINT ( 'NONE',  ( 36.08557433729230723, -35.58569447144768105, 7.455576670931136185 ) ) ;
#48856=ORIENTED_EDGE ( 'NONE', *, *, #19907, .T. ) ;
#48867=EDGE_CURVE ( 'NONE', #23523, #20193, #11748, .T. ) ;
#48871=FACE_OUTER_BOUND ( 'NONE', #25024, .T. ) ;
#48884=CARTESIAN_POINT ( 'NONE',  ( -1.320835335343009787, 0.01943189458965158267, 9.943883492372876276 ) ) ;
#48890=CARTESIAN_POINT ( 'NONE',  ( -34.30563531518998133, -15.23322832906865543, 6.057468652304066836 ) ) ;
#48900=B_SPLINE_CURVE_WITH_KNOTS ( 'NONE', 3,
 ( #10543, #50251, #30308, #38531 ),
 .UNSPECIFIED., .F., .F.,
 ( 4, 4 ),
 ( 7.818293051731877089E-18, 0.0004072981213141015620 ),
 .UNSPECIFIED. ) ;
#48910=ORIENTED_EDGE ( 'NONE', *, *, #9890, .F. ) ;
#48912=B_SPLINE_SURFACE_WITH_KNOTS ( 'NONE', 3, 3, ( 
 ( #16842, #48087, #13230, #43775 ),
 ( #8644, #38371, #9891, #21947 ),
 ( #26054, #13737, #29898, #37622 ),
 ( #2935, #33266, #26309, #49352 ) ),
 .UNSPECIFIED., .F., .F., .F.,
 ( 4, 4 ),
 ( 4, 4 ),
 ( 0.000000000000000000, 1.000000000000000000 ),
 ( 0.000000000000000000, 1.000000000000000000 ),
 .UNSPECIFIED. ) ;
#48919=ORIENTED_EDGE ( 'NONE', *, *, #31182, .T. ) ;
#48927=EDGE_LOOP ( 'NONE', ( #656, #21372, #27840 ) ) ;
#48936=CARTESIAN_POINT ( 'NONE',  ( 0.8282505383454039638, 1.889063466747038289, 9.894754715216722118 ) ) ;
#48937=CARTESIAN_POINT ( 'NONE',  ( 4.641001526964560142, 33.28196331604080171, -8.016098858316199838 ) ) ;
#48939=FACE_OUTER_BOUND ( 'NONE', #14511, .T. ) ;
#48947=CARTESIAN_POINT ( 'NONE',  ( -0.4400426740873942810, 2.015233077865125733, 9.886433018048068178 ) ) ;
#48948=FACE_OUTER_BOUND ( 'NONE', #46625, .T. ) ;
#48950=CARTESIAN_POINT ( 'NONE',  ( 30.64276258327256741, 34.28040101195701794, -8.016098858316205167 ) ) ;
#48952=CARTESIAN_POINT ( 'NONE',  ( 1.011271242968694084, -0.7347315653655782652, 10.00000000000000000 ) ) ;
#48953=CARTESIAN_POINT ( 'NONE',  ( 0.3862712429686894766, -1.188820645368940276, 10.00000000000000000 ) ) ;
#48954=CARTESIAN_POINT ( 'NONE',  ( -1.249999999999999778, 0.000000000000000000, 10.00000000000000000 ) ) ;
#48962=CARTESIAN_POINT ( 'NONE',  ( -8.277096487746778308, 33.14818118907697198, 7.455576670931136185 ) ) ;
#48965=CARTESIAN_POINT ( 'NONE',  ( -8.001683061421429599, -5.997755262142646870, 9.282506307616484875 ) ) ;
#48980=ORIENTED_EDGE ( 'NONE', *, *, #40595, .T. ) ;
#48981=CARTESIAN_POINT ( 'NONE',  ( 0.1287570809895604018, 0.3962735484563146282, 10.00000000000000000 ) ) ;
#48997=CARTESIAN_POINT ( 'NONE',  ( -1.424123654778022274, -0.3625862473323341328, 9.958264684458713489 ) ) ;
#49000=B_SPLINE_CURVE_WITH_KNOTS ( 'NONE', 3,
 ( #15952, #31618, #12337, #24164 ),
 .UNSPECIFIED., .F., .F.,
 ( 4, 4 ),
 ( 0.01012863361515541766, 0.01015667504234211288 ),
 .UNSPECIFIED. ) ;
#49013=FACE_OUTER_BOUND ( 'NONE', #50165, .T. ) ;
#49020=CARTESIAN_POINT ( 'NONE',  ( 0.9983599181300923942, 1.124146016603553733, 9.953784399990620813 ) ) ;
#49022=B_SPLINE_SURFACE_WITH_KNOTS ( 'NONE', 3, 3, ( 
 ( #21053, #33877, #17709, #45125 ),
 ( #2063, #17938, #9254, #33375 ),
 ( #37241, #29006, #5396, #36740 ),
 ( #25162, #25411, #22055, #40807 ) ),
 .UNSPECIFIED., .F., .F., .F.,
 ( 4, 4 ),
 ( 4, 4 ),
 ( 0.000000000000000000, 1.000000000000000000 ),
 ( 0.000000000000000000, 1.000000000000000000 ),
 .UNSPECIFIED. ) ;
#49029=VERTEX_POINT ( 'NONE', #40967 ) ;
#49032=CARTESIAN_POINT ( 'NONE',  ( -1.011271242968677875, -0.7347315653656004697, -10.00000000000000000 ) ) ;
#49036=CARTESIAN_POINT ( 'NONE',  ( -0.1287570809895576818, -0.3962735484563154609, -10.00000000000000000 ) ) ;
#49081=DIRECTION ( 'NONE',  ( 0.000000000000000000, -0.000000000000000000, -1.000000000000000000 ) ) ;
#49093=CARTESIAN_POINT ( 'NONE',  ( 0.6126904405382156416, 1.085824959725723016, 9.981352469109932457 ) ) ;
#49095=LINE ( 'NONE', #25797, #22894 ) ;
#49101=CARTESIAN_POINT ( 'NONE',  ( -31.93002621080269421, -9.285431160462335853, -2.408242355805840784 ) ) ;
#49117=ORIENTED_EDGE ( 'NONE', *, *, #7054, .F. ) ;
#49123=ADVANCED_FACE ( 'NONE', ( #18851 ), #41966, .F. ) ;
#49125=EDGE_CURVE ( 'NONE', #43903, #29160, #46142, .T. ) ;
#49135=CARTESIAN_POINT ( 'NONE',  ( -33.01266944765060174, 5.813986777101691317, 1.847720168420772691 ) ) ;
#49145=CARTESIAN_POINT ( 'NONE',  ( 17.43089236541784359, 28.36237856644539690, 3.199614146704519602 ) ) ;
#49160=B_SPLINE_CURVE_WITH_KNOTS ( 'NONE', 3,
 ( #19183, #10240, #14584, #18427 ),
 .UNSPECIFIED., .F., .F.,
 ( 4, 4 ),
 ( 0.0001535465953326398310, 0.0005837444810855714180 ),
 .UNSPECIFIED. ) ;
#49165=CARTESIAN_POINT ( 'NONE',  ( -0.2131239213568527913, -1.205185050113740219, 9.966990753365125855 ) ) ;
#49172=B_SPLINE_CURVE_WITH_KNOTS ( 'NONE', 3,
 ( #29801, #41600, #8232, #31073 ),
 .UNSPECIFIED., .F., .F.,
 ( 4, 4 ),
 ( 0.0003908573106778929595, 0.0007316046291772774005 ),
 .UNSPECIFIED. ) ;
#49184=ADVANCED_FACE ( 'NONE', ( #35063 ), #5628, .T. ) ;
#49195=B_SPLINE_CURVE_WITH_KNOTS ( 'NONE', 3,
 ( #16435, #7732, #31602, #4132 ),
 .UNSPECIFIED., .F., .F.,
 ( 4, 4 ),
 ( 0.000000000000000000, 0.002466147708923237085 ),
 .UNSPECIFIED. ) ;
#49200=LINE ( 'NONE', #46617, #18856 ) ;
#49205=CARTESIAN_POINT ( 'NONE',  ( -0.9870575514055066613, -1.980598328282574316, 9.881002359080278907 ) ) ;
#49207=CARTESIAN_POINT ( 'NONE',  ( -44.99506233596265048, -23.32283626942287569, 7.455576670931136185 ) ) ;
#49212=CARTESIAN_POINT ( 'NONE',  ( -10.70590866674912967, 12.76446523155714985, -3.546734833711462365 ) ) ;
#49216=CARTESIAN_POINT ( 'NONE',  ( 23.82716369509147825, 44.49195112876006419, 8.356839323120299312 ) ) ;
#49217=CARTESIAN_POINT ( 'NONE',  ( -47.22310614333779455, -16.46562252335923660, -3.760136334089591248 ) ) ;
#49218=CARTESIAN_POINT ( 'NONE',  ( 0.8282505383454039638, 1.889063466747038289, 9.894754715216722118 ) ) ;
#49222=VERTEX_POINT ( 'NONE', #38901 ) ;
#49238=CARTESIAN_POINT ( 'NONE',  ( -36.08557433729204433, 35.58569447144795106, 7.455576670931136185 ) ) ;
#49241=CARTESIAN_POINT ( 'NONE',  ( -49.89397392339119364, 8.245536726717011433, 7.906207997025717304 ) ) ;
#49248=VECTOR ( 'NONE', #15731, 1000.000000000000000 ) ;
#49253=CARTESIAN_POINT ( 'NONE',  ( 0.3862712429686810944, 1.188820645368943607, 10.00000000000000000 ) ) ;
#49262=ADVANCED_FACE ( 'NONE', ( #4490 ), #40869, .T. ) ;
#49271=CARTESIAN_POINT ( 'NONE',  ( 0.1425549192113746144, -1.238581250503543618, 9.981352469109934233 ) ) ;
#49290=VERTEX_POINT ( 'NONE', #24762 ) ;
#49293=ORIENTED_EDGE ( 'NONE', *, *, #30180, .F. ) ;
#49295=CARTESIAN_POINT ( 'NONE',  ( -1.553101183265242602, -0.2460239823947171223, 9.927288994922816912 ) ) ;
#49301=CARTESIAN_POINT ( 'NONE',  ( 46.10908423965007330, 19.89422939639137766, 1.847720168420772691 ) ) ;
#49304=EDGE_CURVE ( 'NONE', #40397, #715, #27844, .T. ) ;
#49311=ORIENTED_EDGE ( 'NONE', *, *, #28761, .F. ) ;
#49327=ORIENTED_EDGE ( 'NONE', *, *, #44797, .T. ) ;
#49336=B_SPLINE_SURFACE_WITH_KNOTS ( 'NONE', 3, 3, ( 
 ( #43252, #35843, #37361, #44248 ),
 ( #21165, #24782, #9869, #13716 ),
 ( #17067, #17818, #25033, #1433 ),
 ( #40429, #1928, #8863, #36851 ) ),
 .UNSPECIFIED., .F., .F., .F.,
 ( 4, 4 ),
 ( 4, 4 ),
 ( 0.000000000000000000, 1.000000000000000000 ),
 ( 0.000000000000000000, 1.000000000000000000 ),
 .UNSPECIFIED. ) ;
#49343=EDGE_CURVE ( 'NONE', #43927, #31351, #41272, .T. ) ;
#49352=CARTESIAN_POINT ( 'NONE',  ( 0.3862712429686978033, -1.188820645368937834, 10.00000000000000000 ) ) ;
#49358=CARTESIAN_POINT ( 'NONE',  ( 37.09740935455766220, -5.526036232978249529, 8.506357886886739550 ) ) ;
#49366=ORIENTED_EDGE ( 'NONE', *, *, #11809, .T. ) ;
#49369=CARTESIAN_POINT ( 'NONE',  ( 2.462075149652696027, -16.57295996686994499, 9.403735324607438884 ) ) ;
#49371=ORIENTED_EDGE ( 'NONE', *, *, #7400, .T. ) ;
#49376=FACE_OUTER_BOUND ( 'NONE', #10850, .T. ) ;
#49379=CARTESIAN_POINT ( 'NONE',  ( 8.277096487746778308, -33.14818118907697198, 7.455576670931136185 ) ) ;
#49382=ORIENTED_EDGE ( 'NONE', *, *, #6688, .T. ) ;
#49383=ORIENTED_EDGE ( 'NONE', *, *, #37617, .F. ) ;
#49389=CARTESIAN_POINT ( 'NONE',  ( -1.424123654778022274, -0.3625862473323341328, 9.958264684458713489 ) ) ;
#49396=VERTEX_POINT ( 'NONE', #21914 ) ;
#49403=CARTESIAN_POINT ( 'NONE',  ( -12.15085308559838317, 11.68662139125813226, 2.590526750877053086 ) ) ;
#49408=ORIENTED_EDGE ( 'NONE', *, *, #18666, .F. ) ;
#49413=EDGE_CURVE ( 'NONE', #37687, #21893, #25382, .T. ) ;
#49438=CARTESIAN_POINT ( 'NONE',  ( 24.47767542868285062, -23.18653802921781448, 8.807470649214879543 ) ) ;
#49449=B_SPLINE_SURFACE_WITH_KNOTS ( 'NONE', 3, 3, ( 
 ( #28147, #12479, #13235, #25299 ),
 ( #43781, #44025, #36367, #48600 ),
 ( #24310, #20949, #28898, #1209 ),
 ( #5543, #39956, #36634, #4780 ) ),
 .UNSPECIFIED., .F., .F., .F.,
 ( 4, 4 ),
 ( 4, 4 ),
 ( 0.000000000000000000, 1.000000000000000000 ),
 ( 0.000000000000000000, 1.000000000000000000 ),
 .UNSPECIFIED. ) ;
#49456=EDGE_LOOP ( 'NONE', ( #46178, #43304, #13953, #24359 ) ) ;
#49457=CARTESIAN_POINT ( 'NONE',  ( 5.320787806771834383, -8.466948512617054945, 0.000000000000000000 ) ) ;
#49459=CARTESIAN_POINT ( 'NONE',  ( 1.011271242968688311, -0.7347315653655855927, 3.333333333333333481 ) ) ;
#49460=ORIENTED_EDGE ( 'NONE', *, *, #46193, .T. ) ;
#49465=EDGE_CURVE ( 'NONE', #49565, #41616, #10017, .T. ) ;
#49472=CARTESIAN_POINT ( 'NONE',  ( 13.92102703536701114, 30.85732372859822803, 8.356839323120299312 ) ) ;
#49478=ORIENTED_EDGE ( 'NONE', *, *, #19699, .T. ) ;
#49482=ORIENTED_EDGE ( 'NONE', *, *, #6114, .T. ) ;
#49508=VECTOR ( 'NONE', #7356, 1000.000000000000000 ) ;
#49510=CARTESIAN_POINT ( 'NONE',  ( -1.782521105131510186, 0.3635605703594341209, 9.903764339332088440 ) ) ;
#49515=CARTESIAN_POINT ( 'NONE',  ( -11.73320209285699889, 11.96063479729179768, 9.403735324607438884 ) ) ;
#49516=CARTESIAN_POINT ( 'NONE',  ( -0.4400426740873942810, 2.015233077865125733, 9.886433018048068178 ) ) ;
#49521=CARTESIAN_POINT ( 'NONE',  ( -7.129058724845069861, -15.30620660340479766, 9.178419661560148768 ) ) ;
#49531=CARTESIAN_POINT ( 'NONE',  ( 0.3862712429686727678, 1.188820645368945605, 10.00000000000000000 ) ) ;
#49540=B_SPLINE_CURVE_WITH_KNOTS ( 'NONE', 3,
 ( #4770, #47835, #12722, #678 ),
 .UNSPECIFIED., .F., .F.,
 ( 4, 4 ),
 ( 9.563268421171419053E-18, 0.009782300387714814097 ),
 .UNSPECIFIED. ) ;
#49550=ORIENTED_EDGE ( 'NONE', *, *, #47857, .T. ) ;
#49565=VERTEX_POINT ( 'NONE', #15722 ) ;
#49566=ORIENTED_EDGE ( 'NONE', *, *, #36402, .T. ) ;
#49573=B_SPLINE_CURVE_WITH_KNOTS ( 'NONE', 3,
 ( #32232, #31738, #47326, #12212 ),
 .UNSPECIFIED., .F., .F.,
 ( 4, 4 ),
 ( 0.7491799374948677759, 1.000000000000000000 ),
 .UNSPECIFIED. ) ;
#49592=CARTESIAN_POINT ( 'NONE',  ( 0.4500758073841586437, 0.7003689023519015233, 9.985686052694765280 ) ) ;
#49601=EDGE_CURVE ( 'NONE', #42210, #14899, #19827, .T. ) ;
#49603=CARTESIAN_POINT ( 'NONE',  ( -16.02661358026017879, -4.530191650547607196, -9.683996418299976483 ) ) ;
#49614=CARTESIAN_POINT ( 'NONE',  ( 1.249999999999999778, 0.000000000000000000, 10.00000000000000000 ) ) ;
#49623=CARTESIAN_POINT ( 'NONE',  ( 31.44259251615245887, 38.95901822126168668, -9.367992836599954742 ) ) ;
#49645=CARTESIAN_POINT ( 'NONE',  ( 2.462075149652696027, -16.57295996686994499, 9.403735324607438884 ) ) ;
#49647=CARTESIAN_POINT ( 'NONE',  ( 10.28825587112223161, -13.03847615613158517, 3.266473740018926541 ) ) ;
#49660=CARTESIAN_POINT ( 'NONE',  ( -45.42829307628559832, -21.98948915213271960, 8.356839323120299312 ) ) ;
#49661=B_SPLINE_CURVE_WITH_KNOTS ( 'NONE', 3,
 ( #31850, #39043, #39548, #39800 ),
 .UNSPECIFIED., .F., .F.,
 ( 4, 4 ),
 ( 0.001403500796105012442, 0.001586656765099013966 ),
 .UNSPECIFIED. ) ;
#49694=CARTESIAN_POINT ( 'NONE',  ( 0.9602803029231544718, -0.8490247040095941777, 9.976582533991681601 ) ) ;
#49698=CARTESIAN_POINT ( 'NONE',  ( -1.249999999999999778, 0.000000000000000000, 9.972675548442463622 ) ) ;
#49699=EDGE_CURVE ( 'NONE', #43553, #44231, #28246, .T. ) ;
#49710=CARTESIAN_POINT ( 'NONE',  ( 10.28825587112223161, -13.03847615613158517, 3.266473740018926541 ) ) ;
#49712=ORIENTED_EDGE ( 'NONE', *, *, #44353, .T. ) ;
#49714=CARTESIAN_POINT ( 'NONE',  ( -36.76598589393961447, -7.383243274241610088, -8.192531242611266862 ) ) ;
#49719=CARTESIAN_POINT ( 'NONE',  ( -1.011271242968688533, 0.7347315653655859258, -3.333333333333333481 ) ) ;
#49721=CARTESIAN_POINT ( 'NONE',  ( 16.16402646813543242, -4.033894069732437693, -3.546734833711462365 ) ) ;
#49734=CARTESIAN_POINT ( 'NONE',  ( -1.228394325311288560, 1.341866297401936636, 9.903764339332077782 ) ) ;
#49739=CARTESIAN_POINT ( 'NONE',  ( -12.97493236725075683, 11.05939663307000664, 8.953103998512858652 ) ) ;
#49740=CARTESIAN_POINT ( 'NONE',  ( 6.408332700304398166, 7.676800896350598258, 0.000000000000000000 ) ) ;
#49741=CARTESIAN_POINT ( 'NONE',  ( -22.50630130403672524, 35.09254592550309582, -9.387872844313825738 ) ) ;
#49744=CARTESIAN_POINT ( 'NONE',  ( 0.3862712429686810944, 1.188820645368943607, 10.00000000000000000 ) ) ;
#49746=ORIENTED_EDGE ( 'NONE', *, *, #30941, .T. ) ;
#49751=LINE ( 'NONE', #38021, #24562 ) ;
#49756=EDGE_CURVE ( 'NONE', #49565, #47768, #44883, .T. ) ;
#49761=ORIENTED_EDGE ( 'NONE', *, *, #15768, .F. ) ;
#49763=CARTESIAN_POINT ( 'NONE',  ( -25.04522487443065160, 22.77512090857326754, 8.356839323120299312 ) ) ;
#49783=ORIENTED_EDGE ( 'NONE', *, *, #21728, .F. ) ;
#49787=CARTESIAN_POINT ( 'NONE',  ( 16.37555114979290849, -29.24217402453064452, -8.466730184410787174 ) ) ;
#49791=ORIENTED_EDGE ( 'NONE', *, *, #50287, .T. ) ;
#49793=LINE ( 'NONE', #17796, #10602 ) ;
#49799=CARTESIAN_POINT ( 'NONE',  ( 17.34922095635755568, 33.24536858281893359, 8.914903342594564961 ) ) ;
#49802=EDGE_LOOP ( 'NONE', ( #32697, #12490, #1483, #50372 ) ) ;
#49820=CARTESIAN_POINT ( 'NONE',  ( -1.024768877994760130, 0.8112356146995477468, 9.945465957785112110 ) ) ;
#49824=CARTESIAN_POINT ( 'NONE',  ( -35.51846793572368455, 35.99772139009146343, 7.906207997025717304 ) ) ;
#49826=CARTESIAN_POINT ( 'NONE',  ( -33.01266944765060174, 5.813986777101691317, 1.847720168420772691 ) ) ;
#49827=CARTESIAN_POINT ( 'NONE',  ( 0.7606162131530698201, -1.296876929034913140, 9.953784399990620813 ) ) ;
#49829=LINE ( 'NONE', #18078, #29965 ) ;
#49833=CARTESIAN_POINT ( 'NONE',  ( -16.76006782980216059, 2.050259795448645228, 9.178419661560148768 ) ) ;
#49843=CARTESIAN_POINT ( 'NONE',  ( 1.011271242968677653, 0.7347315653656002477, -10.00000000000000000 ) ) ;
#49844=CARTESIAN_POINT ( 'NONE',  ( -1.011271242968688533, 0.7347315653655859258, 10.00000000000000000 ) ) ;
#49853=CARTESIAN_POINT ( 'NONE',  ( -25.04522487443065160, 22.77512090857326754, 8.356839323120299312 ) ) ;
#49854=DIRECTION ( 'NONE',  ( -1.000000000000000000, 0.000000000000000000, -0.000000000000000000 ) ) ;
#49869=VERTEX_POINT ( 'NONE', #19179 ) ;
#49876=B_SPLINE_CURVE_WITH_KNOTS ( 'NONE', 3,
 ( #28437, #17131, #2236, #6081, #13521, #9427 ),
 .UNSPECIFIED., .F., .F.,
 ( 4, 2, 4 ),
 ( 4.906538933386796626E-18, 0.009877169331704831884, 0.01975433866340965683 ),
 .UNSPECIFIED. ) ;
#49878=ORIENTED_EDGE ( 'NONE', *, *, #38474, .T. ) ;
#49881=CARTESIAN_POINT ( 'NONE',  ( -0.3618874479330241867, 1.945951947734487320, 9.897807938190496202 ) ) ;
#49895=CARTESIAN_POINT ( 'NONE',  ( 6.875132362119187768, -50.00000000000000711, 8.356839323120299312 ) ) ;
#49916=CARTESIAN_POINT ( 'NONE',  ( -17.43089236541806031, -28.36237856644526900, 3.199614146704519602 ) ) ;
#49925=CARTESIAN_POINT ( 'NONE',  ( -0.4266413953668892756, -1.250184266969579294, 9.943883492372849631 ) ) ;
#49939=VERTEX_POINT ( 'NONE', #468 ) ;
#49941=CARTESIAN_POINT ( 'NONE',  ( -1.962558162477761714, 3.366505435501197407, 9.741991644046970933 ) ) ;
#49944=CARTESIAN_POINT ( 'NONE',  ( 8.831420117243668599, 14.12636088103192655, -3.546734833711462365 ) ) ;
#49956=CARTESIAN_POINT ( 'NONE',  ( 25.63461350838963426, -43.17876197216376966, -8.016098858316199838 ) ) ;
#49959=CARTESIAN_POINT ( 'NONE',  ( -0.7606162131530730397, 1.296876929034918691, 9.953784399990622589 ) ) ;
#49960=VERTEX_POINT ( 'NONE', #28420 ) ;
#49969=CARTESIAN_POINT ( 'NONE',  ( -0.3978397141392179814, -0.1292659590675163117, 9.992713367193013951 ) ) ;
#49975=ORIENTED_EDGE ( 'NONE', *, *, #36629, .F. ) ;
#49976=CARTESIAN_POINT ( 'NONE',  ( -6.875132362119187768, 50.00000000000000711, 8.356839323120299312 ) ) ;
#49977=ORIENTED_EDGE ( 'NONE', *, *, #40595, .F. ) ;
#49984=EDGE_LOOP ( 'NONE', ( #10748, #19165, #48209, #38081 ) ) ;
#49998=CARTESIAN_POINT ( 'NONE',  ( -49.46074318306826001, 9.578883844007169301, 8.807470649214879543 ) ) ;
#50012=CARTESIAN_POINT ( 'NONE',  ( -14.48769039275601145, -30.44468701195584970, 8.807470649214879543 ) ) ;
#50015=CARTESIAN_POINT ( 'NONE',  ( -0.4152287376637092131, 2.070986276654349201, 9.884520316594379352 ) ) ;
#50016=ORIENTED_EDGE ( 'NONE', *, *, #45237, .F. ) ;
#50034=CARTESIAN_POINT ( 'NONE',  ( 12.78770032058947237, 31.68259716188277864, 7.455576670931136185 ) ) ;
#50041=EDGE_CURVE ( 'NONE', #17812, #6007, #35770, .T. ) ;
#50046=CARTESIAN_POINT ( 'NONE',  ( -0.3862712429686977478, 1.188820645368937390, -3.333333333333333481 ) ) ;
#50054=CARTESIAN_POINT ( 'NONE',  ( 16.71930270649943395, 33.57409379679891259, 8.506357886886741326 ) ) ;
#50066=CARTESIAN_POINT ( 'NONE',  ( -0.6440276692615888310, -16.64212148744554298, -9.683996418299976483 ) ) ;
#50070=CARTESIAN_POINT ( 'NONE',  ( -44.94002984196466599, -9.722063056713757589, -8.016098858316205167 ) ) ;
#50073=DIRECTION ( 'NONE',  ( 1.000000000000000000, 0.000000000000000000, 0.000000000000000000 ) ) ;
#50090=CARTESIAN_POINT ( 'NONE',  ( -47.23269937569316568, 16.43609759007082616, -2.408242355805840784 ) ) ;
#50092=CARTESIAN_POINT ( 'NONE',  ( -33.86622497129646092, 3.037805405905158462, 7.906207997025717304 ) ) ;
#50093=ADVANCED_FACE ( 'NONE', ( #1478 ), #5218, .T. ) ;
#50095=CARTESIAN_POINT ( 'NONE',  ( -0.1287570809895632329, 0.3962735484563137400, 10.00000000000000000 ) ) ;
#50098=CARTESIAN_POINT ( 'NONE',  ( 1.337801958641917199, 1.088266084286984015, 9.928159647716135794 ) ) ;
#50099=B_SPLINE_CURVE_WITH_KNOTS ( 'NONE', 3,
 ( #26744, #14939, #46195, #42121 ),
 .UNSPECIFIED., .F., .F.,
 ( 4, 4 ),
 ( 0.0002936521407522628044, 0.0006663369986142421994 ),
 .UNSPECIFIED. ) ;
#50101=EDGE_CURVE ( 'NONE', #8304, #26571, #18543, .T. ) ;
#50103=CARTESIAN_POINT ( 'NONE',  ( 1.011271242968677653, 0.7347315653656002477, 10.00000000000000000 ) ) ;
#50104=CARTESIAN_POINT ( 'NONE',  ( -7.129058724845069861, -15.30620660340479766, 9.178419661560148768 ) ) ;
#50108=B_SPLINE_CURVE_WITH_KNOTS ( 'NONE', 3,
 ( #11846, #27495, #9496, #17210 ),
 .UNSPECIFIED., .F., .F.,
 ( 4, 4 ),
 ( 0.9811748202683399089, 0.9878904167554126703 ),
 .UNSPECIFIED. ) ;
#50110=CARTESIAN_POINT ( 'NONE',  ( -2.462075149652696027, 16.57295996686994499, 9.403735324607438884 ) ) ;
#50113=ORIENTED_EDGE ( 'NONE', *, *, #9952, .F. ) ;
#50114=FACE_OUTER_BOUND ( 'NONE', #41590, .T. ) ;
#50119=ORIENTED_EDGE ( 'NONE', *, *, #26616, .T. ) ;
#50126=CARTESIAN_POINT ( 'NONE',  ( -46.76852358249001895, 17.86468378716740801, -9.367992836599951190 ) ) ;
#50134=ORIENTED_EDGE ( 'NONE', *, *, #2395, .F. ) ;
#50135=EDGE_LOOP ( 'NONE', ( #35940, #3590, #33916, #26149, #35836, #7587, #1238, #41105, #19597, #48919, #44143, #16463 ) ) ;
#50136=B_SPLINE_CURVE_WITH_KNOTS ( 'NONE', 3,
 ( #48659, #25873, #13300, #5354 ),
 .UNSPECIFIED., .F., .F.,
 ( 4, 4 ),
 ( 0.01005345353272278641, 0.01006177981554799705 ),
 .UNSPECIFIED. ) ;
#50147=CARTESIAN_POINT ( 'NONE',  ( -1.780432407520014415, -1.041450996408466612, 9.894754715216725671 ) ) ;
#50155=ORIENTED_EDGE ( 'NONE', *, *, #3633, .F. ) ;
#50163=CARTESIAN_POINT ( 'NONE',  ( 6.619412807845094449, -7.495556955913033725, 9.646707543097347681 ) ) ;
#50164=CARTESIAN_POINT ( 'NONE',  ( -0.2459519479914147599, -1.553112592393893099, 9.927288994922820464 ) ) ;
#50165=EDGE_LOOP ( 'NONE', ( #48438, #10471, #7459 ) ) ;
#50167=B_SPLINE_SURFACE_WITH_KNOTS ( 'NONE', 3, 3, ( 
 ( #22123, #13900, #29567, #45185 ),
 ( #41873, #6230, #49521, #21881 ),
 ( #26228, #18006, #33685, #45437 ),
 ( #6718, #22366, #14154, #29826 ) ),
 .UNSPECIFIED., .F., .F., .F.,
 ( 4, 4 ),
 ( 4, 4 ),
 ( 0.000000000000000000, 1.000000000000000000 ),
 ( 0.000000000000000000, 1.000000000000000000 ),
 .UNSPECIFIED. ) ;
#50172=CARTESIAN_POINT ( 'NONE',  ( -22.69295089195507131, -45.31600496604688999, 7.455576670931136185 ) ) ;
#50175=CARTESIAN_POINT ( 'NONE',  ( 0.4426377647354858835, 1.666766018367784596, 9.928159647716132241 ) ) ;
#50184=CARTESIAN_POINT ( 'NONE',  ( -3.451199890880296994, 1.973209715054570212, 3.247138655587490152 ) ) ;
#50186=VERTEX_POINT ( 'NONE', #26332 ) ;
#50187=ORIENTED_EDGE ( 'NONE', *, *, #24379, .T. ) ;
#50191=CARTESIAN_POINT ( 'NONE',  ( 10.30302290646030627, 13.08520913973580058, -9.683996418299976483 ) ) ;
#50193=B_SPLINE_CURVE_WITH_KNOTS ( 'NONE', 3,
 ( #19012, #14671, #22365, #22874 ),
 .UNSPECIFIED., .F., .F.,
 ( 4, 4 ),
 ( 0.001937412222931638112, 0.003978261222106106373 ),
 .UNSPECIFIED. ) ;
#50197=CARTESIAN_POINT ( 'NONE',  ( -0.4166666666666664631, 0.000000000000000000, 10.00000000000000000 ) ) ;
#50204=CARTESIAN_POINT ( 'NONE',  ( -28.52604530808686079, -41.07801380285659576, -3.760136334089591248 ) ) ;
#50205=VERTEX_POINT ( 'NONE', #41972 ) ;
#50209=CARTESIAN_POINT ( 'NONE',  ( -5.505322767148756569, 37.09368438467003415, 8.914903342594564961 ) ) ;
#50212=CARTESIAN_POINT ( 'NONE',  ( -1.011271242968688533, 0.7347315653655859258, 10.00000000000000000 ) ) ;
#50213=LINE ( 'NONE', #11788, #45001 ) ;
#50249=VERTEX_POINT ( 'NONE', #14777 ) ;
#50251=CARTESIAN_POINT ( 'NONE',  ( 0.3092340281093894361, -2.058543439737950731, 9.888808121373887872 ) ) ;
#50252=ORIENTED_EDGE ( 'NONE', *, *, #41864, .T. ) ;
#50253=CARTESIAN_POINT ( 'NONE',  ( 1.104609456715839766, 0.6504863887005235545, 9.948547179989622791 ) ) ;
#50270=CARTESIAN_POINT ( 'NONE',  ( 1.011271242968677653, 0.7347315653656002477, -3.333333333333333481 ) ) ;
#50271=ORIENTED_EDGE ( 'NONE', *, *, #48296, .T. ) ;
#50279=CARTESIAN_POINT ( 'NONE',  ( 25.60949810002064098, 43.19700938445193827, 1.847720168420772691 ) ) ;
#50283=CARTESIAN_POINT ( 'NONE',  ( -3.566525152643847285, 1.569997364305458776, 9.741991644046965604 ) ) ;
#50284=CARTESIAN_POINT ( 'NONE',  ( -1.343171584780018746, 1.414327272009577641, 9.896382706792429929 ) ) ;
#50287=EDGE_CURVE ( 'NONE', #11996, #40379, #22824, .T. ) ;
#50289=VERTEX_POINT ( 'NONE', #5474 ) ;
#50292=CARTESIAN_POINT ( 'NONE',  ( 22.69295089195473736, 45.31600496604706052, 7.455576670931136185 ) ) ;
#50297=B_SPLINE_CURVE_WITH_KNOTS ( 'NONE', 3,
 ( #34298, #49881, #3754, #7876 ),
 .UNSPECIFIED., .F., .F.,
 ( 4, 4 ),
 ( 6.527761501258140853E-19, 0.0003137973357029442208 ),
 .UNSPECIFIED. ) ;
#50305=ORIENTED_EDGE ( 'NONE', *, *, #40896, .T. ) ;
#50306=ORIENTED_EDGE ( 'NONE', *, *, #44607, .T. ) ;
#50312=CARTESIAN_POINT ( 'NONE',  ( 34.08406891383362591, -15.63733501198463038, -8.192531242611266862 ) ) ;
#50343=CARTESIAN_POINT ( 'NONE',  ( -16.69947034530963847, 2.312583065866374632, 2.590526750877053086 ) ) ;
#50345=CARTESIAN_POINT ( 'NONE',  ( 0.6108107228405675881, -1.056024183042613140, 9.963925895596188909 ) ) ;
#50357=EDGE_LOOP ( 'NONE', ( #7491, #29913, #26935 ) ) ;
#50365=CARTESIAN_POINT ( 'NONE',  ( 0.9599924130074096729, -0.8495346730527926216, 9.948547179989617462 ) ) ;
#50370=CARTESIAN_POINT ( 'NONE',  ( -1.250000000000000222, 0.000000000000000000, 10.00000000000000000 ) ) ;
#50372=ORIENTED_EDGE ( 'NONE', *, *, #27872, .F. ) ;
#50374=CARTESIAN_POINT ( 'NONE',  ( 29.61572577327002520, 16.11461842845735859, 8.807470649214879543 ) ) ;
#50382=PRODUCT_DEFINITION_FORMATION_WITH_SPECIFIED_SOURCE ( 'ANY', '', #10156, .NOT_KNOWN. ) ;
#50390=EDGE_CURVE ( 'NONE', #40728, #12217, #44947, .T. ) ;
#50393=ORIENTED_EDGE ( 'NONE', *, *, #48086, .F. ) ;
#50402=EDGE_CURVE ( 'NONE', #31529, #16294, #29547, .T. ) ;
#50403=CARTESIAN_POINT ( 'NONE',  ( 48.33712804702526000, 13.03701565032775456, -9.367992836599954742 ) ) ;
#50417=CARTESIAN_POINT ( 'NONE',  ( 0.9923808968705242206, -0.8303844723052218324, 9.947020512645417867 ) ) ;
#50420=ORIENTED_EDGE ( 'NONE', *, *, #18887, .T. ) ;
#50421=CARTESIAN_POINT ( 'NONE',  ( 8.277096487746778308, -33.14818118907697198, 7.455576670931136185 ) ) ;
#50425=VERTEX_POINT ( 'NONE', #38983 ) ;
#50437=CARTESIAN_POINT ( 'NONE',  ( -0.3501237319956617688, 1.209643720083639851, 9.974012008644017158 ) ) ;
#50457=CARTESIAN_POINT ( 'NONE',  ( -1.326845121651818227, 0.3624933883365418219, 9.972175347158394487 ) ) ;
#50461=CARTESIAN_POINT ( 'NONE',  ( 44.99506233596246574, 23.32283626942318477, 7.455576670931136185 ) ) ;
#50466=CARTESIAN_POINT ( 'NONE',  ( 9.999999999999998224, 0.04986450829246079353, 8.654293224463657452 ) ) ;
#50471=B_SPLINE_CURVE_WITH_KNOTS ( 'NONE', 3,
 ( #31997, #32244, #20178, #17086 ),
 .UNSPECIFIED., .F., .F.,
 ( 4, 4 ),
 ( 0.001152428489661398931, 0.001623376834729704571 ),
 .UNSPECIFIED. ) ;
#50482=CARTESIAN_POINT ( 'NONE',  ( -45.42829307628559832, -21.98948915213271960, 8.356839323120299312 ) ) ;
#50484=CARTESIAN_POINT ( 'NONE',  ( -0.3862712429686977478, 1.188820645368937390, -3.333333333333333481 ) ) ;
#50487=VERTEX_POINT ( 'NONE', #42800 ) ;
#50493=B_SPLINE_CURVE_WITH_KNOTS ( 'NONE', 3,
 ( #41368, #13895, #41618, #37788 ),
 .UNSPECIFIED., .F., .F.,
 ( 4, 4 ),
 ( 0.000000000000000000, 0.0002610106747148429121 ),
 .UNSPECIFIED. ) ;
#50500=VERTEX_POINT ( 'NONE', #30261 ) ;
#50501=CARTESIAN_POINT ( 'NONE',  ( -27.33593271309441519, 41.94268121623345991, -9.367992836599954742 ) ) ;
#50523=CARTESIAN_POINT ( 'NONE',  ( 0.1287570809895660084, -0.3962735484563127408, 10.00000000000000000 ) ) ;
#50528=EDGE_CURVE ( 'NONE', #30729, #40331, #2550, .T. ) ;
#50542=B_SPLINE_CURVE_WITH_KNOTS ( 'NONE', 3,
 ( #17294, #24757, #40147, #20640 ),
 .UNSPECIFIED., .F., .F.,
 ( 4, 4 ),
 ( 0.9688112071879384501, 0.9724175925769211748 ),
 .UNSPECIFIED. ) ;
#50544=ORIENTED_EDGE ( 'NONE', *, *, #16062, .T. ) ;
#50546=CARTESIAN_POINT ( 'NONE',  ( 23.26005729352310425, 44.90397804740356236, 7.906207997025717304 ) ) ;
#50553=ADVANCED_FACE ( 'NONE', ( #18693 ), #48605, .T. ) ;
#50556=EDGE_CURVE ( 'NONE', #23256, #45635, #30743, .T. ) ;
#50562=UNCERTAINTY_MEASURE_WITH_UNIT (LENGTH_MEASURE( 1.000000000000000082E-05 ), #5960, 'distance_accuracy_value', 'NONE');
#50564=ADVANCED_FACE ( 'NONE', ( #27677, #24092 ), #17573, .T. ) ;
#50565=ORIENTED_EDGE ( 'NONE', *, *, #14634, .T. ) ;
#50566=ORIENTED_EDGE ( 'NONE', *, *, #45961, .T. ) ;
#50568=CARTESIAN_POINT ( 'NONE',  ( 1.588963213309524152E-14, -0.4183134307191408996, 9.992713367193013951 ) ) ;
#50576=ORIENTED_EDGE ( 'NONE', *, *, #21728, .T. ) ;
#50580=CARTESIAN_POINT ( 'NONE',  ( -2.538055338523177440, -50.00000000000000711, -9.367992836599954742 ) ) ;
#50586=ORIENTED_EDGE ( 'NONE', *, *, #13768, .T. ) ;
#50590=CARTESIAN_POINT ( 'NONE',  ( 0.1083376082445593747, 1.382287789010189449, 9.960027343378010656 ) ) ;
#50599=CARTESIAN_POINT ( 'NONE',  ( 12.78770032058947237, 31.68259716188277864, 7.455576670931136185 ) ) ;
#50603=ORIENTED_EDGE ( 'NONE', *, *, #22443, .F. ) ;
#50606=B_SPLINE_SURFACE_WITH_KNOTS ( 'NONE', 3, 3, ( 
 ( #1963, #34031, #49369, #10416 ),
 ( #14000, #10162, #25820, #25311 ),
 ( #6321, #45536, #6818, #26066 ),
 ( #2709, #37140, #40966, #49614 ) ),
 .UNSPECIFIED., .F., .F., .F.,
 ( 4, 4 ),
 ( 4, 4 ),
 ( 0.000000000000000000, 1.000000000000000000 ),
 ( 0.000000000000000000, 1.000000000000000000 ),
 .UNSPECIFIED. ) ;
#50612=CARTESIAN_POINT ( 'NONE',  ( -15.00099850811941948, -7.462898891544107016, 9.403735324607438884 ) ) ;
#50617=EDGE_CURVE ( 'NONE', #17359, #29784, #28914, .T. ) ;
#50619=CARTESIAN_POINT ( 'NONE',  ( 33.16902712922644270, -37.70469005304286725, 1.847720168420772691 ) ) ;
#50632=CARTESIAN_POINT ( 'NONE',  ( 1.250000000000000222, 0.000000000000000000, 10.00000000000000000 ) ) ;
#50638=CARTESIAN_POINT ( 'NONE',  ( -33.43156050989129824, 4.370686678976795747, 8.807470649214879543 ) ) ;
#50641=CARTESIAN_POINT ( 'NONE',  ( 6.174150299305392053, -50.00000000000000711, 8.807470649214879543 ) ) ;
#50643=CARTESIAN_POINT ( 'NONE',  ( 0.9162543521529814550, -1.312131394983855781, 9.919954280166519922 ) ) ;
#50648=CARTESIAN_POINT ( 'NONE',  ( 1.902011274814930042, 1.028513261185797223, 9.882709995651167034 ) ) ;
#50653=CARTESIAN_POINT ( 'NONE',  ( -0.3862712429686977478, 1.188820645368937390, 3.333333333333333481 ) ) ;
#50659=CARTESIAN_POINT ( 'NONE',  ( 5.505322767148756569, -37.09368438467003415, 8.914903342594564961 ) ) ;
#50661=CARTESIAN_POINT ( 'NONE',  ( 1.011271242968677653, 0.7347315653656002477, 10.00000000000000000 ) ) ;
#50662=VERTEX_POINT ( 'NONE', #33745 ) ;
#50671=CARTESIAN_POINT ( 'NONE',  ( 1.142975459103954705, 16.61830776097024653, -2.870787844569587133 ) ) ;
#50672=CARTESIAN_POINT ( 'NONE',  ( 0.000000000000000000, 0.000000000000000000, 0.000000000000000000 ) ) ;
#50688=B_SPLINE_CURVE_WITH_KNOTS ( 'NONE', 3,
 ( #43876, #48689, #44116, #5886 ),
 .UNSPECIFIED., .F., .F.,
 ( 4, 4 ),
 ( 0.9811748202683100439, 0.9878904167554125593 ),
 .UNSPECIFIED. ) ;
#50690=ADVANCED_FACE ( 'NONE', ( #2914 ), #22037, .T. ) ;
#50697=CARTESIAN_POINT ( 'NONE',  ( -36.97942854200451990, 6.226705766838657397, 8.914903342594564961 ) ) ;
#50705=CARTESIAN_POINT ( 'NONE',  ( -34.91952936320829792, 13.67027684621028349, -9.422646554964178023 ) ) ;
#50709=CARTESIAN_POINT ( 'NONE',  ( 12.97493236725083676, -11.05939663306990717, 8.953103998512858652 ) ) ;
#50713=ORIENTED_EDGE ( 'NONE', *, *, #14623, .F. ) ;
#50755=COLOUR_RGB('Sky Blue',0.24,0.69,0.87);
#50756=FILL_AREA_STYLE_COLOUR('',#50755);
#50757=FILL_AREA_STYLE('',(#50756));
#50758=SURFACE_STYLE_FILL_AREA(#50757);
#50759=SURFACE_SIDE_STYLE('',(#50758));
#50760=SURFACE_STYLE_USAGE(.BOTH.,#50759);
#50761=PRESENTATION_STYLE_ASSIGNMENT((#50760));
ENDSEC;
END-ISO-10303-21;
